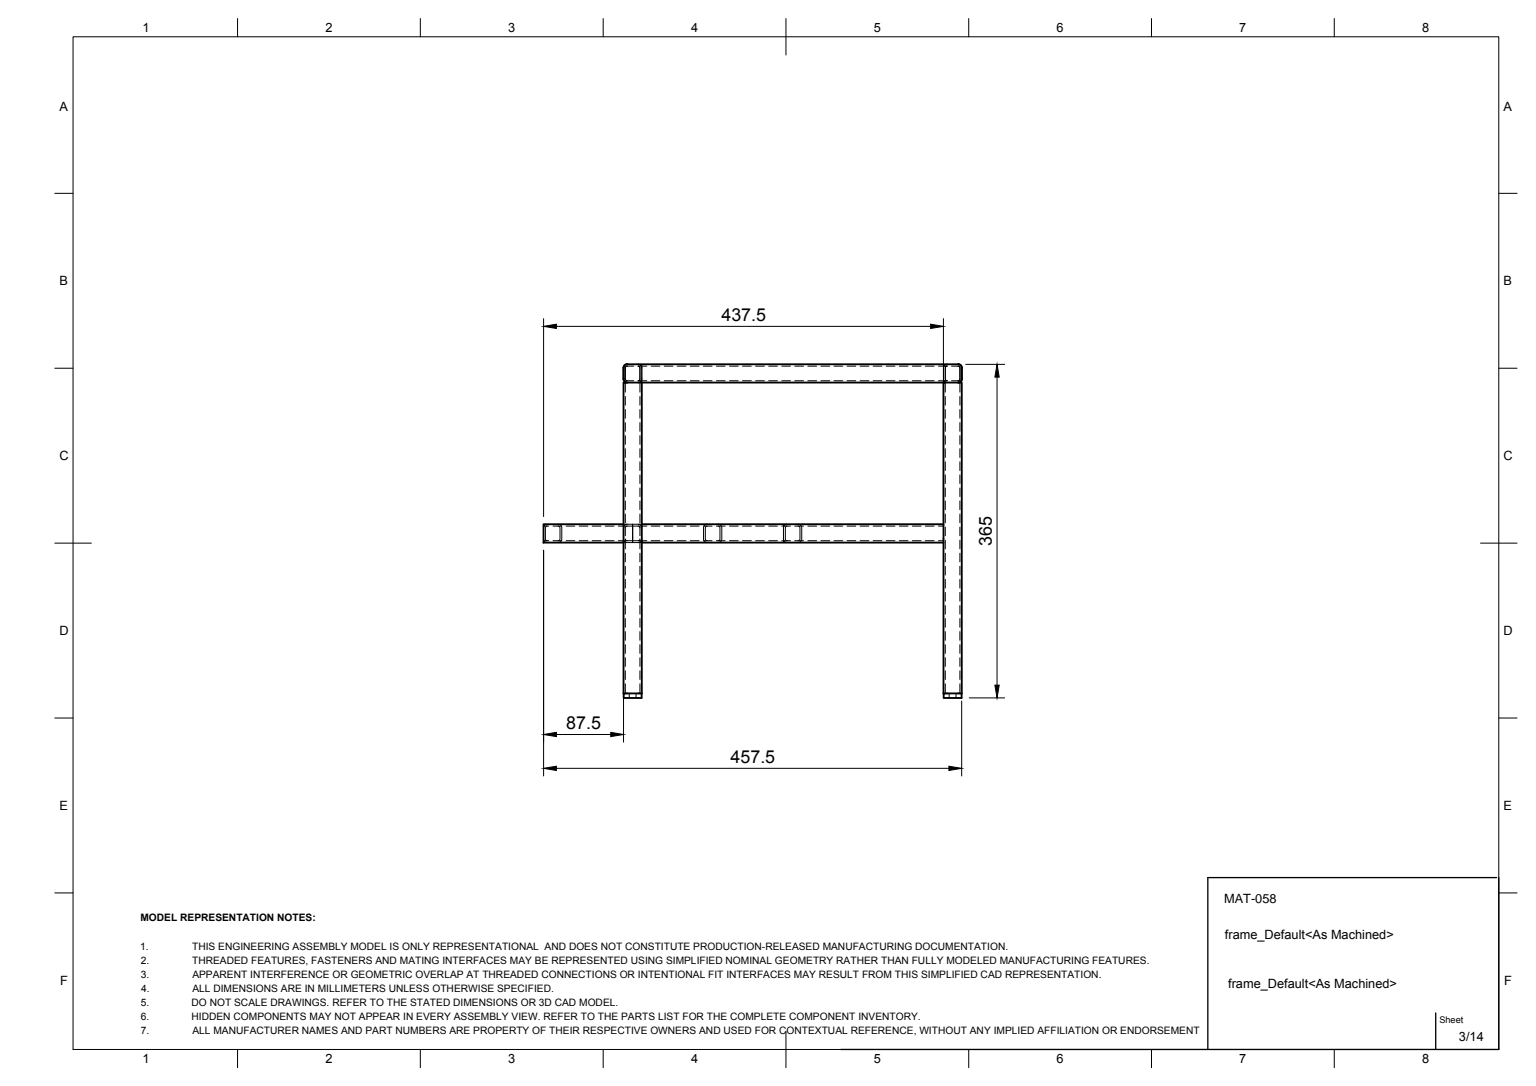
ISO-10303-21;
HEADER;
FILE_DESCRIPTION (('STEP AP214'),
    '1' );
FILE_NAME ('frame_Default<As Machined>.step',
    '2026-10-21T17:54:40',
    ( '' ),
    ( '' ),
    'SwSTEP 2.0',
    'SolidWorks 2026',
    '' );
FILE_SCHEMA (( 'AUTOMOTIVE_DESIGN' ));
ENDSEC;

DATA;
#2=CIRCLE ( 'NONE', #7396, 2.000000000000001776 ) ;
#8=CARTESIAN_POINT ( 'NONE',  ( 341.9999999999999432, -181.0000000000001421, -349.9999999999998863 ) ) ;
#10=ORIENTED_EDGE ( 'NONE', *, *, #50701, .F. ) ;
#13=EDGE_CURVE ( 'NONE', #17667, #14780, #49006, .T. ) ;
#24=AXIS2_PLACEMENT_3D ( 'NONE', #27397, #19697, #35376 ) ;
#26=AXIS2_PLACEMENT_3D ( 'NONE', #26313, #42956, #39141 ) ;
#27=VECTOR ( 'NONE', #2447, 1000.000000000000000 ) ;
#28=EDGE_LOOP ( 'NONE', ( #27721, #41383, #11208, #21958 ) ) ;
#31=ORIENTED_EDGE ( 'NONE', *, *, #39072, .F. ) ;
#35=CARTESIAN_POINT ( 'NONE',  ( 181.0000000000000284, -174.9999999999999716, -111.0000000000001563 ) ) ;
#40=VECTOR ( 'NONE', #48975, 1000.000000000000000 ) ;
#52=( LENGTH_UNIT ( ) NAMED_UNIT ( * ) SI_UNIT ( .MILLI., .METRE. ) );
#53=DIRECTION ( 'NONE',  ( -1.000000000000000000, -0.000000000000000000, -0.000000000000000000 ) ) ;
#55=VERTEX_POINT ( 'NONE', #2115 ) ;
#59=CARTESIAN_POINT ( 'NONE',  ( 164.9999999999999716, -174.9999999999999716, -340.0000000000001137 ) ) ;
#62=AXIS2_PLACEMENT_3D ( 'NONE', #28771, #36489, #21066 ) ;
#68=CARTESIAN_POINT ( 'NONE',  ( 183.0000000000000000, 175.0000000000000284, -356.0000000000001705 ) ) ;
#70=AXIS2_PLACEMENT_3D ( 'NONE', #6927, #30792, #6416 ) ;
#79=DIRECTION ( 'NONE',  ( 0.000000000000000000, -1.000000000000000000, -3.186989995019654210E-49 ) ) ;
#83=ORIENTED_EDGE ( 'NONE', *, *, #42278, .F. ) ;
#87=CARTESIAN_POINT ( 'NONE',  ( 355.9999999999999432, -181.0000000000001421, -349.9999999999999432 ) ) ;
#88=DIRECTION ( 'NONE',  ( 1.121065046350011585E-16, 0.7071067811865475727, 0.7071067811865474617 ) ) ;
#91=ORIENTED_EDGE ( 'NONE', *, *, #48428, .F. ) ;
#96=CIRCLE ( 'NONE', #3362, 4.000000000000003553 ) ;
#98=AXIS2_PLACEMENT_3D ( 'NONE', #41759, #33325, #22512 ) ;
#100=EDGE_LOOP ( 'NONE', ( #22322, #8541, #32792, #19627 ) ) ;
#101=ORIENTED_EDGE ( 'NONE', *, *, #35031, .T. ) ;
#103=FACE_OUTER_BOUND ( 'NONE', #47648, .T. ) ;
#105=ORIENTED_EDGE ( 'NONE', *, *, #23023, .F. ) ;
#111=DIRECTION ( 'NONE',  ( 0.000000000000000000, -2.265761274745217480E-16, 1.000000000000000000 ) ) ;
#114=CARTESIAN_POINT ( 'NONE',  ( 0.000000000000000000, 181.0000000000000284, -356.0000000000002274 ) ) ;
#116=PLANE ( 'NONE',  #46273 ) ;
#117=CARTESIAN_POINT ( 'NONE',  ( 357.1715728752538439, -167.0000000000001137, 342.0000000000000000 ) ) ;
#118=LINE ( 'NONE', #878, #10886 ) ;
#126=CARTESIAN_POINT ( 'NONE',  ( 168.9999999999999716, -272.4999999999999432, -359.9999999999999432 ) ) ;
#127=ORIENTED_EDGE ( 'NONE', *, *, #28456, .T. ) ;
#128=CARTESIAN_POINT ( 'NONE',  ( 355.9999999999999432, 174.9999999999996589, -356.0000000000003411 ) ) ;
#129=CIRCLE ( 'NONE', #5860, 4.000000000000003553 ) ;
#135=EDGE_CURVE ( 'NONE', #16306, #8464, #38459, .T. ) ;
#141=ORIENTED_EDGE ( 'NONE', *, *, #37641, .T. ) ;
#151=ORIENTED_EDGE ( 'NONE', *, *, #46263, .F. ) ;
#152=ORIENTED_EDGE ( 'NONE', *, *, #12710, .F. ) ;
#153=ORIENTED_EDGE ( 'NONE', *, *, #11070, .T. ) ;
#167=EDGE_CURVE ( 'NONE', #5103, #46968, #26727, .T. ) ;
#176=EDGE_CURVE ( 'NONE', #39875, #24207, #43623, .T. ) ;
#177=VECTOR ( 'NONE', #3121, 1000.000000000000000 ) ;
#181=CYLINDRICAL_SURFACE ( 'NONE', #33279, 4.000000000000003553 ) ;
#185=CARTESIAN_POINT ( 'NONE',  ( 359.9999999999999432, -165.0000000000001137, -106.0000000000001990 ) ) ;
#189=EDGE_CURVE ( 'NONE', #37243, #19301, #48193, .T. ) ;
#195=FACE_OUTER_BOUND ( 'NONE', #5721, .T. ) ;
#203=CARTESIAN_POINT ( 'NONE',  ( 349.9999999999999432, -168.9999999999999432, 339.9999999999997726 ) ) ;
#204=ORIENTED_EDGE ( 'NONE', *, *, #887, .F. ) ;
#208=ORIENTED_EDGE ( 'NONE', *, *, #13614, .F. ) ;
#210=CARTESIAN_POINT ( 'NONE',  ( 168.9999999999999716, 165.0000000000000000, -360.0000000000002274 ) ) ;
#211=DIRECTION ( 'NONE',  ( -1.000000000000000000, 0.000000000000000000, 1.860490536778032451E-50 ) ) ;
#212=ADVANCED_FACE ( 'NONE', ( #47688 ), #43368, .T. ) ;
#215=DIRECTION ( 'NONE',  ( 0.000000000000000000, 3.186989995019654210E-49, 1.000000000000000000 ) ) ;
#216=DIRECTION ( 'NONE',  ( 3.172065784643302499E-16, 1.000000000000000000, 0.000000000000000000 ) ) ;
#218=VERTEX_POINT ( 'NONE', #20031 ) ;
#220=CARTESIAN_POINT ( 'NONE',  ( 168.9999999999999716, 10.00000000000006395, 339.9999999999998295 ) ) ;
#223=EDGE_LOOP ( 'NONE', ( #625, #40155, #13058, #17108 ) ) ;
#236=DIRECTION ( 'NONE',  ( -0.000000000000000000, -1.000000000000000000, 2.537652627714643577E-15 ) ) ;
#250=AXIS2_PLACEMENT_3D ( 'NONE', #2774, #2274, #17912 ) ;
#254=DIRECTION ( 'NONE',  ( 0.000000000000000000, -1.000000000000000000, 0.000000000000000000 ) ) ;
#260=ORIENTED_EDGE ( 'NONE', *, *, #20042, .T. ) ;
#262=ORIENTED_EDGE ( 'NONE', *, *, #31509, .T. ) ;
#269=VERTEX_POINT ( 'NONE', #28497 ) ;
#274=ORIENTED_EDGE ( 'NONE', *, *, #2719, .F. ) ;
#276=CARTESIAN_POINT ( 'NONE',  ( 358.0000000000000000, -165.0000000000001137, -94.00000000000019895 ) ) ;
#278=DIRECTION ( 'NONE',  ( 0.000000000000000000, 5.664403186863042467E-17, 1.000000000000000000 ) ) ;
#280=DIRECTION ( 'NONE',  ( 3.172065784643304472E-16, 1.000000000000000000, -1.710569414459005214E-49 ) ) ;
#281=EDGE_CURVE ( 'NONE', #25566, #31089, #9489, .T. ) ;
#286=EDGE_LOOP ( 'NONE', ( #4759, #15600, #2107, #33444, #6619, #35466, #25872, #11433 ) ) ;
#291=CARTESIAN_POINT ( 'NONE',  ( 356.0000000000000000, -167.0000000000001137, -349.9999999999999432 ) ) ;
#292=FACE_OUTER_BOUND ( 'NONE', #17808, .T. ) ;
#296=EDGE_CURVE ( 'NONE', #47828, #22723, #5634, .T. ) ;
#301=DIRECTION ( 'NONE',  ( 0.000000000000000000, 0.000000000000000000, -1.000000000000000000 ) ) ;
#303=ORIENTED_EDGE ( 'NONE', *, *, #21142, .F. ) ;
#304=EDGE_CURVE ( 'NONE', #27971, #25755, #44964, .T. ) ;
#310=CIRCLE ( 'NONE', #31701, 4.000000000000003553 ) ;
#315=CARTESIAN_POINT ( 'NONE',  ( 339.9999999999998863, -183.3431457505075741, 358.3431457505074036 ) ) ;
#318=PLANE ( 'NONE',  #3677 ) ;
#324=CARTESIAN_POINT ( 'NONE',  ( 340.0000000000000000, 181.0000000000000568, 359.9999999999998295 ) ) ;
#328=CARTESIAN_POINT ( 'NONE',  ( 340.0000000000000568, 185.0000000000000284, 355.9999999999997726 ) ) ;
#330=ORIENTED_EDGE ( 'NONE', *, *, #46512, .T. ) ;
#333=CARTESIAN_POINT ( 'NONE',  ( 355.9999999999999432, 185.0000000000002274, -360.0000000000003411 ) ) ;
#336=LINE ( 'NONE', #31644, #47492 ) ;
#340=ORIENTED_EDGE ( 'NONE', *, *, #875, .T. ) ;
#345=DIRECTION ( 'NONE',  ( -1.000000000000000000, 0.000000000000000000, 0.000000000000000000 ) ) ;
#347=VECTOR ( 'NONE', #5302, 1000.000000000000000 ) ;
#351=AXIS2_PLACEMENT_3D ( 'NONE', #22254, #34073, #6858 ) ;
#353=DIRECTION ( 'NONE',  ( 0.000000000000000000, 0.000000000000000000, 1.000000000000000000 ) ) ;
#354=VECTOR ( 'NONE', #29219, 1000.000000000000000 ) ;
#355=DIRECTION ( 'NONE',  ( 3.172065745548403743E-16, 1.000000000000000000, 0.000000000000000000 ) ) ;
#359=EDGE_LOOP ( 'NONE', ( #2759, #29859, #45477, #2453, #26930, #35930, #303, #44900 ) ) ;
#363=ORIENTED_EDGE ( 'NONE', *, *, #44882, .T. ) ;
#370=CARTESIAN_POINT ( 'NONE',  ( 356.0000000000000000, 175.0000000000000284, -108.0000000000002132 ) ) ;
#372=CARTESIAN_POINT ( 'NONE',  ( 185.0000000000000000, -93.49999999999998579, -350.0000000000001705 ) ) ;
#373=LINE ( 'NONE', #27571, #20702 ) ;
#376=EDGE_CURVE ( 'NONE', #35109, #22226, #31907, .T. ) ;
#380=CARTESIAN_POINT ( 'NONE',  ( 0.000000000000000000, -165.1999999999999602, 340.1999999999997044 ) ) ;
#390=DIRECTION ( 'NONE',  ( 0.000000000000000000, -2.265761274745217480E-16, 1.000000000000000000 ) ) ;
#399=CARTESIAN_POINT ( 'NONE',  ( 343.9999999999999432, 174.9999999999996589, -360.0000000000003411 ) ) ;
#401=CYLINDRICAL_SURFACE ( 'NONE', #39045, 4.000000000000003553 ) ;
#402=DIRECTION ( 'NONE',  ( 1.000000000000000000, -4.105366553918459587E-48, -1.586032880504786307E-16 ) ) ;
#416=CARTESIAN_POINT ( 'NONE',  ( 344.0000000000000000, 165.0000000000000000, -90.00000000000018474 ) ) ;
#417=ORIENTED_EDGE ( 'NONE', *, *, #25940, .F. ) ;
#424=LINE ( 'NONE', #28123, #46558 ) ;
#427=EDGE_CURVE ( 'NONE', #32721, #15345, #25659, .T. ) ;
#428=PLANE ( 'NONE',  #26708 ) ;
#432=DIRECTION ( 'NONE',  ( -1.000000000000000000, 1.331116318405244905E-23, 4.755310728521421461E-16 ) ) ;
#433=ADVANCED_FACE ( 'NONE', ( #33614 ), #49204, .F. ) ;
#435=APPLICATION_CONTEXT ( 'automotive_design' ) ;
#439=DIRECTION ( 'NONE',  ( -1.586032892321652236E-16, -1.000000000000000000, -6.853681917100419162E-49 ) ) ;
#441=ORIENTED_EDGE ( 'NONE', *, *, #33733, .F. ) ;
#445=CIRCLE ( 'NONE', #40629, 2.000000000000001776 ) ;
#462=LINE ( 'NONE', #35873, #24910 ) ;
#471=ORIENTED_EDGE ( 'NONE', *, *, #17428, .F. ) ;
#473=CARTESIAN_POINT ( 'NONE',  ( 355.9999999999999432, -185.0000000000001421, 360.0000000000000000 ) ) ;
#474=ORIENTED_EDGE ( 'NONE', *, *, #34538, .F. ) ;
#476=ORIENTED_EDGE ( 'NONE', *, *, #29069, .T. ) ;
#479=AXIS2_PLACEMENT_3D ( 'NONE', #48205, #1053, #44377 ) ;
#481=ORIENTED_EDGE ( 'NONE', *, *, #5333, .T. ) ;
#489=EDGE_CURVE ( 'NONE', #13008, #49667, #30971, .T. ) ;
#492=DIRECTION ( 'NONE',  ( 1.000000000000000000, 0.000000000000000000, 0.000000000000000000 ) ) ;
#495=DIRECTION ( 'NONE',  ( 0.000000000000000000, 2.537652627714642000E-15, 1.000000000000000000 ) ) ;
#497=AXIS2_PLACEMENT_3D ( 'NONE', #34833, #26856, #31230 ) ;
#498=EDGE_CURVE ( 'NONE', #19922, #10844, #20629, .T. ) ;
#500=PLANE ( 'NONE',  #17515 ) ;
#501=CARTESIAN_POINT ( 'NONE',  ( 359.9999999999999432, -181.0000000000001137, -356.0000000000003411 ) ) ;
#504=CARTESIAN_POINT ( 'NONE',  ( 343.9999999999999432, 165.0000000000000000, -108.0000000000002132 ) ) ;
#505=ORIENTED_EDGE ( 'NONE', *, *, #34410, .F. ) ;
#513=LINE ( 'NONE', #24116, #49110 ) ;
#514=EDGE_CURVE ( 'NONE', #45973, #15209, #36212, .T. ) ;
#524=CIRCLE ( 'NONE', #29193, 2.000000000000001776 ) ;
#537=CARTESIAN_POINT ( 'NONE',  ( 168.9999999999999716, 10.00000000000006395, -350.0000000000001705 ) ) ;
#541=VERTEX_POINT ( 'NONE', #28876 ) ;
#545=DIRECTION ( 'NONE',  ( 0.000000000000000000, 0.000000000000000000, -1.000000000000000000 ) ) ;
#551=DIRECTION ( 'NONE',  ( 1.000000000000000000, -4.758098676964956461E-16, -8.975803739141899931E-48 ) ) ;
#557=CARTESIAN_POINT ( 'NONE',  ( 181.0000000000000000, -182.9999999999999716, -350.0000000000001705 ) ) ;
#558=PLANE ( 'NONE',  #37929 ) ;
#564=CARTESIAN_POINT ( 'NONE',  ( 339.9999999999999432, -168.9999999999999432, 343.9999999999998295 ) ) ;
#584=VECTOR ( 'NONE', #25385, 1000.000000000000000 ) ;
#586=VERTEX_POINT ( 'NONE', #1185 ) ;
#590=DIRECTION ( 'NONE',  ( 0.000000000000000000, 0.000000000000000000, -1.000000000000000000 ) ) ;
#605=FACE_OUTER_BOUND ( 'NONE', #3161, .T. ) ;
#606=DIRECTION ( 'NONE',  ( 3.172065745548403743E-16, 1.000000000000000000, 0.000000000000000000 ) ) ;
#607=ORIENTED_EDGE ( 'NONE', *, *, #46352, .F. ) ;
#618=ORIENTED_EDGE ( 'NONE', *, *, #16431, .T. ) ;
#619=CARTESIAN_POINT ( 'NONE',  ( 350.0000000000000000, -164.9999999999999432, -344.0000000000001705 ) ) ;
#621=DIRECTION ( 'NONE',  ( 0.000000000000000000, 0.000000000000000000, -1.000000000000000000 ) ) ;
#625=ORIENTED_EDGE ( 'NONE', *, *, #32485, .F. ) ;
#626=ORIENTED_EDGE ( 'NONE', *, *, #37900, .T. ) ;
#627=DIRECTION ( 'NONE',  ( -0.000000000000000000, 0.000000000000000000, 1.000000000000000000 ) ) ;
#631=DIRECTION ( 'NONE',  ( 0.000000000000000000, -1.000000000000000000, 5.664403186863042467E-17 ) ) ;
#637=DIRECTION ( 'NONE',  ( 0.000000000000000000, 2.537652627714642000E-15, 1.000000000000000000 ) ) ;
#640=ORIENTED_EDGE ( 'NONE', *, *, #27418, .F. ) ;
#644=ORIENTED_EDGE ( 'NONE', *, *, #10302, .T. ) ;
#647=DIRECTION ( 'NONE',  ( 1.000000000000000000, 0.000000000000000000, 0.000000000000000000 ) ) ;
#660=LINE ( 'NONE', #35837, #18061 ) ;
#664=ORIENTED_EDGE ( 'NONE', *, *, #22451, .F. ) ;
#665=ORIENTED_EDGE ( 'NONE', *, *, #13294, .F. ) ;
#673=EDGE_LOOP ( 'NONE', ( #3363, #25492, #26505, #29647 ) ) ;
#677=EDGE_CURVE ( 'NONE', #7451, #29467, #310, .T. ) ;
#695=EDGE_LOOP ( 'NONE', ( #33411, #25754, #20493, #618 ) ) ;
#697=DIRECTION ( 'NONE',  ( -1.000000000000000000, 0.000000000000000000, 0.000000000000000000 ) ) ;
#701=LINE ( 'NONE', #27656, #40511 ) ;
#710=ORIENTED_EDGE ( 'NONE', *, *, #4911, .F. ) ;
#711=AXIS2_PLACEMENT_3D ( 'NONE', #49529, #33197, #17779 ) ;
#716=ORIENTED_EDGE ( 'NONE', *, *, #36986, .T. ) ;
#722=CLOSED_SHELL ( 'NONE', ( #33273, #13699, #32863, #47477, #42616, #48990, #26917, #42906, #40350, #7482, #18343, #10767, #37802, #12006, #35923, #10315, #35706, #47951 ) ) ;
#723=EDGE_CURVE ( 'NONE', #541, #5037, #49825, .T. ) ;
#724=DIRECTION ( 'NONE',  ( 0.000000000000000000, 1.000000000000000000, 0.000000000000000000 ) ) ;
#727=DIRECTION ( 'NONE',  ( 0.000000000000000000, 0.000000000000000000, 1.000000000000000000 ) ) ;
#728=PLANE ( 'NONE',  #43991 ) ;
#737=EDGE_CURVE ( 'NONE', #25893, #7888, #18657, .T. ) ;
#742=DIRECTION ( 'NONE',  ( 1.000000000000000000, 0.000000000000000000, 0.000000000000000000 ) ) ;
#750=VERTEX_POINT ( 'NONE', #17821 ) ;
#753=VECTOR ( 'NONE', #3880, 1000.000000000000000 ) ;
#754=ORIENTED_EDGE ( 'NONE', *, *, #25734, .F. ) ;
#761=CARTESIAN_POINT ( 'NONE',  ( 344.0000000000000568, -165.0000000000001137, 340.0000000000000568 ) ) ;
#767=EDGE_CURVE ( 'NONE', #14253, #48821, #16231, .T. ) ;
#770=DIRECTION ( 'NONE',  ( 0.000000000000000000, 0.000000000000000000, -1.000000000000000000 ) ) ;
#771=ORIENTED_EDGE ( 'NONE', *, *, #33152, .T. ) ;
#773=CARTESIAN_POINT ( 'NONE',  ( 350.0000000000000000, -164.9999999999999432, 339.9999999999997726 ) ) ;
#775=CARTESIAN_POINT ( 'NONE',  ( 181.0000000000000000, -93.49999999999998579, -350.0000000000001705 ) ) ;
#779=PLANE ( 'NONE',  #43621 ) ;
#780=ORIENTED_EDGE ( 'NONE', *, *, #22663, .T. ) ;
#782=ORIENTED_EDGE ( 'NONE', *, *, #44110, .F. ) ;
#786=DIRECTION ( 'NONE',  ( 4.996003610813203446E-16, 1.000000000000000000, 0.000000000000000000 ) ) ;
#790=FACE_OUTER_BOUND ( 'NONE', #30397, .T. ) ;
#792=EDGE_LOOP ( 'NONE', ( #16265, #22967, #43892, #43654, #12939, #41162, #11499, #30707 ) ) ;
#795=DIRECTION ( 'NONE',  ( -1.586032892321652236E-16, -1.000000000000000000, -6.853681917100419162E-49 ) ) ;
#804=VECTOR ( 'NONE', #10594, 1000.000000000000000 ) ;
#805=FACE_OUTER_BOUND ( 'NONE', #27242, .T. ) ;
#808=EDGE_CURVE ( 'NONE', #7132, #20673, #30143, .T. ) ;
#812=ORIENTED_EDGE ( 'NONE', *, *, #6128, .T. ) ;
#813=EDGE_CURVE ( 'NONE', #46472, #47613, #15528, .T. ) ;
#816=CARTESIAN_POINT ( 'NONE',  ( 340.0000000000000000, 165.0000000000000000, -94.00000000000019895 ) ) ;
#825=DIRECTION ( 'NONE',  ( 0.000000000000000000, 3.186989995019654210E-49, 1.000000000000000000 ) ) ;
#827=DIRECTION ( 'NONE',  ( 1.000000000000000000, -4.996003610813203446E-16, 1.033975765691284410E-24 ) ) ;
#828=AXIS2_PLACEMENT_3D ( 'NONE', #16656, #16407, #1278 ) ;
#831=VECTOR ( 'NONE', #20626, 1000.000000000000000 ) ;
#843=ORIENTED_EDGE ( 'NONE', *, *, #48550, .T. ) ;
#846=ORIENTED_EDGE ( 'NONE', *, *, #17978, .T. ) ;
#847=DIRECTION ( 'NONE',  ( 0.000000000000000000, 0.000000000000000000, -1.000000000000000000 ) ) ;
#849=CARTESIAN_POINT ( 'NONE',  ( 181.0000000000000000, 165.0000000000000000, -356.0000000000001705 ) ) ;
#850=ORIENTED_EDGE ( 'NONE', *, *, #26302, .T. ) ;
#853=CARTESIAN_POINT ( 'NONE',  ( 341.9999999999999432, -174.9999999999999432, 343.9999999999998295 ) ) ;
#859=ORIENTED_EDGE ( 'NONE', *, *, #37775, .T. ) ;
#870=CARTESIAN_POINT ( 'NONE',  ( 360.0000000000000000, 169.0000000000000000, -344.0000000000001705 ) ) ;
#873=EDGE_CURVE ( 'NONE', #23733, #17617, #46498, .T. ) ;
#874=AXIS2_PLACEMENT_3D ( 'NONE', #50548, #11862, #46963 ) ;
#875=EDGE_CURVE ( 'NONE', #3991, #24185, #15745, .T. ) ;
#878=CARTESIAN_POINT ( 'NONE',  ( 350.0000000000001137, 165.0000000000000000, 339.9999999999997726 ) ) ;
#879=ORIENTED_EDGE ( 'NONE', *, *, #10874, .F. ) ;
#881=VECTOR ( 'NONE', #25390, 1000.000000000000000 ) ;
#887=EDGE_CURVE ( 'NONE', #25778, #16503, #8068, .T. ) ;
#888=ADVANCED_FACE ( 'NONE', ( #35027, #43446 ), #35271, .F. ) ;
#890=CARTESIAN_POINT ( 'NONE',  ( 356.0000000000000000, 175.0000000000000284, -106.0000000000001990 ) ) ;
#891=VERTEX_POINT ( 'NONE', #8318 ) ;
#899=DIRECTION ( 'NONE',  ( -1.000000000000000000, 0.000000000000000000, -2.958228394578794270E-31 ) ) ;
#901=EDGE_LOOP ( 'NONE', ( #812, #8607, #36597, #25658, #49808, #20531, #25126, #10877 ) ) ;
#905=AXIS2_PLACEMENT_3D ( 'NONE', #21960, #14251, #29911 ) ;
#912=CARTESIAN_POINT ( 'NONE',  ( 358.0000000000000000, 181.0000000000000284, -356.0000000000001705 ) ) ;
#913=VERTEX_POINT ( 'NONE', #3428 ) ;
#917=ADVANCED_FACE ( 'NONE', ( #47265 ), #4455, .F. ) ;
#921=VERTEX_POINT ( 'NONE', #15493 ) ;
#922=CARTESIAN_POINT ( 'NONE',  ( 166.9999999999999716, -81.49999999999997158, -350.0000000000001705 ) ) ;
#933=EDGE_CURVE ( 'NONE', #12765, #28712, #42680, .T. ) ;
#943=EDGE_CURVE ( 'NONE', #29362, #4473, #21108, .T. ) ;
#945=LINE ( 'NONE', #44015, #12242 ) ;
#946=VECTOR ( 'NONE', #12223, 1000.000000000000000 ) ;
#948=CIRCLE ( 'NONE', #42702, 4.000000000000003553 ) ;
#951=( LENGTH_UNIT ( ) NAMED_UNIT ( * ) SI_UNIT ( .MILLI., .METRE. ) );
#958=FACE_OUTER_BOUND ( 'NONE', #48495, .T. ) ;
#964=DIRECTION ( 'NONE',  ( -1.586032880504786307E-16, 1.654361225106055350E-24, -1.000000000000000000 ) ) ;
#974=ORIENTED_EDGE ( 'NONE', *, *, #47561, .T. ) ;
#976=VECTOR ( 'NONE', #24664, 1000.000000000000000 ) ;
#980=VERTEX_POINT ( 'NONE', #870 ) ;
#994=FACE_BOUND ( 'NONE', #1999, .T. ) ;
#996=UNCERTAINTY_MEASURE_WITH_UNIT (LENGTH_MEASURE( 1.000000000000000082E-05 ), #25917, 'distance_accuracy_value', 'NONE');
#1002=AXIS2_PLACEMENT_3D ( 'NONE', #43365, #551, #47189 ) ;
#1006=AXIS2_PLACEMENT_3D ( 'NONE', #10575, #7241, #26244 ) ;
#1007=ORIENTED_EDGE ( 'NONE', *, *, #6239, .F. ) ;
#1009=AXIS2_PLACEMENT_3D ( 'NONE', #24502, #44226, #9104 ) ;
#1011=ORIENTED_EDGE ( 'NONE', *, *, #33096, .F. ) ;
#1013=CARTESIAN_POINT ( 'NONE',  ( 169.0000000000000000, -174.9999999999999716, -111.0000000000001563 ) ) ;
#1018=ORIENTED_EDGE ( 'NONE', *, *, #28826, .T. ) ;
#1025=DIRECTION ( 'NONE',  ( 2.874857526315640942E-31, -1.000000000000000000, 2.537652627714643577E-15 ) ) ;
#1026=AXIS2_PLACEMENT_3D ( 'NONE', #8099, #23744, #11682 ) ;
#1033=VECTOR ( 'NONE', #47820, 1000.000000000000000 ) ;
#1042=LINE ( 'NONE', #5128, #26252 ) ;
#1043=DIRECTION ( 'NONE',  ( -1.000000000000000000, 1.331116318405244905E-23, 4.759647537211363479E-16 ) ) ;
#1044=AXIS2_PLACEMENT_3D ( 'NONE', #45099, #28976, #17429 ) ;
#1045=VERTEX_POINT ( 'NONE', #32667 ) ;
#1047=PLANE ( 'NONE',  #45564 ) ;
#1053=DIRECTION ( 'NONE',  ( 0.000000000000000000, -2.537652627714643577E-15, -1.000000000000000000 ) ) ;
#1056=CARTESIAN_POINT ( 'NONE',  ( 183.0000000000000000, -164.9999999999999432, -344.0000000000001137 ) ) ;
#1063=PLANE ( 'NONE',  #31580 ) ;
#1064=EDGE_CURVE ( 'NONE', #18038, #23733, #24471, .T. ) ;
#1065=CARTESIAN_POINT ( 'NONE',  ( 0.000000000000000000, -184.9999999999999716, -344.0000000000001705 ) ) ;
#1076=DIRECTION ( 'NONE',  ( -4.996003610813203446E-16, -1.000000000000000000, 0.000000000000000000 ) ) ;
#1079=DIRECTION ( 'NONE',  ( -1.000000000000000000, 0.000000000000000000, -2.958228394578794270E-31 ) ) ;
#1080=VECTOR ( 'NONE', #22199, 1000.000000000000000 ) ;
#1084=LINE ( 'NONE', #28024, #34432 ) ;
#1088=ORIENTED_EDGE ( 'NONE', *, *, #677, .F. ) ;
#1102=EDGE_CURVE ( 'NONE', #9708, #15072, #33683, .T. ) ;
#1107=VERTEX_POINT ( 'NONE', #14152 ) ;
#1109=CIRCLE ( 'NONE', #39605, 4.000000000000003553 ) ;
#1115=VERTEX_POINT ( 'NONE', #45936 ) ;
#1122=CARTESIAN_POINT ( 'NONE',  ( 350.0000000000000000, -166.9999999999999432, -356.0000000000002274 ) ) ;
#1123=DIRECTION ( 'NONE',  ( -1.000000000000000000, 0.000000000000000000, 1.860490536778032451E-50 ) ) ;
#1124=DIRECTION ( 'NONE',  ( -1.860490536778032451E-50, 0.000000000000000000, 1.000000000000000000 ) ) ;
#1127=AXIS2_PLACEMENT_3D ( 'NONE', #37314, #21123, #10080 ) ;
#1132=CARTESIAN_POINT ( 'NONE',  ( 183.0000000000000000, -5.999999999999950262, -350.0000000000001705 ) ) ;
#1136=VECTOR ( 'NONE', #49570, 1000.000000000000000 ) ;
#1138=EDGE_LOOP ( 'NONE', ( #3171, #13323, #12762, #33669 ) ) ;
#1140=ORIENTED_EDGE ( 'NONE', *, *, #36191, .F. ) ;
#1146=CARTESIAN_POINT ( 'NONE',  ( 344.0000000000000000, 165.0000000000000000, -340.0000000000001137 ) ) ;
#1151=ORIENTED_EDGE ( 'NONE', *, *, #23396, .F. ) ;
#1163=LINE ( 'NONE', #28851, #47055 ) ;
#1166=ORIENTED_EDGE ( 'NONE', *, *, #19540, .F. ) ;
#1171=EDGE_CURVE ( 'NONE', #24437, #48718, #17769, .T. ) ;
#1175=FACE_OUTER_BOUND ( 'NONE', #4354, .T. ) ;
#1177=VERTEX_POINT ( 'NONE', #50018 ) ;
#1185=CARTESIAN_POINT ( 'NONE',  ( 168.9999999999999716, 165.0000000000000000, -342.0000000000001137 ) ) ;
#1187=DIRECTION ( 'NONE',  ( 0.000000000000000000, -1.000000000000000000, 3.186989995019654210E-49 ) ) ;
#1190=DIRECTION ( 'NONE',  ( 0.000000000000000000, -1.000000000000000000, 2.537652627714643577E-15 ) ) ;
#1191=ORIENTED_EDGE ( 'NONE', *, *, #21634, .T. ) ;
#1194=DIRECTION ( 'NONE',  ( 0.000000000000000000, 0.000000000000000000, 1.000000000000000000 ) ) ;
#1196=AXIS2_PLACEMENT_3D ( 'NONE', #1796, #2048, #11002 ) ;
#1203=ORIENTED_EDGE ( 'NONE', *, *, #7025, .F. ) ;
#1206=AXIS2_PLACEMENT_3D ( 'NONE', #1940, #6300, #16138 ) ;
#1207=VERTEX_POINT ( 'NONE', #42867 ) ;
#1210=CARTESIAN_POINT ( 'NONE',  ( 343.9999999999999432, 183.0000000000002274, -358.0000000000003411 ) ) ;
#1218=EDGE_CURVE ( 'NONE', #14253, #1522, #27244, .T. ) ;
#1225=EDGE_CURVE ( 'NONE', #46658, #3850, #26979, .T. ) ;
#1242=CARTESIAN_POINT ( 'NONE',  ( 5.551115123125782702E-14, -168.9999999999999432, 355.9999999999997726 ) ) ;
#1254=DIRECTION ( 'NONE',  ( 1.586032880504786307E-16, -1.654361225106055350E-24, 1.000000000000000000 ) ) ;
#1255=DIRECTION ( 'NONE',  ( 0.000000000000000000, 0.000000000000000000, 1.000000000000000000 ) ) ;
#1256=AXIS2_PLACEMENT_3D ( 'NONE', #22784, #50179, #26889 ) ;
#1260=LINE ( 'NONE', #5343, #40134 ) ;
#1264=LINE ( 'NONE', #17150, #43490 ) ;
#1271=CARTESIAN_POINT ( 'NONE',  ( 181.0000000000000000, -95.49999999999998579, -340.0000000000001137 ) ) ;
#1273=LINE ( 'NONE', #24619, #10109 ) ;
#1278=DIRECTION ( 'NONE',  ( 0.000000000000000000, 0.000000000000000000, -1.000000000000000000 ) ) ;
#1281=CARTESIAN_POINT ( 'NONE',  ( 339.9999999999999432, -180.9999999999999432, 355.9999999999998295 ) ) ;
#1283=DIRECTION ( 'NONE',  ( -1.586032892321652482E-16, 0.000000000000000000, -1.000000000000000000 ) ) ;
#1290=CARTESIAN_POINT ( 'NONE',  ( 358.0000000000000568, -167.8284271247462982, -342.8284271247463835 ) ) ;
#1300=DIRECTION ( 'NONE',  ( -1.000000000000000000, 0.000000000000000000, 0.000000000000000000 ) ) ;
#1301=DIRECTION ( 'NONE',  ( 0.000000000000000000, 1.000000000000000000, 0.000000000000000000 ) ) ;
#1304=ORIENTED_EDGE ( 'NONE', *, *, #7631, .F. ) ;
#1309=ORIENTED_EDGE ( 'NONE', *, *, #16925, .F. ) ;
#1311=SHAPE_DEFINITION_REPRESENTATION ( #4067, #13952 ) ;
#1312=CARTESIAN_POINT ( 'NONE',  ( -5.000000000000000000, -165.1999999999999602, -340.2000000000001592 ) ) ;
#1315=CARTESIAN_POINT ( 'NONE',  ( 341.9999999999999432, -169.0000000000001705, 344.0000000000000568 ) ) ;
#1316=CIRCLE ( 'NONE', #14411, 2.000000000000001776 ) ;
#1317=DIRECTION ( 'NONE',  ( -1.000000000000000000, 4.996003610813203446E-16, 1.586032878436834529E-16 ) ) ;
#1318=ORIENTED_EDGE ( 'NONE', *, *, #3537, .T. ) ;
#1325=EDGE_CURVE ( 'NONE', #33108, #17487, #26735, .T. ) ;
#1332=LINE ( 'NONE', #2322, #36429 ) ;
#1338=CARTESIAN_POINT ( 'NONE',  ( 168.9999999999999716, -164.9999999999999432, -340.0000000000001705 ) ) ;
#1342=CARTESIAN_POINT ( 'NONE',  ( 168.9999999999999716, -168.9999999999999432, -340.0000000000001137 ) ) ;
#1345=DIRECTION ( 'NONE',  ( 0.000000000000000000, 0.000000000000000000, -1.000000000000000000 ) ) ;
#1351=AXIS2_PLACEMENT_3D ( 'NONE', #46682, #786, #27229 ) ;
#1358=DIRECTION ( 'NONE',  ( -1.000000000000000000, 0.000000000000000000, 0.000000000000000000 ) ) ;
#1361=ORIENTED_EDGE ( 'NONE', *, *, #3520, .F. ) ;
#1363=ORIENTED_EDGE ( 'NONE', *, *, #40965, .F. ) ;
#1368=CARTESIAN_POINT ( 'NONE',  ( 356.0000000000000000, 183.0000000000000284, -358.0000000000002842 ) ) ;
#1371=EDGE_CURVE ( 'NONE', #10844, #33292, #12098, .T. ) ;
#1378=DIRECTION ( 'NONE',  ( -1.612977847700450206E-50, 0.000000000000000000, -1.000000000000000000 ) ) ;
#1382=DIRECTION ( 'NONE',  ( -1.000000000000000000, 0.000000000000000000, -0.000000000000000000 ) ) ;
#1390=AXIS2_PLACEMENT_3D ( 'NONE', #45292, #10176, #42469 ) ;
#1391=ORIENTED_EDGE ( 'NONE', *, *, #49902, .T. ) ;
#1394=CARTESIAN_POINT ( 'NONE',  ( 356.0000000000000568, 185.0000000000001137, 359.9999999999998295 ) ) ;
#1397=LINE ( 'NONE', #5476, #31278 ) ;
#1398=VERTEX_POINT ( 'NONE', #44129 ) ;
#1406=ADVANCED_FACE ( 'NONE', ( #805 ), #5140, .T. ) ;
#1411=ORIENTED_EDGE ( 'NONE', *, *, #17073, .T. ) ;
#1412=ADVANCED_FACE ( 'NONE', ( #40805 ), #8763, .F. ) ;
#1414=LINE ( 'NONE', #32464, #28071 ) ;
#1426=VERTEX_POINT ( 'NONE', #1312 ) ;
#1428=CARTESIAN_POINT ( 'NONE',  ( 360.0000000000000000, 169.0000000000000000, -344.0000000000001705 ) ) ;
#1438=EDGE_CURVE ( 'NONE', #16652, #39156, #48204, .T. ) ;
#1442=CARTESIAN_POINT ( 'NONE',  ( 167.0000000000000000, 2.775557561562891351E-14, -111.0000000000001563 ) ) ;
#1447=ADVANCED_FACE ( 'NONE', ( #43629 ), #8507, .F. ) ;
#1449=LINE ( 'NONE', #40699, #40095 ) ;
#1450=DIRECTION ( 'NONE',  ( 0.000000000000000000, 2.969158215481698263E-48, -1.000000000000000000 ) ) ;
#1454=EDGE_CURVE ( 'NONE', #19947, #30540, #41558, .T. ) ;
#1469=ORIENTED_EDGE ( 'NONE', *, *, #25027, .T. ) ;
#1472=FACE_OUTER_BOUND ( 'NONE', #12433, .T. ) ;
#1484=ORIENTED_EDGE ( 'NONE', *, *, #39994, .T. ) ;
#1488=LINE ( 'NONE', #1981, #6990 ) ;
#1489=EDGE_LOOP ( 'NONE', ( #35101, #41501, #18818, #26566 ) ) ;
#1490=CARTESIAN_POINT ( 'NONE',  ( 181.0000000000000284, -174.9999999999999716, -95.00000000000014211 ) ) ;
#1493=DIRECTION ( 'NONE',  ( 0.000000000000000000, 0.7071067811865475727, 0.7071067811865474617 ) ) ;
#1508=DIRECTION ( 'NONE',  ( 0.000000000000000000, -1.000000000000000000, 0.000000000000000000 ) ) ;
#1511=ADVANCED_FACE ( 'NONE', ( #37485 ), #21549, .F. ) ;
#1515=VERTEX_POINT ( 'NONE', #49713 ) ;
#1516=CARTESIAN_POINT ( 'NONE',  ( 340.0000000000000000, 2.999999999999780176, -172.0000000000003126 ) ) ;
#1518=LINE ( 'NONE', #31819, #42378 ) ;
#1522=VERTEX_POINT ( 'NONE', #29757 ) ;
#1531=LINE ( 'NONE', #48673, #24115 ) ;
#1534=CLOSED_SHELL ( 'NONE', ( #35763, #10524, #38050, #13677, #45020, #8977, #29636, #25368 ) ) ;
#1540=ORIENTED_EDGE ( 'NONE', *, *, #24099, .F. ) ;
#1544=CARTESIAN_POINT ( 'NONE',  ( 168.9999999999999716, -77.49999999999997158, -350.0000000000001705 ) ) ;
#1552=CARTESIAN_POINT ( 'NONE',  ( 185.0000000000000568, 175.0000000000000284, 343.9999999999998863 ) ) ;
#1554=LINE ( 'NONE', #40548, #3495 ) ;
#1557=VECTOR ( 'NONE', #22431, 1000.000000000000000 ) ;
#1563=CARTESIAN_POINT ( 'NONE',  ( 166.9999999999999716, -81.49999999999988631, -115.0000000000001563 ) ) ;
#1569=VECTOR ( 'NONE', #37477, 1000.000000000000000 ) ;
#1575=CARTESIAN_POINT ( 'NONE',  ( 0.000000000000000000, 184.8000000000000114, -340.2000000000001592 ) ) ;
#1583=ORIENTED_EDGE ( 'NONE', *, *, #30240, .F. ) ;
#1589=CARTESIAN_POINT ( 'NONE',  ( -5.000000000000000000, 175.0000000000000284, -350.0000000000002274 ) ) ;
#1600=DIRECTION ( 'NONE',  ( 0.000000000000000000, 0.000000000000000000, -1.000000000000000000 ) ) ;
#1604=DIRECTION ( 'NONE',  ( 0.000000000000000000, 0.000000000000000000, 1.000000000000000000 ) ) ;
#1606=CARTESIAN_POINT ( 'NONE',  ( 168.9999999999999716, -256.4999999999999432, -349.9999999999999432 ) ) ;
#1609=CARTESIAN_POINT ( 'NONE',  ( 183.0000000000000284, 2.775557561562891351E-14, -111.0000000000001563 ) ) ;
#1612=ORIENTED_EDGE ( 'NONE', *, *, #40096, .F. ) ;
#1615=CYLINDRICAL_SURFACE ( 'NONE', #5829, 4.000000000000003553 ) ;
#1622=ORIENTED_EDGE ( 'NONE', *, *, #18111, .T. ) ;
#1640=ADVANCED_FACE ( 'NONE', ( #18697 ), #19729, .F. ) ;
#1643=DIRECTION ( 'NONE',  ( -1.000000000000000000, 0.000000000000000000, 0.000000000000000000 ) ) ;
#1644=CARTESIAN_POINT ( 'NONE',  ( 181.0000000000000284, -9.999999999999953815, -97.00000000000014211 ) ) ;
#1645=ORIENTED_EDGE ( 'NONE', *, *, #40228, .T. ) ;
#1647=DIRECTION ( 'NONE',  ( -0.000000000000000000, -0.000000000000000000, 1.000000000000000000 ) ) ;
#1655=ORIENTED_EDGE ( 'NONE', *, *, #46232, .F. ) ;
#1659=DIRECTION ( 'NONE',  ( 0.000000000000000000, 2.537652627714642000E-15, 1.000000000000000000 ) ) ;
#1668=CARTESIAN_POINT ( 'NONE',  ( 169.0000000000000000, -174.9999999999999716, -115.0000000000001563 ) ) ;
#1680=CARTESIAN_POINT ( 'NONE',  ( 185.0000000000000000, -93.49999999999997158, -115.0000000000001563 ) ) ;
#1685=ORIENTED_EDGE ( 'NONE', *, *, #39068, .F. ) ;
#1688=CARTESIAN_POINT ( 'NONE',  ( 341.9999999999999432, -169.0000000000001137, -344.0000000000002842 ) ) ;
#1690=EDGE_CURVE ( 'NONE', #32484, #24437, #16703, .T. ) ;
#1692=LINE ( 'NONE', #37373, #33868 ) ;
#1698=AXIS2_PLACEMENT_3D ( 'NONE', #6620, #22275, #38696 ) ;
#1702=CIRCLE ( 'NONE', #49186, 2.000000000000001776 ) ;
#1722=FACE_OUTER_BOUND ( 'NONE', #20432, .T. ) ;
#1724=ADVANCED_FACE ( 'NONE', ( #23579 ), #22557, .T. ) ;
#1731=ORIENTED_EDGE ( 'NONE', *, *, #10149, .F. ) ;
#1733=EDGE_CURVE ( 'NONE', #27742, #2419, #8705, .T. ) ;
#1740=PLANE ( 'NONE',  #4006 ) ;
#1742=LINE ( 'NONE', #9179, #8730 ) ;
#1749=EDGE_CURVE ( 'NONE', #8266, #33773, #42921, .T. ) ;
#1753=LINE ( 'NONE', #10453, #28621 ) ;
#1757=CARTESIAN_POINT ( 'NONE',  ( 168.9999999999999716, -5.999999999999950262, 339.9999999999998295 ) ) ;
#1758=ORIENTED_EDGE ( 'NONE', *, *, #29451, .T. ) ;
#1760=DIRECTION ( 'NONE',  ( 0.000000000000000000, -1.000000000000000000, 0.000000000000000000 ) ) ;
#1766=AXIS2_PLACEMENT_3D ( 'NONE', #6164, #29765, #40809 ) ;
#1771=DIRECTION ( 'NONE',  ( 0.000000000000000000, 1.000000000000000000, 0.000000000000000000 ) ) ;
#1779=DIRECTION ( 'NONE',  ( -0.000000000000000000, -1.000000000000000000, -0.000000000000000000 ) ) ;
#1781=DIRECTION ( 'NONE',  ( 1.000000000000000000, 0.000000000000000000, 0.000000000000000000 ) ) ;
#1782=ORIENTED_EDGE ( 'NONE', *, *, #10448, .T. ) ;
#1789=ORIENTED_EDGE ( 'NONE', *, *, #37137, .F. ) ;
#1791=DIRECTION ( 'NONE',  ( 0.000000000000000000, 1.000000000000000000, 3.186989995019654210E-49 ) ) ;
#1795=ADVANCED_FACE ( 'NONE', ( #994, #12278 ), #500, .F. ) ;
#1796=CARTESIAN_POINT ( 'NONE',  ( 168.9999999999999716, -180.9999999999999716, -340.0000000000001137 ) ) ;
#1799=DIRECTION ( 'NONE',  ( 4.759647537211363479E-16, -5.772796816983493182E-42, 1.000000000000000000 ) ) ;
#1800=ORIENTED_EDGE ( 'NONE', *, *, #24123, .F. ) ;
#1808=ORIENTED_EDGE ( 'NONE', *, *, #7338, .T. ) ;
#1809=PRODUCT_CONTEXT ( 'NONE', #435, 'mechanical' ) ;
#1811=CARTESIAN_POINT ( 'NONE',  ( 350.0000000000000000, -180.9999999999999716, -342.0000000000001705 ) ) ;
#1831=EDGE_CURVE ( 'NONE', #2097, #37129, #16137, .T. ) ;
#1832=DIRECTION ( 'NONE',  ( 0.000000000000000000, 0.000000000000000000, -1.000000000000000000 ) ) ;
#1833=ORIENTED_EDGE ( 'NONE', *, *, #29322, .T. ) ;
#1841=ORIENTED_EDGE ( 'NONE', *, *, #15312, .T. ) ;
#1847=AXIS2_PLACEMENT_3D ( 'NONE', #32204, #47802, #21146 ) ;
#1855=DIRECTION ( 'NONE',  ( 0.000000000000000000, 0.000000000000000000, -1.000000000000000000 ) ) ;
#1858=DIRECTION ( 'NONE',  ( 0.000000000000000000, 0.000000000000000000, -1.000000000000000000 ) ) ;
#1861=VERTEX_POINT ( 'NONE', #10199 ) ;
#1879=DIRECTION ( 'NONE',  ( 3.172065745548403743E-16, 1.000000000000000000, 0.000000000000000000 ) ) ;
#1885=CIRCLE ( 'NONE', #37936, 4.000000000000003553 ) ;
#1887=ORIENTED_EDGE ( 'NONE', *, *, #32928, .T. ) ;
#1903=DIRECTION ( 'NONE',  ( -1.654361225106055350E-24, -1.654361225106055350E-24, 1.000000000000000000 ) ) ;
#1905=ORIENTED_EDGE ( 'NONE', *, *, #23688, .T. ) ;
#1906=DIRECTION ( 'NONE',  ( 0.000000000000000000, 2.537652627714642000E-15, 1.000000000000000000 ) ) ;
#1907=CARTESIAN_POINT ( 'NONE',  ( 181.0000000000000000, 165.0000000000000000, -342.0000000000001137 ) ) ;
#1908=DIRECTION ( 'NONE',  ( -1.000000000000000000, 0.000000000000000000, 1.860490536778032451E-50 ) ) ;
#1917=CARTESIAN_POINT ( 'NONE',  ( 358.0000000000001137, 181.0000000000000284, 355.9999999999998295 ) ) ;
#1918=DIRECTION ( 'NONE',  ( 5.473822126268816076E-48, -1.000000000000000000, -1.654361225106055350E-24 ) ) ;
#1922=EDGE_CURVE ( 'NONE', #43357, #31210, #34071, .T. ) ;
#1925=ORIENTED_EDGE ( 'NONE', *, *, #50399, .T. ) ;
#1930=CARTESIAN_POINT ( 'NONE',  ( 164.9999999999999716, -174.9999999999999716, -344.0000000000001137 ) ) ;
#1933=CARTESIAN_POINT ( 'NONE',  ( 169.0000000000000284, 165.0000000000000000, 355.9999999999998863 ) ) ;
#1937=DIRECTION ( 'NONE',  ( 0.000000000000000000, 0.000000000000000000, -1.000000000000000000 ) ) ;
#1938=DIRECTION ( 'NONE',  ( -0.000000000000000000, -1.000000000000000000, -0.000000000000000000 ) ) ;
#1939=CARTESIAN_POINT ( 'NONE',  ( 169.0000000000000284, -164.9999999999999432, 357.9999999999998863 ) ) ;
#1940=CARTESIAN_POINT ( 'NONE',  ( 164.9999999999999716, -81.49999999999997158, -350.0000000000001705 ) ) ;
#1942=CYLINDRICAL_SURFACE ( 'NONE', #24536, 2.000000000000001776 ) ;
#1944=CARTESIAN_POINT ( 'NONE',  ( 181.0000000000000000, -81.49999999999997158, -340.0000000000001137 ) ) ;
#1960=CYLINDRICAL_SURFACE ( 'NONE', #905, 4.000000000000003553 ) ;
#1961=AXIS2_PLACEMENT_3D ( 'NONE', #37355, #34239, #45491 ) ;
#1965=ORIENTED_EDGE ( 'NONE', *, *, #42761, .F. ) ;
#1969=DIRECTION ( 'NONE',  ( -1.000000000000000000, 4.996003610813203446E-16, -1.033975765691284226E-24 ) ) ;
#1975=VERTEX_POINT ( 'NONE', #13532 ) ;
#1978=DIRECTION ( 'NONE',  ( 1.000000000000000000, 0.000000000000000000, 0.000000000000000000 ) ) ;
#1981=CARTESIAN_POINT ( 'NONE',  ( 169.0000000000000000, -174.9999999999999716, -97.00000000000014211 ) ) ;
#1982=ORIENTED_EDGE ( 'NONE', *, *, #10169, .F. ) ;
#1987=CARTESIAN_POINT ( 'NONE',  ( 0.000000000000000000, -175.0000000000000284, 350.0000000000002274 ) ) ;
#1988=CARTESIAN_POINT ( 'NONE',  ( 169.0000000000000000, -174.9999999999999716, -95.00000000000014211 ) ) ;
#1998=DIRECTION ( 'NONE',  ( 1.000000000000000000, 0.000000000000000000, 0.000000000000000000 ) ) ;
#1999=EDGE_LOOP ( 'NONE', ( #37853, #12484 ) ) ;
#2010=VECTOR ( 'NONE', #2165, 1000.000000000000000 ) ;
#2018=EDGE_CURVE ( 'NONE', #19301, #5374, #45810, .T. ) ;
#2027=DIRECTION ( 'NONE',  ( -3.364279341222521245E-16, -0.7071067811865474617, 0.7071067811865476838 ) ) ;
#2032=LINE ( 'NONE', #36962, #2633 ) ;
#2033=VECTOR ( 'NONE', #32426, 1000.000000000000000 ) ;
#2035=VERTEX_POINT ( 'NONE', #4525 ) ;
#2038=CARTESIAN_POINT ( 'NONE',  ( 344.0000000000000000, 165.0000000000000000, -340.0000000000001137 ) ) ;
#2040=AXIS2_PLACEMENT_3D ( 'NONE', #24732, #40384, #5220 ) ;
#2045=LINE ( 'NONE', #47938, #29961 ) ;
#2048=DIRECTION ( 'NONE',  ( 0.000000000000000000, -2.537652627714643577E-15, -1.000000000000000000 ) ) ;
#2051=EDGE_LOOP ( 'NONE', ( #4881, #9393, #45610, #17203, #16422, #32497, #38156, #30559 ) ) ;
#2058=ADVANCED_FACE ( 'NONE', ( #39693 ), #31486, .F. ) ;
#2059=VERTEX_POINT ( 'NONE', #47332 ) ;
#2079=ORIENTED_EDGE ( 'NONE', *, *, #4226, .T. ) ;
#2080=EDGE_CURVE ( 'NONE', #26957, #35927, #31747, .T. ) ;
#2081=DIRECTION ( 'NONE',  ( 0.000000000000000000, -1.000000000000000000, -0.000000000000000000 ) ) ;
#2084=AXIS2_PLACEMENT_3D ( 'NONE', #35793, #19594, #621 ) ;
#2092=AXIS2_PLACEMENT_3D ( 'NONE', #39484, #32035, #23299 ) ;
#2097=VERTEX_POINT ( 'NONE', #4278 ) ;
#2099=VECTOR ( 'NONE', #44927, 1000.000000000000000 ) ;
#2103=CARTESIAN_POINT ( 'NONE',  ( 168.9999999999999716, -93.49999999999997158, -115.0000000000001563 ) ) ;
#2106=CARTESIAN_POINT ( 'NONE',  ( 344.0000000000000568, 165.0000000000000000, 339.9999999999998295 ) ) ;
#2107=ORIENTED_EDGE ( 'NONE', *, *, #15288, .T. ) ;
#2115=CARTESIAN_POINT ( 'NONE',  ( 168.9999999999999716, -184.9999999999999716, -360.0000000000002274 ) ) ;
#2122=ORIENTED_EDGE ( 'NONE', *, *, #44011, .T. ) ;
#2125=( GEOMETRIC_REPRESENTATION_CONTEXT ( 3 ) GLOBAL_UNCERTAINTY_ASSIGNED_CONTEXT ( ( #15805 ) ) GLOBAL_UNIT_ASSIGNED_CONTEXT ( ( #47360, #50706, #15603 ) ) REPRESENTATION_CONTEXT ( 'NONE', 'WORKASPACE' ) );
#2132=CARTESIAN_POINT ( 'NONE',  ( 356.0000000000000000, 183.0000000000000284, -358.0000000000002842 ) ) ;
#2134=DIRECTION ( 'NONE',  ( 1.000000000000000000, 0.000000000000000000, -0.000000000000000000 ) ) ;
#2145=ADVANCED_FACE ( 'NONE', ( #38849 ), #14973, .T. ) ;
#2147=EDGE_CURVE ( 'NONE', #4051, #45035, #26522, .T. ) ;
#2149=AXIS2_PLACEMENT_3D ( 'NONE', #39779, #12555, #7716 ) ;
#2154=LINE ( 'NONE', #26261, #29470 ) ;
#2161=VECTOR ( 'NONE', #28800, 1000.000000000000000 ) ;
#2163=EDGE_LOOP ( 'NONE', ( #44906, #42703, #11861, #33184 ) ) ;
#2165=DIRECTION ( 'NONE',  ( 0.000000000000000000, -2.265761274745217480E-16, 1.000000000000000000 ) ) ;
#2167=CARTESIAN_POINT ( 'NONE',  ( 339.9999999999999432, 169.0000000000000000, -360.0000000000002274 ) ) ;
#2168=VECTOR ( 'NONE', #40547, 1000.000000000000000 ) ;
#2175=ORIENTED_EDGE ( 'NONE', *, *, #25307, .F. ) ;
#2176=LINE ( 'NONE', #11381, #9477 ) ;
#2187=CYLINDRICAL_SURFACE ( 'NONE', #42517, 4.000000000000003553 ) ;
#2188=CARTESIAN_POINT ( 'NONE',  ( 168.9999999999999716, -184.9999999999999716, -342.0000000000001137 ) ) ;
#2190=ORIENTED_EDGE ( 'NONE', *, *, #135, .T. ) ;
#2194=FACE_OUTER_BOUND ( 'NONE', #13713, .T. ) ;
#2196=DIRECTION ( 'NONE',  ( 0.000000000000000000, -1.000000000000000000, -3.186989995019654210E-49 ) ) ;
#2198=CYLINDRICAL_SURFACE ( 'NONE', #5680, 2.000000000000001776 ) ;
#2199=CARTESIAN_POINT ( 'NONE',  ( 344.0000000000000000, 185.0000000000000284, -360.0000000000002274 ) ) ;
#2202=VECTOR ( 'NONE', #33848, 1000.000000000000000 ) ;
#2204=EDGE_LOOP ( 'NONE', ( #30820, #13242, #49742, #5430 ) ) ;
#2208=EDGE_CURVE ( 'NONE', #44283, #11192, #19323, .T. ) ;
#2214=CARTESIAN_POINT ( 'NONE',  ( 185.0000000000000000, -81.49999999999997158, -340.0000000000001137 ) ) ;
#2219=ORIENTED_EDGE ( 'NONE', *, *, #45089, .F. ) ;
#2221=ORIENTED_EDGE ( 'NONE', *, *, #5750, .F. ) ;
#2224=LINE ( 'NONE', #40973, #47164 ) ;
#2226=LINE ( 'NONE', #6578, #11231 ) ;
#2227=DIRECTION ( 'NONE',  ( 1.000000000000000000, -4.758098676964956461E-16, -8.975803739141899931E-48 ) ) ;
#2228=VERTEX_POINT ( 'NONE', #15237 ) ;
#2231=CARTESIAN_POINT ( 'NONE',  ( 341.9999999999999432, 169.0000000000000568, -344.0000000000002842 ) ) ;
#2239=CARTESIAN_POINT ( 'NONE',  ( 168.9999999999999716, -9.999999999999953815, -340.0000000000001137 ) ) ;
#2241=DIRECTION ( 'NONE',  ( 0.000000000000000000, 5.664403186863042467E-17, 1.000000000000000000 ) ) ;
#2245=CARTESIAN_POINT ( 'NONE',  ( -5.000000000000000000, 165.2000000000000171, -359.8000000000002387 ) ) ;
#2251=DIRECTION ( 'NONE',  ( 0.000000000000000000, 4.687818848539279227E-49, -1.000000000000000000 ) ) ;
#2252=CARTESIAN_POINT ( 'NONE',  ( 358.0000000000000568, 3.000000000000086153, 177.9999999999998295 ) ) ;
#2270=EDGE_CURVE ( 'NONE', #43944, #27545, #39351, .T. ) ;
#2272=DIRECTION ( 'NONE',  ( -7.793956916774524585E-48, 0.000000000000000000, -1.000000000000000000 ) ) ;
#2274=DIRECTION ( 'NONE',  ( 0.000000000000000000, -1.000000000000000000, -3.186989995019654210E-49 ) ) ;
#2279=AXIS2_PLACEMENT_3D ( 'NONE', #44315, #4588, #1254 ) ;
#2281=FACE_BOUND ( 'NONE', #45381, .T. ) ;
#2286=CARTESIAN_POINT ( 'NONE',  ( 168.9999999999999716, -256.5000000000000000, -114.9999999999999574 ) ) ;
#2298=DIRECTION ( 'NONE',  ( -1.000000000000000000, 4.758098676964957447E-16, 1.586032892321651989E-16 ) ) ;
#2301=CARTESIAN_POINT ( 'NONE',  ( 350.0000000000001137, 169.0000000000000000, 339.9999999999997726 ) ) ;
#2306=CARTESIAN_POINT ( 'NONE',  ( 350.0000000000000000, 165.0000000000000000, -356.0000000000002274 ) ) ;
#2308=CARTESIAN_POINT ( 'NONE',  ( 168.9999999999999716, -272.4999999999999432, -343.9999999999999432 ) ) ;
#2313=EDGE_CURVE ( 'NONE', #26016, #29839, #45378, .T. ) ;
#2322=CARTESIAN_POINT ( 'NONE',  ( -5.000000000000000000, 184.8000000000000114, 340.1999999999997044 ) ) ;
#2328=ORIENTED_EDGE ( 'NONE', *, *, #11109, .F. ) ;
#2339=DIRECTION ( 'NONE',  ( -7.793956916774524585E-48, 0.000000000000000000, -1.000000000000000000 ) ) ;
#2341=ORIENTED_EDGE ( 'NONE', *, *, #41912, .F. ) ;
#2342=CARTESIAN_POINT ( 'NONE',  ( 168.9999999999999716, -95.49999999999998579, -350.0000000000001705 ) ) ;
#2344=PLANE ( 'NONE',  #23482 ) ;
#2347=CARTESIAN_POINT ( 'NONE',  ( 168.9999999999999716, -174.9999999999999716, -344.0000000000001137 ) ) ;
#2355=AXIS2_PLACEMENT_3D ( 'NONE', #30400, #50607, #11660 ) ;
#2360=PLANE ( 'NONE',  #30682 ) ;
#2361=EDGE_CURVE ( 'NONE', #14253, #47520, #3083, .T. ) ;
#2363=CLOSED_SHELL ( 'NONE', ( #3342, #14419, #2748, #34512, #34172, #9170, #15477, #49367, #30911, #4283, #29578, #33056, #33074, #22732, #2145, #35939, #19462, #13002 ) ) ;
#2365=CARTESIAN_POINT ( 'NONE',  ( 185.0000000000000000, -272.5000000000000000, -98.99999999999874944 ) ) ;
#2368=CARTESIAN_POINT ( 'NONE',  ( 344.0000000000000000, 175.0000000000000284, -90.00000000000018474 ) ) ;
#2369=DIRECTION ( 'NONE',  ( -2.220446049250312588E-16, -0.7071067811865475727, -0.7071067811865474617 ) ) ;
#2371=DIRECTION ( 'NONE',  ( 0.000000000000000000, 1.000000000000000000, 0.000000000000000000 ) ) ;
#2372=DIRECTION ( 'NONE',  ( -4.755310728521421461E-16, 0.000000000000000000, -1.000000000000000000 ) ) ;
#2378=DIRECTION ( 'NONE',  ( 1.000000000000000000, 0.000000000000000000, -1.132880637372608740E-16 ) ) ;
#2379=ORIENTED_EDGE ( 'NONE', *, *, #11745, .T. ) ;
#2381=CARTESIAN_POINT ( 'NONE',  ( 168.9999999999999716, 175.0000000000000284, -344.0000000000001137 ) ) ;
#2384=LINE ( 'NONE', #29339, #15161 ) ;
#2386=EDGE_LOOP ( 'NONE', ( #42573, #21078, #47318, #22481 ) ) ;
#2387=CIRCLE ( 'NONE', #17935, 4.000000000000003553 ) ;
#2388=AXIS2_PLACEMENT_3D ( 'NONE', #2308, #25931, #45386 ) ;
#2392=DIRECTION ( 'NONE',  ( 0.000000000000000000, -3.186989995019654210E-49, -1.000000000000000000 ) ) ;
#2393=VECTOR ( 'NONE', #7981, 1000.000000000000000 ) ;
#2396=AXIS2_PLACEMENT_3D ( 'NONE', #6923, #46891, #27436 ) ;
#2401=EDGE_LOOP ( 'NONE', ( #45203, #22728, #47305, #23767 ) ) ;
#2408=LINE ( 'NONE', #34746, #30082 ) ;
#2411=PLANE ( 'NONE',  #25717 ) ;
#2419=VERTEX_POINT ( 'NONE', #38768 ) ;
#2420=LINE ( 'NONE', #18066, #10038 ) ;
#2424=EDGE_CURVE ( 'NONE', #26016, #15667, #10789, .T. ) ;
#2438=AXIS2_PLACEMENT_3D ( 'NONE', #35705, #23368, #545 ) ;
#2447=DIRECTION ( 'NONE',  ( -1.000000000000000000, 0.000000000000000000, 0.000000000000000000 ) ) ;
#2449=VERTEX_POINT ( 'NONE', #46150 ) ;
#2453=ORIENTED_EDGE ( 'NONE', *, *, #25212, .F. ) ;
#2457=EDGE_CURVE ( 'NONE', #48255, #46544, #10294, .T. ) ;
#2460=ORIENTED_EDGE ( 'NONE', *, *, #35958, .T. ) ;
#2467=STYLED_ITEM('',(#50747),#5021);
#2468=DIRECTION ( 'NONE',  ( -1.000000000000000000, -0.000000000000000000, -0.000000000000000000 ) ) ;
#2469=PLANE ( 'NONE',  #47155 ) ;
#2470=DIRECTION ( 'NONE',  ( -1.000000000000000000, 0.000000000000000000, 0.000000000000000000 ) ) ;
#2477=CARTESIAN_POINT ( 'NONE',  ( -5.000000000000000000, 184.8000000000000114, -340.2000000000001592 ) ) ;
#2488=CARTESIAN_POINT ( 'NONE',  ( 344.0000000000000000, -166.9999999999999716, 341.9999999999998295 ) ) ;
#2491=( NAMED_UNIT ( * ) PLANE_ANGLE_UNIT ( ) SI_UNIT ( $, .RADIAN. ) );
#2492=EDGE_CURVE ( 'NONE', #30746, #40029, #27211, .T. ) ;
#2493=CARTESIAN_POINT ( 'NONE',  ( 339.9999999999999432, -169.0000000000001137, -349.9999999999998863 ) ) ;
#2496=CIRCLE ( 'NONE', #16462, 2.000000000000001776 ) ;
#2498=VECTOR ( 'NONE', #50224, 1000.000000000000000 ) ;
#2501=VECTOR ( 'NONE', #18867, 1000.000000000000000 ) ;
#2502=CARTESIAN_POINT ( 'NONE',  ( 168.9999999999999716, -184.9999999999999716, -344.0000000000001137 ) ) ;
#2512=PLANE ( 'NONE',  #24670 ) ;
#2515=ORIENTED_EDGE ( 'NONE', *, *, #16148, .F. ) ;
#2522=DIRECTION ( 'NONE',  ( 0.000000000000000000, 0.000000000000000000, -1.000000000000000000 ) ) ;
#2524=CARTESIAN_POINT ( 'NONE',  ( -5.000000000000000000, 0.000000000000000000, 0.000000000000000000 ) ) ;
#2529=CIRCLE ( 'NONE', #36175, 4.000000000000003553 ) ;
#2541=VERTEX_POINT ( 'NONE', #42839 ) ;
#2545=CYLINDRICAL_SURFACE ( 'NONE', #3046, 3.749999999999975575 ) ;
#2546=ORIENTED_EDGE ( 'NONE', *, *, #32505, .T. ) ;
#2548=ADVANCED_FACE ( 'NONE', ( #4623 ), #20009, .T. ) ;
#2551=VERTEX_POINT ( 'NONE', #20268 ) ;
#2553=LINE ( 'NONE', #37983, #38904 ) ;
#2557=CARTESIAN_POINT ( 'NONE',  ( 168.9999999999999716, -164.9999999999999432, -342.0000000000001137 ) ) ;
#2560=CARTESIAN_POINT ( 'NONE',  ( 183.0000000000000000, -268.4999999999999432, -349.9999999999999432 ) ) ;
#2574=LINE ( 'NONE', #10289, #3246 ) ;
#2577=LINE ( 'NONE', #18223, #6215 ) ;
#2584=CARTESIAN_POINT ( 'NONE',  ( 0.000000000000000000, 169.0000000000000000, -340.0000000000001705 ) ) ;
#2588=LINE ( 'NONE', #49506, #26736 ) ;
#2590=CYLINDRICAL_SURFACE ( 'NONE', #2970, 4.000000000000003553 ) ;
#2596=ORIENTED_EDGE ( 'NONE', *, *, #44123, .T. ) ;
#2600=CARTESIAN_POINT ( 'NONE',  ( 183.0000000000000284, -174.9999999999999716, -111.0000000000001563 ) ) ;
#2604=ORIENTED_EDGE ( 'NONE', *, *, #16925, .T. ) ;
#2610=DIRECTION ( 'NONE',  ( -1.586032892321651989E-16, 8.666415220619855873E-32, -1.000000000000000000 ) ) ;
#2615=CARTESIAN_POINT ( 'NONE',  ( -5.000000000000000000, 175.0000000000000284, 350.0000000000002274 ) ) ;
#2616=DIRECTION ( 'NONE',  ( 0.000000000000000000, -1.000000000000000000, -3.186989995019654210E-49 ) ) ;
#2619=ORIENTED_EDGE ( 'NONE', *, *, #19864, .F. ) ;
#2621=ORIENTED_EDGE ( 'NONE', *, *, #16201, .F. ) ;
#2624=CIRCLE ( 'NONE', #18996, 3.749999999999975575 ) ;
#2629=VERTEX_POINT ( 'NONE', #3853 ) ;
#2633=VECTOR ( 'NONE', #24633, 1000.000000000000000 ) ;
#2637=CARTESIAN_POINT ( 'NONE',  ( 350.0000000000001137, 181.0000000000000284, 359.9999999999997726 ) ) ;
#2638=EDGE_CURVE ( 'NONE', #11949, #7818, #19759, .T. ) ;
#2648=CARTESIAN_POINT ( 'NONE',  ( 185.0000000000000000, -256.4999999999999432, -349.9999999999999432 ) ) ;
#2650=FACE_BOUND ( 'NONE', #33391, .T. ) ;
#2651=ORIENTED_EDGE ( 'NONE', *, *, #19532, .T. ) ;
#2655=EDGE_CURVE ( 'NONE', #15017, #11842, #1531, .T. ) ;
#2664=VECTOR ( 'NONE', #47949, 1000.000000000000000 ) ;
#2674=DIRECTION ( 'NONE',  ( 1.000000000000000000, 0.000000000000000000, 1.612977847700450206E-50 ) ) ;
#2680=DIRECTION ( 'NONE',  ( 0.000000000000000000, 1.000000000000000000, 6.123233995736766036E-17 ) ) ;
#2683=DIRECTION ( 'NONE',  ( 1.000000000000000000, 0.000000000000000000, -4.758098676964956461E-16 ) ) ;
#2685=ADVANCED_FACE ( 'NONE', ( #17173 ), #48921, .T. ) ;
#2690=CARTESIAN_POINT ( 'NONE',  ( 166.9999999999999716, -93.49999999999998579, -350.0000000000001705 ) ) ;
#2693=EDGE_CURVE ( 'NONE', #25153, #19185, #16663, .T. ) ;
#2696=CARTESIAN_POINT ( 'NONE',  ( 341.9999999999999432, -169.0000000000001137, -344.0000000000002842 ) ) ;
#2703=AXIS2_PLACEMENT_3D ( 'NONE', #27519, #26312, #46017 ) ;
#2705=CARTESIAN_POINT ( 'NONE',  ( 181.0000000000000000, -164.9999999999999432, 355.9999999999998863 ) ) ;
#2706=ADVANCED_FACE ( 'NONE', ( #28726 ), #44099, .F. ) ;
#2714=DIRECTION ( 'NONE',  ( 0.000000000000000000, 0.000000000000000000, 1.000000000000000000 ) ) ;
#2717=ORIENTED_EDGE ( 'NONE', *, *, #18899, .T. ) ;
#2719=EDGE_CURVE ( 'NONE', #22911, #25388, #32841, .T. ) ;
#2720=LINE ( 'NONE', #33034, #22236 ) ;
#2721=CARTESIAN_POINT ( 'NONE',  ( 0.000000000000000000, -164.9999999999999432, -356.0000000000002274 ) ) ;
#2723=( BOUNDED_CURVE ( )  B_SPLINE_CURVE ( 3, ( #20348, #32663, #48259, #24213 ),
 .UNSPECIFIED., .F., .F. ) 
 B_SPLINE_CURVE_WITH_KNOTS ( ( 4, 4 ),
 ( 4.712388980384682569, 6.283185307179586232 ),
 .UNSPECIFIED. ) 
 CURVE ( )  GEOMETRIC_REPRESENTATION_ITEM ( )  RATIONAL_B_SPLINE_CURVE ( ( 1.000000000000000000, 0.8047378541243632721, 0.8047378541243632721, 1.000000000000000000 ) ) 
 REPRESENTATION_ITEM ( '' )  );
#2728=ORIENTED_EDGE ( 'NONE', *, *, #167, .F. ) ;
#2731=DIRECTION ( 'NONE',  ( -1.000000000000000000, -0.000000000000000000, -0.000000000000000000 ) ) ;
#2733=AXIS2_PLACEMENT_3D ( 'NONE', #43344, #47167, #770 ) ;
#2746=DIRECTION ( 'NONE',  ( -1.586032892321652236E-16, -1.000000000000000000, -6.853681917100419162E-49 ) ) ;
#2748=ADVANCED_FACE ( 'NONE', ( #37209 ), #24628, .T. ) ;
#2749=ADVANCED_FACE ( 'NONE', ( #33846 ), #42028, .T. ) ;
#2750=CARTESIAN_POINT ( 'NONE',  ( 181.0000000000000000, -252.5000000000000000, -114.9999999999999716 ) ) ;
#2755=CARTESIAN_POINT ( 'NONE',  ( 0.000000000000000000, -165.1999999999999602, -359.8000000000002387 ) ) ;
#2759=ORIENTED_EDGE ( 'NONE', *, *, #28887, .F. ) ;
#2763=ADVANCED_FACE ( 'NONE', ( #14066 ), #30231, .T. ) ;
#2764=ORIENTED_EDGE ( 'NONE', *, *, #43668, .T. ) ;
#2765=FACE_OUTER_BOUND ( 'NONE', #28, .T. ) ;
#2766=VECTOR ( 'NONE', #1025, 1000.000000000000000 ) ;
#2772=DIRECTION ( 'NONE',  ( 0.000000000000000000, -2.969158215481698263E-48, 1.000000000000000000 ) ) ;
#2774=CARTESIAN_POINT ( 'NONE',  ( 181.0000000000000000, -164.9999999999999432, -356.0000000000001705 ) ) ;
#2779=ORIENTED_EDGE ( 'NONE', *, *, #37076, .T. ) ;
#2780=CARTESIAN_POINT ( 'NONE',  ( 340.0000000000000568, 169.0000000000000000, 357.9999999999997726 ) ) ;
#2787=DIRECTION ( 'NONE',  ( -1.000000000000000000, 0.000000000000000000, 1.586032892321651989E-16 ) ) ;
#2793=LINE ( 'NONE', #15874, #12076 ) ;
#2799=DIRECTION ( 'NONE',  ( -1.000000000000000000, 5.326388832052271710E-25, -1.587271980518778491E-16 ) ) ;
#2800=DIRECTION ( 'NONE',  ( 1.000000000000000000, 0.000000000000000000, 0.000000000000000000 ) ) ;
#2814=ORIENTED_EDGE ( 'NONE', *, *, #43072, .F. ) ;
#2818=DIRECTION ( 'NONE',  ( -0.000000000000000000, -0.000000000000000000, 1.000000000000000000 ) ) ;
#2819=ORIENTED_EDGE ( 'NONE', *, *, #38022, .T. ) ;
#2834=CIRCLE ( 'NONE', #13502, 4.000000000000003553 ) ;
#2836=EDGE_LOOP ( 'NONE', ( #15416, #20351, #9369, #19438 ) ) ;
#2845=VERTEX_POINT ( 'NONE', #29728 ) ;
#2847=LINE ( 'NONE', #46690, #18224 ) ;
#2864=VERTEX_POINT ( 'NONE', #22021 ) ;
#2873=ORIENTED_EDGE ( 'NONE', *, *, #943, .F. ) ;
#2876=CARTESIAN_POINT ( 'NONE',  ( 344.0000000000000000, 165.0000000000000000, -106.0000000000001990 ) ) ;
#2881=LINE ( 'NONE', #50053, #43153 ) ;
#2882=DIRECTION ( 'NONE',  ( 0.000000000000000000, 0.000000000000000000, -1.000000000000000000 ) ) ;
#2889=EDGE_LOOP ( 'NONE', ( #8359, #12907, #27713, #1484 ) ) ;
#2895=CARTESIAN_POINT ( 'NONE',  ( 350.0000000000000000, 167.0000000000000000, -356.0000000000002274 ) ) ;
#2897=DIRECTION ( 'NONE',  ( -9.711650524620651178E-33, 1.223873602809432483E-48, -1.000000000000000000 ) ) ;
#2898=VECTOR ( 'NONE', #22285, 1000.000000000000000 ) ;
#2903=CARTESIAN_POINT ( 'NONE',  ( 344.0000000000000000, -167.0000000000001137, 342.0000000000000000 ) ) ;
#2910=VECTOR ( 'NONE', #15592, 1000.000000000000000 ) ;
#2911=DIRECTION ( 'NONE',  ( -1.000000000000000000, 0.000000000000000000, 0.000000000000000000 ) ) ;
#2913=ORIENTED_EDGE ( 'NONE', *, *, #26154, .T. ) ;
#2926=DIRECTION ( 'NONE',  ( -1.000000000000000000, 0.000000000000000000, 0.000000000000000000 ) ) ;
#2928=CIRCLE ( 'NONE', #2149, 4.000000000000003553 ) ;
#2938=VECTOR ( 'NONE', #50385, 1000.000000000000000 ) ;
#2942=STYLED_ITEM('',(#50747),#21395);
#2945=CARTESIAN_POINT ( 'NONE',  ( 0.000000000000000000, -184.7999999999999545, 359.7999999999997840 ) ) ;
#2946=EDGE_CURVE ( 'NONE', #891, #3572, #16803, .T. ) ;
#2948=VERTEX_POINT ( 'NONE', #28353 ) ;
#2953=VERTEX_POINT ( 'NONE', #912 ) ;
#2960=CARTESIAN_POINT ( 'NONE',  ( 344.0000000000000000, -167.0000000000001137, -349.9999999999998863 ) ) ;
#2969=EDGE_CURVE ( 'NONE', #10537, #47246, #45013, .T. ) ;
#2970=AXIS2_PLACEMENT_3D ( 'NONE', #7481, #38785, #33917 ) ;
#2979=VECTOR ( 'NONE', #15930, 1000.000000000000000 ) ;
#2981=DIRECTION ( 'NONE',  ( 0.000000000000000000, 1.000000000000000000, 0.000000000000000000 ) ) ;
#2984=MECHANICAL_DESIGN_GEOMETRIC_PRESENTATION_REPRESENTATION('',(#20173),#3804);
#2987=CARTESIAN_POINT ( 'NONE',  ( 339.9999999999999432, 181.0000000000000284, -344.0000000000001705 ) ) ;
#2988=EDGE_CURVE ( 'NONE', #8719, #14950, #29690, .T. ) ;
#2990=ADVANCED_FACE ( 'NONE', ( #8356 ), #5248, .F. ) ;
#2994=ADVANCED_FACE ( 'NONE', ( #16299 ), #31960, .T. ) ;
#2996=DIRECTION ( 'NONE',  ( -1.000000000000000000, -0.000000000000000000, -0.000000000000000000 ) ) ;
#2999=DIRECTION ( 'NONE',  ( 0.000000000000000000, 0.000000000000000000, 1.000000000000000000 ) ) ;
#3003=AXIS2_PLACEMENT_3D ( 'NONE', #28425, #36657, #24825 ) ;
#3019=CARTESIAN_POINT ( 'NONE',  ( 339.9999999999998863, -168.9999999999999432, 359.9999999999998295 ) ) ;
#3026=LINE ( 'NONE', #46094, #25786 ) ;
#3030=CARTESIAN_POINT ( 'NONE',  ( 356.0000000000000000, -167.0000000000001137, -342.0000000000003411 ) ) ;
#3031=CARTESIAN_POINT ( 'NONE',  ( 350.0000000000000000, -184.9999999999999716, -360.0000000000002274 ) ) ;
#3042=ADVANCED_FACE ( 'NONE', ( #2650, #14191 ), #29862, .T. ) ;
#3046=AXIS2_PLACEMENT_3D ( 'NONE', #25399, #10254, #18187 ) ;
#3051=VERTEX_POINT ( 'NONE', #2167 ) ;
#3053=EDGE_CURVE ( 'NONE', #40413, #29620, #38717, .T. ) ;
#3063=PLANE ( 'NONE',  #26611 ) ;
#3067=CARTESIAN_POINT ( 'NONE',  ( 169.0000000000000000, -184.9999999999999716, -115.0000000000001137 ) ) ;
#3068=ORIENTED_EDGE ( 'NONE', *, *, #48539, .F. ) ;
#3076=AXIS2_PLACEMENT_3D ( 'NONE', #25784, #41431, #22936 ) ;
#3083=LINE ( 'NONE', #23094, #39682 ) ;
#3090=ORIENTED_EDGE ( 'NONE', *, *, #5480, .T. ) ;
#3092=PLANE ( 'NONE',  #35201 ) ;
#3103=ADVANCED_FACE ( 'NONE', ( #10104 ), #40907, .F. ) ;
#3109=EDGE_LOOP ( 'NONE', ( #26223, #41186, #50645, #15630 ) ) ;
#3117=CARTESIAN_POINT ( 'NONE',  ( 339.9999999999999432, 181.0000000000000284, -356.0000000000002274 ) ) ;
#3119=ORIENTED_EDGE ( 'NONE', *, *, #9665, .F. ) ;
#3121=DIRECTION ( 'NONE',  ( 0.000000000000000000, -2.265761274745217480E-16, 1.000000000000000000 ) ) ;
#3122=CARTESIAN_POINT ( 'NONE',  ( 0.000000000000000000, 181.0000000000000284, -358.0000000000002274 ) ) ;
#3125=ORIENTED_EDGE ( 'NONE', *, *, #489, .F. ) ;
#3127=EDGE_LOOP ( 'NONE', ( #32010, #30119, #20434, #19432, #32405, #5133, #24170, #17306 ) ) ;
#3128=DIRECTION ( 'NONE',  ( 0.000000000000000000, 0.000000000000000000, -1.000000000000000000 ) ) ;
#3145=ORIENTED_EDGE ( 'NONE', *, *, #1325, .F. ) ;
#3146=DIRECTION ( 'NONE',  ( -1.000000000000000000, 0.000000000000000000, -1.612977847700450206E-50 ) ) ;
#3148=DIRECTION ( 'NONE',  ( 0.000000000000000000, 1.000000000000000000, 3.186989995019654210E-49 ) ) ;
#3150=PLANE ( 'NONE',  #12025 ) ;
#3158=ORIENTED_EDGE ( 'NONE', *, *, #41068, .F. ) ;
#3161=EDGE_LOOP ( 'NONE', ( #20847, #24621, #34113, #33708 ) ) ;
#3162=PLANE ( 'NONE',  #17396 ) ;
#3165=CARTESIAN_POINT ( 'NONE',  ( 356.0000000000000000, -165.0000000000001137, 339.9999999999999432 ) ) ;
#3168=DIRECTION ( 'NONE',  ( -1.612977847700450206E-50, 0.000000000000000000, -1.000000000000000000 ) ) ;
#3171=ORIENTED_EDGE ( 'NONE', *, *, #26645, .F. ) ;
#3172=EDGE_CURVE ( 'NONE', #43697, #47413, #15239, .T. ) ;
#3174=LINE ( 'NONE', #49089, #37999 ) ;
#3179=VECTOR ( 'NONE', #31098, 1000.000000000000000 ) ;
#3184=AXIS2_PLACEMENT_3D ( 'NONE', #45627, #5893, #29753 ) ;
#3186=EDGE_CURVE ( 'NONE', #10986, #4748, #46729, .T. ) ;
#3187=EDGE_LOOP ( 'NONE', ( #16068, #45085, #15128, #42404 ) ) ;
#3192=ORIENTED_EDGE ( 'NONE', *, *, #28018, .F. ) ;
#3204=ORIENTED_EDGE ( 'NONE', *, *, #45592, .F. ) ;
#3206=CYLINDRICAL_SURFACE ( 'NONE', #16813, 3.749999999999975575 ) ;
#3219=VECTOR ( 'NONE', #30789, 1000.000000000000000 ) ;
#3227=AXIS2_PLACEMENT_3D ( 'NONE', #2876, #41648, #21639 ) ;
#3232=ORIENTED_EDGE ( 'NONE', *, *, #33834, .F. ) ;
#3234=ADVANCED_FACE ( 'NONE', ( #15229 ), #22406, .F. ) ;
#3235=CARTESIAN_POINT ( 'NONE',  ( 181.0000000000000000, -270.5000000000000000, -114.9999999999999147 ) ) ;
#3239=EDGE_CURVE ( 'NONE', #16830, #586, #41153, .T. ) ;
#3243=ORIENTED_EDGE ( 'NONE', *, *, #1225, .F. ) ;
#3246=VECTOR ( 'NONE', #45655, 1000.000000000000000 ) ;
#3248=VERTEX_POINT ( 'NONE', #35005 ) ;
#3251=CYLINDRICAL_SURFACE ( 'NONE', #40962, 2.000000000000001776 ) ;
#3252=ORIENTED_EDGE ( 'NONE', *, *, #4842, .T. ) ;
#3253=DIRECTION ( 'NONE',  ( -1.000000000000000000, 0.000000000000000000, -0.000000000000000000 ) ) ;
#3257=LINE ( 'NONE', #46079, #10237 ) ;
#3262=EDGE_LOOP ( 'NONE', ( #6568, #13904, #48658, #8787, #15034, #39005, #20964, #2515 ) ) ;
#3265=AXIS2_PLACEMENT_3D ( 'NONE', #29791, #37017, #18483 ) ;
#3268=ORIENTED_EDGE ( 'NONE', *, *, #20803, .F. ) ;
#3269=CARTESIAN_POINT ( 'NONE',  ( 0.000000000000000000, -168.9999999999999432, -360.0000000000002274 ) ) ;
#3272=EDGE_CURVE ( 'NONE', #23694, #14722, #50314, .T. ) ;
#3282=ORIENTED_EDGE ( 'NONE', *, *, #15272, .F. ) ;
#3283=VERTEX_POINT ( 'NONE', #19316 ) ;
#3290=AXIS2_PLACEMENT_3D ( 'NONE', #42388, #7253, #38578 ) ;
#3292=CARTESIAN_POINT ( 'NONE',  ( 168.9999999999999716, 165.0000000000000000, -356.0000000000001705 ) ) ;
#3298=CARTESIAN_POINT ( 'NONE',  ( 181.0000000000000000, -174.9999999999999716, -344.0000000000001137 ) ) ;
#3308=DIRECTION ( 'NONE',  ( -2.958228394578793832E-31, 0.000000000000000000, -1.000000000000000000 ) ) ;
#3312=EDGE_CURVE ( 'NONE', #2953, #46163, #28291, .T. ) ;
#3318=VERTEX_POINT ( 'NONE', #16239 ) ;
#3319=DIRECTION ( 'NONE',  ( 0.000000000000000000, -1.000000000000000000, 0.000000000000000000 ) ) ;
#3320=EDGE_CURVE ( 'NONE', #16572, #26176, #25634, .T. ) ;
#3322=CARTESIAN_POINT ( 'NONE',  ( 343.9999999999999432, -185.0000000000001421, -360.0000000000003411 ) ) ;
#3330=CARTESIAN_POINT ( 'NONE',  ( 356.0000000000001137, 185.0000000000000284, 349.9999999999998295 ) ) ;
#3334=CARTESIAN_POINT ( 'NONE',  ( 356.0000000000000000, -174.9999999999999432, 339.9999999999998295 ) ) ;
#3337=EDGE_CURVE ( 'NONE', #31887, #46968, #35500, .T. ) ;
#3342=ADVANCED_FACE ( 'NONE', ( #8800 ), #24451, .T. ) ;
#3343=LINE ( 'NONE', #25251, #28878 ) ;
#3358=CARTESIAN_POINT ( 'NONE',  ( 344.0000000000000568, 165.0000000000000000, 339.9999999999998295 ) ) ;
#3362=AXIS2_PLACEMENT_3D ( 'NONE', #10601, #19310, #2882 ) ;
#3363=ORIENTED_EDGE ( 'NONE', *, *, #4350, .T. ) ;
#3366=CARTESIAN_POINT ( 'NONE',  ( 168.9999999999999716, -174.9999999999999716, -340.0000000000001137 ) ) ;
#3368=DIRECTION ( 'NONE',  ( 0.000000000000000000, 0.000000000000000000, -1.000000000000000000 ) ) ;
#3372=AXIS2_PLACEMENT_3D ( 'NONE', #30630, #11891, #353 ) ;
#3376=PLANE ( 'NONE',  #1006 ) ;
#3392=LINE ( 'NONE', #30879, #29506 ) ;
#3394=VECTOR ( 'NONE', #6579, 1000.000000000000000 ) ;
#3399=DIRECTION ( 'NONE',  ( 0.000000000000000000, 0.000000000000000000, -1.000000000000000000 ) ) ;
#3408=ORIENTED_EDGE ( 'NONE', *, *, #14245, .F. ) ;
#3420=DIRECTION ( 'NONE',  ( -1.000000000000000000, 0.000000000000000000, -4.758098658057970186E-16 ) ) ;
#3422=ORIENTED_EDGE ( 'NONE', *, *, #38744, .F. ) ;
#3428=CARTESIAN_POINT ( 'NONE',  ( 181.0000000000003411, 165.0000000000000000, 341.9999999999998863 ) ) ;
#3431=CARTESIAN_POINT ( 'NONE',  ( 350.0000000000001137, 185.0000000000000284, 343.9999999999997726 ) ) ;
#3435=CIRCLE ( 'NONE', #32132, 2.000000000000001776 ) ;
#3439=EDGE_CURVE ( 'NONE', #34800, #16909, #48597, .T. ) ;
#3440=LINE ( 'NONE', #23202, #28871 ) ;
#3441=VECTOR ( 'NONE', #27335, 1000.000000000000000 ) ;
#3445=CARTESIAN_POINT ( 'NONE',  ( 356.0000000000000000, 175.0000000000000284, -110.0000000000002132 ) ) ;
#3449=CARTESIAN_POINT ( 'NONE',  ( 359.9999999999999432, -165.0000000000001137, -106.0000000000001990 ) ) ;
#3451=EDGE_LOOP ( 'NONE', ( #36840, #5856, #20569, #18117, #14582, #42576, #19182, #46370 ) ) ;
#3454=DIRECTION ( 'NONE',  ( 1.000000000000000000, 0.000000000000000000, 1.612977847700450206E-50 ) ) ;
#3462=ORIENTED_EDGE ( 'NONE', *, *, #24269, .F. ) ;
#3467=DIRECTION ( 'NONE',  ( 0.000000000000000000, 0.000000000000000000, -1.000000000000000000 ) ) ;
#3479=CARTESIAN_POINT ( 'NONE',  ( 168.9999999999999716, -184.9999999999999716, -342.0000000000001137 ) ) ;
#3482=CARTESIAN_POINT ( 'NONE',  ( 356.0000000000001137, 185.0000000000000284, 359.9999999999998295 ) ) ;
#3490=EDGE_CURVE ( 'NONE', #11094, #28407, #10304, .T. ) ;
#3495=VECTOR ( 'NONE', #2298, 1000.000000000000000 ) ;
#3496=CARTESIAN_POINT ( 'NONE',  ( 0.000000000000000000, 169.0000000000000000, 343.9999999999997726 ) ) ;
#3511=ORIENTED_EDGE ( 'NONE', *, *, #33199, .T. ) ;
#3516=ORIENTED_EDGE ( 'NONE', *, *, #41546, .T. ) ;
#3519=DIRECTION ( 'NONE',  ( -1.586032892321652236E-16, -1.000000000000000000, -6.853681917100419162E-49 ) ) ;
#3520=EDGE_CURVE ( 'NONE', #19871, #11669, #41598, .T. ) ;
#3525=DIRECTION ( 'NONE',  ( -1.000000000000000000, 0.000000000000000000, -2.958228394578794270E-31 ) ) ;
#3526=EDGE_CURVE ( 'NONE', #33292, #50656, #50146, .T. ) ;
#3527=DIRECTION ( 'NONE',  ( 0.000000000000000000, 0.000000000000000000, 1.000000000000000000 ) ) ;
#3537=EDGE_CURVE ( 'NONE', #25776, #3827, #22096, .T. ) ;
#3542=( LENGTH_UNIT ( ) NAMED_UNIT ( * ) SI_UNIT ( .MILLI., .METRE. ) );
#3544=LINE ( 'NONE', #34121, #37892 ) ;
#3547=CIRCLE ( 'NONE', #37977, 4.000000000000003553 ) ;
#3551=CARTESIAN_POINT ( 'NONE',  ( 0.000000000000000000, 184.8000000000000114, 359.7999999999997840 ) ) ;
#3554=EDGE_CURVE ( 'NONE', #48314, #3283, #8429, .T. ) ;
#3568=CARTESIAN_POINT ( 'NONE',  ( 168.9999999999999716, -166.9999999999999432, -350.0000000000001705 ) ) ;
#3572=VERTEX_POINT ( 'NONE', #34941 ) ;
#3578=FACE_OUTER_BOUND ( 'NONE', #13186, .T. ) ;
#3582=ORIENTED_EDGE ( 'NONE', *, *, #24464, .F. ) ;
#3585=EDGE_CURVE ( 'NONE', #47178, #12755, #26452, .T. ) ;
#3587=VERTEX_POINT ( 'NONE', #6955 ) ;
#3595=ORIENTED_EDGE ( 'NONE', *, *, #9327, .F. ) ;
#3598=EDGE_CURVE ( 'NONE', #8209, #33697, #26206, .T. ) ;
#3603=CARTESIAN_POINT ( 'NONE',  ( 181.0000000000000000, 175.0000000000000284, -344.0000000000001137 ) ) ;
#3609=CARTESIAN_POINT ( 'NONE',  ( 339.9999999999999432, 169.0000000000000000, -342.0000000000001705 ) ) ;
#3612=CARTESIAN_POINT ( 'NONE',  ( 0.000000000000000000, -175.0000000000000284, -350.0000000000002274 ) ) ;
#3615=VECTOR ( 'NONE', #15292, 1000.000000000000000 ) ;
#3621=EDGE_LOOP ( 'NONE', ( #43249, #780, #29487, #20056 ) ) ;
#3622=AXIS2_PLACEMENT_3D ( 'NONE', #24895, #36459, #1300 ) ;
#3626=CARTESIAN_POINT ( 'NONE',  ( 5.551115123125782702E-14, -168.9999999999999432, 339.9999999999997726 ) ) ;
#3627=ADVANCED_FACE ( 'NONE', ( #34421 ), #3092, .F. ) ;
#3628=EDGE_CURVE ( 'NONE', #35494, #45431, #34342, .T. ) ;
#3640=ADVANCED_FACE ( 'NONE', ( #14399 ), #34678, .F. ) ;
#3645=DIRECTION ( 'NONE',  ( 0.000000000000000000, 2.537652627714642000E-15, 1.000000000000000000 ) ) ;
#3646=ORIENTED_EDGE ( 'NONE', *, *, #43668, .F. ) ;
#3648=DIRECTION ( 'NONE',  ( 1.860490536778032451E-50, 0.000000000000000000, -1.000000000000000000 ) ) ;
#3653=DIRECTION ( 'NONE',  ( -1.000000000000000000, 0.000000000000000000, 0.000000000000000000 ) ) ;
#3655=CARTESIAN_POINT ( 'NONE',  ( 343.9999999999998863, -165.0000000000001137, -110.0000000000002132 ) ) ;
#3658=VERTEX_POINT ( 'NONE', #49502 ) ;
#3660=CARTESIAN_POINT ( 'NONE',  ( 5.551115123125782702E-14, -168.9999999999999432, 339.9999999999997726 ) ) ;
#3664=ORIENTED_EDGE ( 'NONE', *, *, #13355, .T. ) ;
#3668=LINE ( 'NONE', #31659, #25168 ) ;
#3677=AXIS2_PLACEMENT_3D ( 'NONE', #31623, #43385, #23902 ) ;
#3681=LINE ( 'NONE', #23699, #15884 ) ;
#3684=ORIENTED_EDGE ( 'NONE', *, *, #43166, .T. ) ;
#3687=CARTESIAN_POINT ( 'NONE',  ( 350.0000000000000000, 181.0000000000000284, -342.0000000000001705 ) ) ;
#3688=DIRECTION ( 'NONE',  ( -1.000000000000000000, 0.000000000000000000, 1.586032892321651989E-16 ) ) ;
#3692=EDGE_CURVE ( 'NONE', #22226, #28031, #43117, .T. ) ;
#3694=CARTESIAN_POINT ( 'NONE',  ( 4.999999999999999112, -175.0000000000000284, 346.2500000000002274 ) ) ;
#3702=CARTESIAN_POINT ( 'NONE',  ( 183.0000000000000000, -272.4999999999999432, -356.0000000000001705 ) ) ;
#3707=CARTESIAN_POINT ( 'NONE',  ( 350.0000000000001137, 169.0000000000000000, 355.9999999999997726 ) ) ;
#3708=ORIENTED_EDGE ( 'NONE', *, *, #5550, .T. ) ;
#3716=LINE ( 'NONE', #43470, #31128 ) ;
#3717=DIRECTION ( 'NONE',  ( 0.000000000000000000, 2.537652627714642000E-15, 1.000000000000000000 ) ) ;
#3721=CARTESIAN_POINT ( 'NONE',  ( 181.0000000000000000, 8.000000000000062172, -340.0000000000001137 ) ) ;
#3723=AXIS2_PLACEMENT_3D ( 'NONE', #10567, #45186, #2371 ) ;
#3729=VECTOR ( 'NONE', #42933, 1000.000000000000000 ) ;
#3734=CIRCLE ( 'NONE', #38991, 3.749999999999975575 ) ;
#3738=ORIENTED_EDGE ( 'NONE', *, *, #16114, .T. ) ;
#3741=DIRECTION ( 'NONE',  ( 7.793956916774525800E-48, 0.000000000000000000, 1.000000000000000000 ) ) ;
#3743=ORIENTED_EDGE ( 'NONE', *, *, #48497, .F. ) ;
#3751=ORIENTED_EDGE ( 'NONE', *, *, #9821, .F. ) ;
#3757=AXIS2_PLACEMENT_3D ( 'NONE', #37588, #17056, #33476 ) ;
#3761=VECTOR ( 'NONE', #19467, 1000.000000000000000 ) ;
#3763=EDGE_CURVE ( 'NONE', #17953, #42814, #31332, .T. ) ;
#3767=MECHANICAL_DESIGN_GEOMETRIC_PRESENTATION_REPRESENTATION('',(#48780),#46328);
#3773=CIRCLE ( 'NONE', #43113, 4.000000000000003553 ) ;
#3774=EDGE_LOOP ( 'NONE', ( #34613, #34237, #18842, #18030 ) ) ;
#3776=DIRECTION ( 'NONE',  ( 0.000000000000000000, -0.000000000000000000, 1.000000000000000000 ) ) ;
#3790=PLANE ( 'NONE',  #24 ) ;
#3792=AXIS2_PLACEMENT_3D ( 'NONE', #8237, #35194, #35952 ) ;
#3795=EDGE_CURVE ( 'NONE', #25569, #6330, #43356, .T. ) ;
#3802=LINE ( 'NONE', #8424, #49042 ) ;
#3804=( GEOMETRIC_REPRESENTATION_CONTEXT ( 3 ) GLOBAL_UNCERTAINTY_ASSIGNED_CONTEXT ( ( #44071 ) ) GLOBAL_UNIT_ASSIGNED_CONTEXT ( ( #19723, #46878, #43572 ) ) REPRESENTATION_CONTEXT ( 'NONE', 'WORKASPACE' ) );
#3808=DIRECTION ( 'NONE',  ( 1.000000000000000000, 0.000000000000000000, 2.958228394578794270E-31 ) ) ;
#3809=VERTEX_POINT ( 'NONE', #4124 ) ;
#3816=FACE_OUTER_BOUND ( 'NONE', #13441, .T. ) ;
#3821=ORIENTED_EDGE ( 'NONE', *, *, #16569, .F. ) ;
#3823=LINE ( 'NONE', #38492, #3761 ) ;
#3827=VERTEX_POINT ( 'NONE', #8230 ) ;
#3829=CARTESIAN_POINT ( 'NONE',  ( 0.000000000000000000, -180.9999999999999716, -340.0000000000001705 ) ) ;
#3835=CARTESIAN_POINT ( 'NONE',  ( 343.9999999999999432, -165.0000000000001137, -106.0000000000001990 ) ) ;
#3837=DIRECTION ( 'NONE',  ( -4.758098676964956461E-16, 0.000000000000000000, -1.000000000000000000 ) ) ;
#3850=VERTEX_POINT ( 'NONE', #32595 ) ;
#3853=CARTESIAN_POINT ( 'NONE',  ( 356.0000000000006253, 167.0000000000000000, 341.9999999999998863 ) ) ;
#3854=VERTEX_POINT ( 'NONE', #5373 ) ;
#3856=CARTESIAN_POINT ( 'NONE',  ( 344.0000000000000568, 181.0000000000000284, 349.9999999999998295 ) ) ;
#3857=EDGE_CURVE ( 'NONE', #21703, #29662, #29319, .T. ) ;
#3859=ADVANCED_FACE ( 'NONE', ( #36967 ), #37464, .F. ) ;
#3865=FACE_OUTER_BOUND ( 'NONE', #49674, .T. ) ;
#3873=ORIENTED_EDGE ( 'NONE', *, *, #9412, .T. ) ;
#3874=FACE_OUTER_BOUND ( 'NONE', #19231, .T. ) ;
#3875=DIRECTION ( 'NONE',  ( 1.000000000000000000, 0.000000000000000000, -1.586032892321651989E-16 ) ) ;
#3877=EDGE_CURVE ( 'NONE', #8815, #47173, #13814, .T. ) ;
#3880=DIRECTION ( 'NONE',  ( -1.586032892321652236E-16, -1.000000000000000000, -2.288264760618012091E-48 ) ) ;
#3883=EDGE_CURVE ( 'NONE', #34447, #17617, #20770, .T. ) ;
#3886=VERTEX_POINT ( 'NONE', #48930 ) ;
#3892=CARTESIAN_POINT ( 'NONE',  ( 344.0000000000000000, 174.9999999999996589, -344.0000000000002842 ) ) ;
#3894=DIRECTION ( 'NONE',  ( 3.172065745548403743E-16, 1.000000000000000000, 0.000000000000000000 ) ) ;
#3895=AXIS2_PLACEMENT_3D ( 'NONE', #12157, #20101, #1378 ) ;
#3902=CARTESIAN_POINT ( 'NONE',  ( 181.0000000000000000, -184.9999999999999716, -342.0000000000001137 ) ) ;
#3903=ORIENTED_EDGE ( 'NONE', *, *, #13705, .F. ) ;
#3904=CARTESIAN_POINT ( 'NONE',  ( 5.551115123125782702E-14, -168.9999999999999432, 359.9999999999997726 ) ) ;
#3905=DIRECTION ( 'NONE',  ( 0.000000000000000000, 0.000000000000000000, -1.000000000000000000 ) ) ;
#3913=ADVANCED_FACE ( 'NONE', ( #2281, #21788 ), #44851, .F. ) ;
#3918=EDGE_CURVE ( 'NONE', #34995, #13154, #32326, .T. ) ;
#3931=CARTESIAN_POINT ( 'NONE',  ( 185.0000000000000284, -180.9999999999993747, -115.0000000000001279 ) ) ;
#3939=CARTESIAN_POINT ( 'NONE',  ( 344.0000000000000000, 175.0000000000000284, -94.00000000000019895 ) ) ;
#3942=DIRECTION ( 'NONE',  ( -1.368455531567204171E-48, 1.000000000000000000, 2.265761274745217480E-16 ) ) ;
#3944=( NAMED_UNIT ( * ) PLANE_ANGLE_UNIT ( ) SI_UNIT ( $, .RADIAN. ) );
#3946=LINE ( 'NONE', #19079, #14545 ) ;
#3959=ORIENTED_EDGE ( 'NONE', *, *, #50304, .T. ) ;
#3962=DIRECTION ( 'NONE',  ( 0.000000000000000000, -2.265761274745217480E-16, 1.000000000000000000 ) ) ;
#3963=ORIENTED_EDGE ( 'NONE', *, *, #13651, .T. ) ;
#3967=CARTESIAN_POINT ( 'NONE',  ( 183.0000000000000568, 175.0000000000000284, 355.9999999999998863 ) ) ;
#3970=CLOSED_SHELL ( 'NONE', ( #5604, #21662, #14912, #36988, #40306, #22135, #14564, #29609, #3913, #4055, #40441, #39067, #37568, #15185, #49985, #11877, #2685, #16782 ) ) ;
#3979=FACE_OUTER_BOUND ( 'NONE', #5848, .T. ) ;
#3987=EDGE_CURVE ( 'NONE', #20660, #10986, #48211, .T. ) ;
#3991=VERTEX_POINT ( 'NONE', #33855 ) ;
#3994=DIRECTION ( 'NONE',  ( -1.000000000000000000, -0.000000000000000000, -0.000000000000000000 ) ) ;
#3995=ORIENTED_EDGE ( 'NONE', *, *, #23764, .T. ) ;
#3996=EDGE_LOOP ( 'NONE', ( #13400, #28611, #38508, #24216 ) ) ;
#4002=UNCERTAINTY_MEASURE_WITH_UNIT (LENGTH_MEASURE( 1.000000000000000082E-05 ), #34161, 'distance_accuracy_value', 'NONE');
#4003=VERTEX_POINT ( 'NONE', #50453 ) ;
#4006=AXIS2_PLACEMENT_3D ( 'NONE', #17381, #17135, #21731 ) ;
#4007=EDGE_LOOP ( 'NONE', ( #3068, #30208, #39787, #782 ) ) ;
#4010=CARTESIAN_POINT ( 'NONE',  ( 181.0000000000000000, -164.9999999999999432, -350.0000000000001705 ) ) ;
#4013=VECTOR ( 'NONE', #39558, 1000.000000000000000 ) ;
#4014=VERTEX_POINT ( 'NONE', #2780 ) ;
#4026=CARTESIAN_POINT ( 'NONE',  ( 183.0000000000000568, 175.0000000000000284, 343.9999999999998863 ) ) ;
#4028=VERTEX_POINT ( 'NONE', #18428 ) ;
#4029=DIRECTION ( 'NONE',  ( -1.000000000000000000, 0.000000000000000000, -7.793956916774525800E-48 ) ) ;
#4030=CARTESIAN_POINT ( 'NONE',  ( 181.0000000000000284, -174.9999999999999716, -113.0000000000001563 ) ) ;
#4032=DIRECTION ( 'NONE',  ( -1.000000000000000000, 0.000000000000000000, 0.000000000000000000 ) ) ;
#4035=ORIENTED_EDGE ( 'NONE', *, *, #24733, .F. ) ;
#4042=EDGE_CURVE ( 'NONE', #18475, #55, #46609, .T. ) ;
#4043=AXIS2_PLACEMENT_3D ( 'NONE', #40755, #1508, #13033 ) ;
#4046=FACE_OUTER_BOUND ( 'NONE', #4196, .T. ) ;
#4048=( GEOMETRIC_REPRESENTATION_CONTEXT ( 3 ) GLOBAL_UNCERTAINTY_ASSIGNED_CONTEXT ( ( #38700 ) ) GLOBAL_UNIT_ASSIGNED_CONTEXT ( ( #20976, #36658, #48372 ) ) REPRESENTATION_CONTEXT ( 'NONE', 'WORKASPACE' ) );
#4051=VERTEX_POINT ( 'NONE', #15361 ) ;
#4054=DIRECTION ( 'NONE',  ( 1.000000000000000000, -3.172065784643302499E-16, -1.942330104924128867E-32 ) ) ;
#4055=ADVANCED_FACE ( 'NONE', ( #14842 ), #30494, .F. ) ;
#4057=AXIS2_PLACEMENT_3D ( 'NONE', #24752, #36814, #43720 ) ;
#4065=EDGE_CURVE ( 'NONE', #24372, #6656, #22031, .T. ) ;
#4067=PRODUCT_DEFINITION_SHAPE ( 'NONE', 'NONE',  #6792 ) ;
#4081=DIRECTION ( 'NONE',  ( 0.000000000000000000, 1.000000000000000000, 7.004339610132985974E-48 ) ) ;
#4089=LINE ( 'NONE', #19471, #3219 ) ;
#4090=EDGE_CURVE ( 'NONE', #11678, #7132, #7150, .T. ) ;
#4094=EDGE_CURVE ( 'NONE', #14213, #34995, #39982, .T. ) ;
#4103=ORIENTED_EDGE ( 'NONE', *, *, #35044, .F. ) ;
#4106=EDGE_LOOP ( 'NONE', ( #5600, #5557, #11696, #10221 ) ) ;
#4109=ORIENTED_EDGE ( 'NONE', *, *, #35919, .F. ) ;
#4113=VERTEX_POINT ( 'NONE', #43803 ) ;
#4115=AXIS2_PLACEMENT_3D ( 'NONE', #4245, #30424, #43231 ) ;
#4124=CARTESIAN_POINT ( 'NONE',  ( 168.9999999999999716, -164.9999999999999432, 339.9999999999997726 ) ) ;
#4128=AXIS2_PLACEMENT_3D ( 'NONE', #35136, #26655, #23821 ) ;
#4147=CYLINDRICAL_SURFACE ( 'NONE', #7760, 2.000000000000001776 ) ;
#4154=DIRECTION ( 'NONE',  ( 1.333906992743555050E-23, -1.000000000000000000, 0.000000000000000000 ) ) ;
#4163=LINE ( 'NONE', #39836, #23280 ) ;
#4170=CARTESIAN_POINT ( 'NONE',  ( 359.9999999999999432, 181.0000000000002274, -356.0000000000003411 ) ) ;
#4172=LINE ( 'NONE', #19302, #49987 ) ;
#4179=EDGE_CURVE ( 'NONE', #48410, #42209, #3802, .T. ) ;
#4182=DIRECTION ( 'NONE',  ( 0.000000000000000000, 2.969158215481698263E-48, -1.000000000000000000 ) ) ;
#4184=EDGE_LOOP ( 'NONE', ( #47272, #39256, #17712, #24398 ) ) ;
#4186=EDGE_CURVE ( 'NONE', #6015, #18793, #33541, .T. ) ;
#4196=EDGE_LOOP ( 'NONE', ( #24393, #2122, #39598, #1151 ) ) ;
#4201=EDGE_CURVE ( 'NONE', #20632, #2059, #39478, .T. ) ;
#4209=( NAMED_UNIT ( * ) SI_UNIT ( $, .STERADIAN. ) SOLID_ANGLE_UNIT ( ) );
#4226=EDGE_CURVE ( 'NONE', #11669, #31642, #27373, .T. ) ;
#4227=ORIENTED_EDGE ( 'NONE', *, *, #1690, .T. ) ;
#4232=ORIENTED_EDGE ( 'NONE', *, *, #23170, .F. ) ;
#4233=DIRECTION ( 'NONE',  ( 1.586032892321652236E-16, 1.000000000000000000, 2.288264760618012091E-48 ) ) ;
#4236=ORIENTED_EDGE ( 'NONE', *, *, #28320, .F. ) ;
#4239=EDGE_CURVE ( 'NONE', #5007, #44276, #10595, .T. ) ;
#4242=ORIENTED_EDGE ( 'NONE', *, *, #17612, .F. ) ;
#4243=EDGE_CURVE ( 'NONE', #15209, #25755, #24335, .T. ) ;
#4245=CARTESIAN_POINT ( 'NONE',  ( 350.0000000000000000, 169.0000000000000000, -340.0000000000001705 ) ) ;
#4268=CARTESIAN_POINT ( 'NONE',  ( 181.0000000000000000, -270.4999999999999432, -339.9999999999998863 ) ) ;
#4277=CARTESIAN_POINT ( 'NONE',  ( 360.0000000000000568, 175.0000000000000284, -94.00000000000019895 ) ) ;
#4278=CARTESIAN_POINT ( 'NONE',  ( 341.9999999999999432, 181.0000000000001705, -356.0000000000003411 ) ) ;
#4281=MANIFOLD_SOLID_BREP ( 'Cut-Extrude1[2]', #49809 ) ;
#4283=ADVANCED_FACE ( 'NONE', ( #13255 ), #28920, .F. ) ;
#4312=FACE_OUTER_BOUND ( 'NONE', #10861, .T. ) ;
#4313=CARTESIAN_POINT ( 'NONE',  ( 185.0000000000000000, -256.4999999999999432, -339.9999999999999432 ) ) ;
#4319=ORIENTED_EDGE ( 'NONE', *, *, #5775, .F. ) ;
#4320=ORIENTED_EDGE ( 'NONE', *, *, #23459, .T. ) ;
#4323=DIRECTION ( 'NONE',  ( 2.874857526315639190E-31, -1.000000000000000000, 2.537652627714642000E-15 ) ) ;
#4328=DIRECTION ( 'NONE',  ( 0.000000000000000000, -1.000000000000000000, 0.000000000000000000 ) ) ;
#4336=DIRECTION ( 'NONE',  ( -1.586032880504786307E-16, 1.654361225106055350E-24, -1.000000000000000000 ) ) ;
#4344=EDGE_LOOP ( 'NONE', ( #19608, #49372, #18854, #12937, #4227, #10937, #4320, #34801 ) ) ;
#4346=EDGE_CURVE ( 'NONE', #23180, #25776, #50129, .T. ) ;
#4350=EDGE_CURVE ( 'NONE', #24372, #46042, #30176, .T. ) ;
#4354=EDGE_LOOP ( 'NONE', ( #8608, #27915, #8498, #19628 ) ) ;
#4357=CARTESIAN_POINT ( 'NONE',  ( 181.0000000000000000, -272.5000000000000000, -110.9999999999999005 ) ) ;
#4364=ORIENTED_EDGE ( 'NONE', *, *, #12501, .T. ) ;
#4373=ORIENTED_EDGE ( 'NONE', *, *, #17362, .F. ) ;
#4380=ORIENTED_EDGE ( 'NONE', *, *, #427, .T. ) ;
#4385=CARTESIAN_POINT ( 'NONE',  ( 350.0000000000000000, 169.0000000000000000, -344.0000000000001705 ) ) ;
#4397=CIRCLE ( 'NONE', #28174, 2.000000000000001776 ) ;
#4404=( GEOMETRIC_REPRESENTATION_CONTEXT ( 3 ) GLOBAL_UNCERTAINTY_ASSIGNED_CONTEXT ( ( #35331 ) ) GLOBAL_UNIT_ASSIGNED_CONTEXT ( ( #46966, #14238, #23660 ) ) REPRESENTATION_CONTEXT ( 'NONE', 'WORKASPACE' ) );
#4417=ORIENTED_EDGE ( 'NONE', *, *, #3337, .T. ) ;
#4418=VECTOR ( 'NONE', #39610, 1000.000000000000000 ) ;
#4422=CARTESIAN_POINT ( 'NONE',  ( 343.9999999999993747, -183.0000000000000000, 357.9999999999998295 ) ) ;
#4425=CYLINDRICAL_SURFACE ( 'NONE', #17665, 2.000000000000001776 ) ;
#4433=DIRECTION ( 'NONE',  ( 1.612977847700450206E-50, 0.000000000000000000, -1.000000000000000000 ) ) ;
#4435=DIRECTION ( 'NONE',  ( -1.586032892321652236E-16, -1.000000000000000000, -2.288264760618012091E-48 ) ) ;
#4436=CIRCLE ( 'NONE', #38068, 2.000000000000001776 ) ;
#4438=( GEOMETRIC_REPRESENTATION_CONTEXT ( 3 ) GLOBAL_UNCERTAINTY_ASSIGNED_CONTEXT ( ( #23426 ) ) GLOBAL_UNIT_ASSIGNED_CONTEXT ( ( #10973, #50166, #38953 ) ) REPRESENTATION_CONTEXT ( 'NONE', 'WORKASPACE' ) );
#4442=CARTESIAN_POINT ( 'NONE',  ( 185.0000000000000000, -180.9999999999999716, -350.0000000000001705 ) ) ;
#4444=VERTEX_POINT ( 'NONE', #2721 ) ;
#4445=MANIFOLD_SOLID_BREP ( 'Square tube 20 X 20 X 2(1)[10]', #47371 ) ;
#4448=CARTESIAN_POINT ( 'NONE',  ( 339.9999999999998863, -181.0000000000001990, -356.0000000000003411 ) ) ;
#4450=FACE_OUTER_BOUND ( 'NONE', #35951, .T. ) ;
#4455=PLANE ( 'NONE',  #8129 ) ;
#4457=CARTESIAN_POINT ( 'NONE',  ( 350.0000000000000000, 165.0000000000000000, -340.0000000000001705 ) ) ;
#4469=EDGE_CURVE ( 'NONE', #14362, #45172, #37649, .T. ) ;
#4473=VERTEX_POINT ( 'NONE', #10428 ) ;
#4475=LINE ( 'NONE', #42450, #21265 ) ;
#4477=EDGE_CURVE ( 'NONE', #4444, #24185, #33794, .T. ) ;
#4479=ORIENTED_EDGE ( 'NONE', *, *, #24296, .T. ) ;
#4481=CARTESIAN_POINT ( 'NONE',  ( 169.0000000000000000, 2.775557561562891351E-14, -97.00000000000014211 ) ) ;
#4488=CARTESIAN_POINT ( 'NONE',  ( 169.0000000000000284, 175.0000000000000284, 357.9999999999998863 ) ) ;
#4489=CARTESIAN_POINT ( 'NONE',  ( 165.0000000000000284, 175.0000000000000284, 339.9999999999998863 ) ) ;
#4491=CARTESIAN_POINT ( 'NONE',  ( 339.9999999999999432, 174.9999999999996589, -344.0000000000002842 ) ) ;
#4508=( NAMED_UNIT ( * ) PLANE_ANGLE_UNIT ( ) SI_UNIT ( $, .RADIAN. ) );
#4514=LINE ( 'NONE', #20402, #1033 ) ;
#4515=ORIENTED_EDGE ( 'NONE', *, *, #45651, .F. ) ;
#4525=CARTESIAN_POINT ( 'NONE',  ( 356.0000000000000000, 167.0000000000001990, -342.0000000000002842 ) ) ;
#4528=EDGE_CURVE ( 'NONE', #25778, #15830, #47310, .T. ) ;
#4530=DIRECTION ( 'NONE',  ( -1.000000000000000000, 0.000000000000000000, -7.793956916774525800E-48 ) ) ;
#4532=DIRECTION ( 'NONE',  ( -0.000000000000000000, 1.544785076050074834E-48, 1.000000000000000000 ) ) ;
#4534=EDGE_CURVE ( 'NONE', #40413, #41767, #47563, .T. ) ;
#4556=ADVANCED_FACE ( 'NONE', ( #31459 ), #24270, .T. ) ;
#4561=ADVANCED_FACE ( 'NONE', ( #1175 ), #28601, .T. ) ;
#4565=DIRECTION ( 'NONE',  ( 0.000000000000000000, -1.000000000000000000, -3.186989995019654210E-49 ) ) ;
#4573=CIRCLE ( 'NONE', #479, 2.000000000000001776 ) ;
#4577=LINE ( 'NONE', #20224, #22970 ) ;
#4583=VECTOR ( 'NONE', #38297, 1000.000000000000000 ) ;
#4588=DIRECTION ( 'NONE',  ( -1.000000000000000000, 4.105366553918459587E-48, 1.586032880504786307E-16 ) ) ;
#4596=EDGE_LOOP ( 'NONE', ( #30129, #44161, #27134, #24118 ) ) ;
#4608=ORIENTED_EDGE ( 'NONE', *, *, #3877, .F. ) ;
#4610=DIRECTION ( 'NONE',  ( 1.000000000000000000, 0.000000000000000000, 1.612977847700450206E-50 ) ) ;
#4614=ORIENTED_EDGE ( 'NONE', *, *, #23802, .F. ) ;
#4619=EDGE_CURVE ( 'NONE', #35739, #48420, #23779, .T. ) ;
#4621=DIRECTION ( 'NONE',  ( -4.996003610813203446E-16, -1.000000000000000000, 0.000000000000000000 ) ) ;
#4622=FACE_OUTER_BOUND ( 'NONE', #43088, .T. ) ;
#4623=FACE_OUTER_BOUND ( 'NONE', #36457, .T. ) ;
#4624=CARTESIAN_POINT ( 'NONE',  ( 168.9999999999999147, -272.5000000000000000, -96.99999999999988631 ) ) ;
#4633=ORIENTED_EDGE ( 'NONE', *, *, #7158, .T. ) ;
#4636=CARTESIAN_POINT ( 'NONE',  ( 344.0000000000000568, 165.0000000000000000, 339.9999999999998295 ) ) ;
#4641=CARTESIAN_POINT ( 'NONE',  ( 169.0000000000000000, 2.775557561562891351E-14, -115.0000000000001563 ) ) ;
#4642=EDGE_CURVE ( 'NONE', #13147, #6226, #49255, .T. ) ;
#4651=ORIENTED_EDGE ( 'NONE', *, *, #28220, .F. ) ;
#4654=CARTESIAN_POINT ( 'NONE',  ( 181.0000000000000000, -93.49999999999998579, -350.0000000000001705 ) ) ;
#4655=DIRECTION ( 'NONE',  ( -0.000000000000000000, -1.000000000000000000, -0.000000000000000000 ) ) ;
#4663=DIRECTION ( 'NONE',  ( 0.000000000000000000, 0.000000000000000000, -1.000000000000000000 ) ) ;
#4667=EDGE_LOOP ( 'NONE', ( #3743, #25148, #44337, #20755 ) ) ;
#4673=DIRECTION ( 'NONE',  ( 0.000000000000000000, -1.000000000000000000, 0.000000000000000000 ) ) ;
#4674=EDGE_LOOP ( 'NONE', ( #39071, #15651, #40427, #12695 ) ) ;
#4675=EDGE_CURVE ( 'NONE', #30474, #19896, #34182, .T. ) ;
#4679=ORIENTED_EDGE ( 'NONE', *, *, #44953, .F. ) ;
#4686=DIRECTION ( 'NONE',  ( 0.000000000000000000, 1.000000000000000000, -7.004339610132985974E-48 ) ) ;
#4695=CARTESIAN_POINT ( 'NONE',  ( 166.9999999999999716, -180.9999999999999716, -340.0000000000001137 ) ) ;
#4697=ADVANCED_FACE ( 'NONE', ( #6705 ), #30572, .F. ) ;
#4703=DIRECTION ( 'NONE',  ( -1.586032880504786307E-16, 1.654361225106055350E-24, -1.000000000000000000 ) ) ;
#4709=VERTEX_POINT ( 'NONE', #50009 ) ;
#4719=CARTESIAN_POINT ( 'NONE',  ( 341.9999999999999432, 169.0000000000001990, -344.0000000000002842 ) ) ;
#4721=EDGE_LOOP ( 'NONE', ( #30390, #101, #27010, #3516 ) ) ;
#4724=DIRECTION ( 'NONE',  ( 0.000000000000000000, 0.000000000000000000, 1.000000000000000000 ) ) ;
#4732=DIRECTION ( 'NONE',  ( 0.000000000000000000, 0.000000000000000000, -1.000000000000000000 ) ) ;
#4733=LINE ( 'NONE', #20375, #38965 ) ;
#4740=ORIENTED_EDGE ( 'NONE', *, *, #15770, .F. ) ;
#4741=VERTEX_POINT ( 'NONE', #18502 ) ;
#4746=ORIENTED_EDGE ( 'NONE', *, *, #46903, .T. ) ;
#4748=VERTEX_POINT ( 'NONE', #42359 ) ;
#4759=ORIENTED_EDGE ( 'NONE', *, *, #41700, .T. ) ;
#4765=DIRECTION ( 'NONE',  ( -1.000000000000000000, 0.000000000000000000, 0.000000000000000000 ) ) ;
#4772=DIRECTION ( 'NONE',  ( -0.000000000000000000, 1.000000000000000000, 0.000000000000000000 ) ) ;
#4774=CARTESIAN_POINT ( 'NONE',  ( 343.9999999999993747, -183.0000000000000000, 357.9999999999998295 ) ) ;
#4782=DIRECTION ( 'NONE',  ( -3.172065784643302499E-16, -1.000000000000000000, 2.537652627714642000E-15 ) ) ;
#4787=ORIENTED_EDGE ( 'NONE', *, *, #20326, .F. ) ;
#4789=CARTESIAN_POINT ( 'NONE',  ( 0.000000000000000000, -165.1999999999999602, 359.7999999999997840 ) ) ;
#4801=ORIENTED_EDGE ( 'NONE', *, *, #37775, .F. ) ;
#4808=EDGE_CURVE ( 'NONE', #11842, #39424, #45925, .T. ) ;
#4810=DIRECTION ( 'NONE',  ( 0.000000000000000000, 1.000000000000000000, 0.000000000000000000 ) ) ;
#4816=LINE ( 'NONE', #48135, #43873 ) ;
#4824=DIRECTION ( 'NONE',  ( 0.000000000000000000, -1.000000000000000000, -0.000000000000000000 ) ) ;
#4826=EDGE_CURVE ( 'NONE', #13377, #46801, #19773, .T. ) ;
#4829=EDGE_CURVE ( 'NONE', #25755, #24963, #8991, .T. ) ;
#4830=EDGE_LOOP ( 'NONE', ( #10, #3738, #28768, #18671 ) ) ;
#4831=LINE ( 'NONE', #47394, #28905 ) ;
#4833=VECTOR ( 'NONE', #35972, 1000.000000000000000 ) ;
#4841=CYLINDRICAL_SURFACE ( 'NONE', #35859, 2.000000000000001776 ) ;
#4842=EDGE_CURVE ( 'NONE', #25256, #46047, #1042, .T. ) ;
#4844=CARTESIAN_POINT ( 'NONE',  ( 165.0000000000000000, -174.9999999999999716, -115.0000000000001563 ) ) ;
#4848=ORIENTED_EDGE ( 'NONE', *, *, #17713, .F. ) ;
#4849=DIRECTION ( 'NONE',  ( 1.000000000000000000, 0.000000000000000000, 0.000000000000000000 ) ) ;
#4850=CARTESIAN_POINT ( 'NONE',  ( 181.0000000000000000, -256.5000000000000000, -114.9999999999999574 ) ) ;
#4860=ORIENTED_EDGE ( 'NONE', *, *, #44400, .T. ) ;
#4865=DIRECTION ( 'NONE',  ( 1.000000000000000000, 0.000000000000000000, 0.000000000000000000 ) ) ;
#4880=DIRECTION ( 'NONE',  ( -1.000000000000000000, 0.000000000000000000, 0.000000000000000000 ) ) ;
#4881=ORIENTED_EDGE ( 'NONE', *, *, #49715, .T. ) ;
#4884=VECTOR ( 'NONE', #27836, 1000.000000000000000 ) ;
#4885=CARTESIAN_POINT ( 'NONE',  ( 360.0000000000000000, 165.0000000000000000, -106.0000000000001990 ) ) ;
#4886=CARTESIAN_POINT ( 'NONE',  ( 168.9999999999999147, -182.9999999999999716, -340.0000000000001137 ) ) ;
#4891=CARTESIAN_POINT ( 'NONE',  ( 183.0000000000000000, 6.000000000000060396, -340.0000000000001137 ) ) ;
#4901=ORIENTED_EDGE ( 'NONE', *, *, #35450, .F. ) ;
#4906=CARTESIAN_POINT ( 'NONE',  ( 344.0000000000000000, -165.0000000000001137, -349.9999999999999432 ) ) ;
#4907=CIRCLE ( 'NONE', #10656, 4.000000000000003553 ) ;
#4910=CIRCLE ( 'NONE', #30304, 4.000000000000003553 ) ;
#4911=EDGE_CURVE ( 'NONE', #46936, #20632, #30350, .T. ) ;
#4919=VECTOR ( 'NONE', #33797, 1000.000000000000000 ) ;
#4922=ORIENTED_EDGE ( 'NONE', *, *, #5195, .T. ) ;
#4926=ORIENTED_EDGE ( 'NONE', *, *, #7368, .F. ) ;
#4932=DIRECTION ( 'NONE',  ( 0.000000000000000000, 0.000000000000000000, 1.000000000000000000 ) ) ;
#4935=DIRECTION ( 'NONE',  ( 0.000000000000000000, 0.000000000000000000, 1.000000000000000000 ) ) ;
#4947=CIRCLE ( 'NONE', #3290, 2.000000000000001776 ) ;
#4950=DIRECTION ( 'NONE',  ( 1.000000000000000000, -1.586032997072805650E-16, -4.759647537211363479E-16 ) ) ;
#4954=CARTESIAN_POINT ( 'NONE',  ( 356.0000000000001137, 185.0000000000000284, 359.9999999999998295 ) ) ;
#4957=EDGE_LOOP ( 'NONE', ( #34276, #33944, #15179, #17325 ) ) ;
#4960=AXIS2_PLACEMENT_3D ( 'NONE', #922, #47566, #16308 ) ;
#4961=AXIS2_PLACEMENT_3D ( 'NONE', #35075, #19126, #50644 ) ;
#4963=AXIS2_PLACEMENT_3D ( 'NONE', #10016, #44629, #36745 ) ;
#4968=ORIENTED_EDGE ( 'NONE', *, *, #16129, .T. ) ;
#4971=LINE ( 'NONE', #1394, #33610 ) ;
#4973=LINE ( 'NONE', #5229, #45981 ) ;
#4979=EDGE_CURVE ( 'NONE', #42541, #19163, #14084, .T. ) ;
#4983=ORIENTED_EDGE ( 'NONE', *, *, #31542, .F. ) ;
#4984=FACE_BOUND ( 'NONE', #6640, .T. ) ;
#5002=EDGE_LOOP ( 'NONE', ( #34463, #19470, #9346, #1309 ) ) ;
#5007=VERTEX_POINT ( 'NONE', #33865 ) ;
#5010=DIRECTION ( 'NONE',  ( 0.000000000000000000, 0.000000000000000000, -1.000000000000000000 ) ) ;
#5013=FACE_OUTER_BOUND ( 'NONE', #34492, .T. ) ;
#5014=PLANE ( 'NONE',  #47391 ) ;
#5021=MANIFOLD_SOLID_BREP ( 'Square tube 20 X 20 X 2(1)[17]', #722 ) ;
#5029=VERTEX_POINT ( 'NONE', #26145 ) ;
#5032=DIRECTION ( 'NONE',  ( 3.172065745548403743E-16, 1.000000000000000000, 0.000000000000000000 ) ) ;
#5036=CARTESIAN_POINT ( 'NONE',  ( 181.0000000000000284, -174.9999999999999716, -99.00000000000014211 ) ) ;
#5037=VERTEX_POINT ( 'NONE', #14853 ) ;
#5038=ORIENTED_EDGE ( 'NONE', *, *, #6128, .F. ) ;
#5051=FACE_OUTER_BOUND ( 'NONE', #31565, .T. ) ;
#5059=DIRECTION ( 'NONE',  ( -3.172065784643302499E-16, -1.000000000000000000, 2.537652627714642000E-15 ) ) ;
#5060=CARTESIAN_POINT ( 'NONE',  ( 0.000000000000000000, -184.7999999999999545, 340.1999999999997044 ) ) ;
#5062=EDGE_CURVE ( 'NONE', #24255, #26993, #38722, .T. ) ;
#5064=DIRECTION ( 'NONE',  ( 0.000000000000000000, 0.000000000000000000, -1.000000000000000000 ) ) ;
#5083=ORIENTED_EDGE ( 'NONE', *, *, #42429, .T. ) ;
#5084=CARTESIAN_POINT ( 'NONE',  ( 181.0000000000000284, -182.9999999999999716, -340.0000000000001137 ) ) ;
#5090=DIRECTION ( 'NONE',  ( 1.000000000000000000, 0.000000000000000000, 0.000000000000000000 ) ) ;
#5095=ORIENTED_EDGE ( 'NONE', *, *, #12796, .T. ) ;
#5098=EDGE_CURVE ( 'NONE', #35933, #22449, #36081, .T. ) ;
#5099=EDGE_LOOP ( 'NONE', ( #8851, #44841, #22069, #50245 ) ) ;
#5102=MANIFOLD_SOLID_BREP ( 'Square tube 20 X 20 X 2(1)[4]', #21186 ) ;
#5103=VERTEX_POINT ( 'NONE', #30256 ) ;
#5107=DIRECTION ( 'NONE',  ( -0.000000000000000000, 1.000000000000000000, 0.000000000000000000 ) ) ;
#5108=AXIS2_PLACEMENT_3D ( 'NONE', #18291, #13940, #14460 ) ;
#5111=ORIENTED_EDGE ( 'NONE', *, *, #11475, .T. ) ;
#5116=CARTESIAN_POINT ( 'NONE',  ( 339.9999999999999432, -171.9999999999998863, 346.9999999999998295 ) ) ;
#5120=CARTESIAN_POINT ( 'NONE',  ( -5.000000000000000000, 184.8000000000000114, 340.1999999999997044 ) ) ;
#5122=DIRECTION ( 'NONE',  ( -1.612977847700450206E-50, 0.000000000000000000, -1.000000000000000000 ) ) ;
#5123=EDGE_CURVE ( 'NONE', #36547, #14416, #47531, .T. ) ;
#5128=CARTESIAN_POINT ( 'NONE',  ( 183.0000000000000000, -164.9999999999999432, -356.0000000000001705 ) ) ;
#5133=ORIENTED_EDGE ( 'NONE', *, *, #3795, .F. ) ;
#5136=EDGE_CURVE ( 'NONE', #46920, #25256, #4577, .T. ) ;
#5137=LINE ( 'NONE', #12841, #2664 ) ;
#5140=PLANE ( 'NONE',  #42523 ) ;
#5141=CARTESIAN_POINT ( 'NONE',  ( 181.0000000000000284, 2.775557561562891351E-14, -113.0000000000001563 ) ) ;
#5144=ORIENTED_EDGE ( 'NONE', *, *, #8038, .T. ) ;
#5148=LINE ( 'NONE', #36744, #14333 ) ;
#5150=CARTESIAN_POINT ( 'NONE',  ( -5.000000000000000000, 165.2000000000000171, 359.7999999999997840 ) ) ;
#5151=EDGE_LOOP ( 'NONE', ( #47247, #28527, #3595, #14498 ) ) ;
#5153=ORIENTED_EDGE ( 'NONE', *, *, #19035, .T. ) ;
#5154=ADVANCED_FACE ( 'NONE', ( #40231 ), #27671, .F. ) ;
#5155=PLANE ( 'NONE',  #28610 ) ;
#5170=CARTESIAN_POINT ( 'NONE',  ( 339.9999999999998863, -168.9999999999999432, 339.9999999999997726 ) ) ;
#5175=ORIENTED_EDGE ( 'NONE', *, *, #31986, .F. ) ;
#5179=( BOUNDED_CURVE ( )  B_SPLINE_CURVE ( 3, ( #25306, #21444, #40462, #48859 ),
 .UNSPECIFIED., .F., .F. ) 
 B_SPLINE_CURVE_WITH_KNOTS ( ( 4, 4 ),
 ( 1.570796326794896780, 3.141592653589793116 ),
 .UNSPECIFIED. ) 
 CURVE ( )  GEOMETRIC_REPRESENTATION_ITEM ( )  RATIONAL_B_SPLINE_CURVE ( ( 1.000000000000000000, 0.8047378541243650485, 0.8047378541243650485, 1.000000000000000000 ) ) 
 REPRESENTATION_ITEM ( '' )  );
#5182=DIRECTION ( 'NONE',  ( 6.203854594147707562E-25, -2.067951531382569187E-25, 1.000000000000000000 ) ) ;
#5184=EDGE_CURVE ( 'NONE', #38709, #9291, #35281, .T. ) ;
#5185=ORIENTED_EDGE ( 'NONE', *, *, #3628, .F. ) ;
#5188=CARTESIAN_POINT ( 'NONE',  ( 342.0000000000000000, 165.0000000000000000, -106.0000000000001990 ) ) ;
#5195=EDGE_CURVE ( 'NONE', #31812, #8645, #12515, .T. ) ;
#5202=CARTESIAN_POINT ( 'NONE',  ( 181.0000000000000000, -174.9999999999999716, -360.0000000000001705 ) ) ;
#5211=CARTESIAN_POINT ( 'NONE',  ( 355.9999999999998863, -185.0000000000002558, -360.0000000000003411 ) ) ;
#5220=DIRECTION ( 'NONE',  ( 0.000000000000000000, 0.000000000000000000, 1.000000000000000000 ) ) ;
#5221=VECTOR ( 'NONE', #20152, 1000.000000000000000 ) ;
#5222=CARTESIAN_POINT ( 'NONE',  ( 181.0000000000000000, -184.9999999999999716, -340.0000000000001137 ) ) ;
#5225=CARTESIAN_POINT ( 'NONE',  ( 181.0000000000000000, -184.9999999999999716, -356.0000000000001705 ) ) ;
#5229=CARTESIAN_POINT ( 'NONE',  ( 181.0000000000000000, -166.9999999999999432, -350.0000000000001705 ) ) ;
#5232=CARTESIAN_POINT ( 'NONE',  ( 181.0000000000000000, -256.5000000000000000, -114.9999999999999574 ) ) ;
#5235=DIRECTION ( 'NONE',  ( 1.586032892321651989E-16, -8.666415220619855873E-32, 1.000000000000000000 ) ) ;
#5242=AXIS2_PLACEMENT_3D ( 'NONE', #4654, #5900, #14605 ) ;
#5245=DIRECTION ( 'NONE',  ( -1.860490536778032451E-50, 0.000000000000000000, 1.000000000000000000 ) ) ;
#5246=CYLINDRICAL_SURFACE ( 'NONE', #21674, 2.000000000000001776 ) ;
#5248=PLANE ( 'NONE',  #28891 ) ;
#5250=ORIENTED_EDGE ( 'NONE', *, *, #17713, .T. ) ;
#5251=ORIENTED_EDGE ( 'NONE', *, *, #37371, .T. ) ;
#5252=LINE ( 'NONE', #27857, #43890 ) ;
#5275=AXIS2_PLACEMENT_3D ( 'NONE', #33892, #22578, #42072 ) ;
#5281=AXIS2_PLACEMENT_3D ( 'NONE', #42718, #26838, #38911 ) ;
#5282=DIRECTION ( 'NONE',  ( 6.203854594147707562E-25, -2.067951531382569187E-25, 1.000000000000000000 ) ) ;
#5292=CARTESIAN_POINT ( 'NONE',  ( 181.0000000000000568, 175.0000000000000284, 339.9999999999998863 ) ) ;
#5293=CARTESIAN_POINT ( 'NONE',  ( 342.8284271247460993, 183.0000000000002558, -358.0000000000002842 ) ) ;
#5300=ORIENTED_EDGE ( 'NONE', *, *, #42207, .T. ) ;
#5302=DIRECTION ( 'NONE',  ( 1.000000000000000000, 0.000000000000000000, 0.000000000000000000 ) ) ;
#5304=VERTEX_POINT ( 'NONE', #21474 ) ;
#5305=ORIENTED_EDGE ( 'NONE', *, *, #14245, .T. ) ;
#5324=CARTESIAN_POINT ( 'NONE',  ( 360.0000000000001137, -172.0000000000000000, -3.000000000000058620 ) ) ;
#5326=DIRECTION ( 'NONE',  ( -3.172065745548403743E-16, -1.000000000000000000, 0.000000000000000000 ) ) ;
#5327=AXIS2_PLACEMENT_3D ( 'NONE', #3117, #7235, #50532 ) ;
#5333=EDGE_CURVE ( 'NONE', #47613, #980, #40488, .T. ) ;
#5337=DIRECTION ( 'NONE',  ( 9.711650524620651178E-33, -1.223873602809432483E-48, 1.000000000000000000 ) ) ;
#5340=ORIENTED_EDGE ( 'NONE', *, *, #28158, .F. ) ;
#5343=CARTESIAN_POINT ( 'NONE',  ( 181.0000000000000284, -174.9999999999999716, -115.0000000000001563 ) ) ;
#5348=EDGE_LOOP ( 'NONE', ( #11752, #34730, #47560, #9812 ) ) ;
#5350=EDGE_LOOP ( 'NONE', ( #17797, #28284, #30245, #12155 ) ) ;
#5352=CARTESIAN_POINT ( 'NONE',  ( 181.0000000000000000, -182.9999999999999716, -350.0000000000001705 ) ) ;
#5363=DIRECTION ( 'NONE',  ( -5.551115123125782086E-17, -0.7071067811865475727, -0.7071067811865474617 ) ) ;
#5373=CARTESIAN_POINT ( 'NONE',  ( 356.0000000000001137, 165.0000000000000000, -108.0000000000002132 ) ) ;
#5374=VERTEX_POINT ( 'NONE', #46313 ) ;
#5375=VECTOR ( 'NONE', #24342, 1000.000000000000000 ) ;
#5376=EDGE_LOOP ( 'NONE', ( #3204, #47357, #7903, #27457 ) ) ;
#5385=ORIENTED_EDGE ( 'NONE', *, *, #20891, .F. ) ;
#5391=ORIENTED_EDGE ( 'NONE', *, *, #27997, .F. ) ;
#5398=CARTESIAN_POINT ( 'NONE',  ( 342.0000000000000000, 182.1715728752538439, 357.1715728752535597 ) ) ;
#5413=ADVANCED_FACE ( 'NONE', ( #30185 ), #41992, .F. ) ;
#5416=VECTOR ( 'NONE', #26952, 1000.000000000000000 ) ;
#5417=EDGE_CURVE ( 'NONE', #40834, #34025, #18627, .T. ) ;
#5419=VERTEX_POINT ( 'NONE', #3479 ) ;
#5428=DIRECTION ( 'NONE',  ( 0.000000000000000000, 7.004339610132985974E-48, 1.000000000000000000 ) ) ;
#5430=ORIENTED_EDGE ( 'NONE', *, *, #35263, .T. ) ;
#5436=CARTESIAN_POINT ( 'NONE',  ( -5.000000000000000000, 0.000000000000000000, 0.000000000000000000 ) ) ;
#5444=ORIENTED_EDGE ( 'NONE', *, *, #37795, .F. ) ;
#5454=EDGE_CURVE ( 'NONE', #14517, #7888, #6588, .T. ) ;
#5457=ORIENTED_EDGE ( 'NONE', *, *, #30071, .F. ) ;
#5460=LINE ( 'NONE', #9807, #33466 ) ;
#5465=VERTEX_POINT ( 'NONE', #46050 ) ;
#5476=CARTESIAN_POINT ( 'NONE',  ( 341.9999999999999432, -174.9999999999999432, 355.9999999999998295 ) ) ;
#5480=EDGE_CURVE ( 'NONE', #28586, #19058, #43753, .T. ) ;
#5489=ORIENTED_EDGE ( 'NONE', *, *, #50415, .T. ) ;
#5490=ORIENTED_EDGE ( 'NONE', *, *, #45364, .T. ) ;
#5501=ORIENTED_EDGE ( 'NONE', *, *, #36731, .F. ) ;
#5508=VECTOR ( 'NONE', #28679, 1000.000000000000000 ) ;
#5509=EDGE_CURVE ( 'NONE', #34922, #35337, #4514, .T. ) ;
#5512=CARTESIAN_POINT ( 'NONE',  ( 356.0000000000000000, 165.0000000000000000, -340.0000000000001137 ) ) ;
#5515=EDGE_LOOP ( 'NONE', ( #33670, #14415, #34675, #18540 ) ) ;
#5520=DIRECTION ( 'NONE',  ( 0.000000000000000000, 1.000000000000000000, 6.123233995736766036E-17 ) ) ;
#5534=DIRECTION ( 'NONE',  ( 3.172065745548403743E-16, 1.000000000000000000, 0.000000000000000000 ) ) ;
#5550=EDGE_CURVE ( 'NONE', #29259, #20258, #29373, .T. ) ;
#5557=ORIENTED_EDGE ( 'NONE', *, *, #34410, .T. ) ;
#5564=CARTESIAN_POINT ( 'NONE',  ( 185.0000000000000284, -174.9999999999999716, -99.00000000000014211 ) ) ;
#5576=VECTOR ( 'NONE', #2369, 1000.000000000000000 ) ;
#5584=DIRECTION ( 'NONE',  ( 1.000000000000000000, 0.000000000000000000, 0.000000000000000000 ) ) ;
#5586=FACE_OUTER_BOUND ( 'NONE', #11858, .T. ) ;
#5599=EDGE_CURVE ( 'NONE', #31636, #25458, #33247, .T. ) ;
#5600=ORIENTED_EDGE ( 'NONE', *, *, #7631, .T. ) ;
#5604=ADVANCED_FACE ( 'NONE', ( #44989 ), #49076, .T. ) ;
#5610=MANIFOLD_SOLID_BREP ( 'Cut-Extrude1[4]', #1534 ) ;
#5611=ORIENTED_EDGE ( 'NONE', *, *, #25632, .F. ) ;
#5612=DIRECTION ( 'NONE',  ( -1.000000000000000000, 0.000000000000000000, 0.000000000000000000 ) ) ;
#5613=DIRECTION ( 'NONE',  ( 0.000000000000000000, -2.265761274745217480E-16, 1.000000000000000000 ) ) ;
#5619=FACE_OUTER_BOUND ( 'NONE', #10615, .T. ) ;
#5623=EDGE_LOOP ( 'NONE', ( #19375, #43841, #13617, #30615 ) ) ;
#5634=LINE ( 'NONE', #45369, #34347 ) ;
#5640=EDGE_CURVE ( 'NONE', #49297, #5007, #37852, .T. ) ;
#5648=CARTESIAN_POINT ( 'NONE',  ( 342.0000000000000568, 181.0000000000000568, 355.9999999999998295 ) ) ;
#5659=ORIENTED_EDGE ( 'NONE', *, *, #5854, .T. ) ;
#5674=DIRECTION ( 'NONE',  ( 7.793956916774525800E-48, 0.000000000000000000, 1.000000000000000000 ) ) ;
#5679=LINE ( 'NONE', #6690, #27598 ) ;
#5680=AXIS2_PLACEMENT_3D ( 'NONE', #28889, #44507, #42883 ) ;
#5687=AXIS2_PLACEMENT_3D ( 'NONE', #12505, #39729, #32029 ) ;
#5693=CARTESIAN_POINT ( 'NONE',  ( 0.000000000000000000, -180.9999999999999716, -344.0000000000001705 ) ) ;
#5702=DIRECTION ( 'NONE',  ( 4.996003610813203446E-16, 1.000000000000000000, 0.000000000000000000 ) ) ;
#5707=CARTESIAN_POINT ( 'NONE',  ( -5.000000000000000000, 184.8000000000000114, 359.7999999999997840 ) ) ;
#5709=CARTESIAN_POINT ( 'NONE',  ( 168.9999999999999716, -180.9999999999999716, -340.0000000000001137 ) ) ;
#5713=ORIENTED_EDGE ( 'NONE', *, *, #47402, .T. ) ;
#5716=DIRECTION ( 'NONE',  ( 0.000000000000000000, 0.000000000000000000, -1.000000000000000000 ) ) ;
#5719=CIRCLE ( 'NONE', #34418, 2.000000000000001776 ) ;
#5720=CARTESIAN_POINT ( 'NONE',  ( 350.0000000000000000, -174.9999999999999716, -350.0000000000002274 ) ) ;
#5721=EDGE_LOOP ( 'NONE', ( #18465, #39616, #33856, #13679 ) ) ;
#5723=DIRECTION ( 'NONE',  ( 0.000000000000000000, 0.000000000000000000, -1.000000000000000000 ) ) ;
#5729=VERTEX_POINT ( 'NONE', #3165 ) ;
#5740=PLANE ( 'NONE',  #25497 ) ;
#5741=ADVANCED_FACE ( 'NONE', ( #47211 ), #8014, .F. ) ;
#5747=VERTEX_POINT ( 'NONE', #1065 ) ;
#5750=EDGE_CURVE ( 'NONE', #37243, #46256, #23903, .T. ) ;
#5752=PLANE ( 'NONE',  #39008 ) ;
#5754=EDGE_CURVE ( 'NONE', #19349, #21703, #39825, .T. ) ;
#5755=CARTESIAN_POINT ( 'NONE',  ( 4.999999999999999112, -175.0000000000000284, 350.0000000000002274 ) ) ;
#5759=AXIS2_PLACEMENT_3D ( 'NONE', #46305, #19648, #27351 ) ;
#5773=DIRECTION ( 'NONE',  ( 0.000000000000000000, -1.000000000000000000, 0.000000000000000000 ) ) ;
#5775=EDGE_CURVE ( 'NONE', #24618, #32124, #12595, .T. ) ;
#5776=LINE ( 'NONE', #37106, #36448 ) ;
#5781=DIRECTION ( 'NONE',  ( 0.000000000000000000, 1.000000000000000000, 0.000000000000000000 ) ) ;
#5793=VECTOR ( 'NONE', #49364, 1000.000000000000000 ) ;
#5796=EDGE_CURVE ( 'NONE', #39156, #5803, #31203, .T. ) ;
#5801=CARTESIAN_POINT ( 'NONE',  ( 344.0000000000000000, 183.0000000000000284, 357.9999999999998863 ) ) ;
#5803=VERTEX_POINT ( 'NONE', #41319 ) ;
#5806=DIRECTION ( 'NONE',  ( 0.000000000000000000, -2.265761274745217480E-16, 1.000000000000000000 ) ) ;
#5813=ORIENTED_EDGE ( 'NONE', *, *, #3987, .T. ) ;
#5816=LINE ( 'NONE', #37147, #10321 ) ;
#5829=AXIS2_PLACEMENT_3D ( 'NONE', #17507, #36020, #17258 ) ;
#5830=DIRECTION ( 'NONE',  ( 0.000000000000000000, 1.000000000000000000, 0.000000000000000000 ) ) ;
#5839=VECTOR ( 'NONE', #49149, 1000.000000000000000 ) ;
#5841=ADVANCED_FACE ( 'NONE', ( #17463 ), #29266, .T. ) ;
#5845=EDGE_CURVE ( 'NONE', #21498, #50507, #9077, .T. ) ;
#5847=LINE ( 'NONE', #21488, #42915 ) ;
#5848=EDGE_LOOP ( 'NONE', ( #16107, #30418, #1318, #15537 ) ) ;
#5854=EDGE_CURVE ( 'NONE', #46920, #12938, #27938, .T. ) ;
#5856=ORIENTED_EDGE ( 'NONE', *, *, #49764, .T. ) ;
#5860=AXIS2_PLACEMENT_3D ( 'NONE', #33793, #2227, #37648 ) ;
#5865=FACE_OUTER_BOUND ( 'NONE', #49027, .T. ) ;
#5870=CARTESIAN_POINT ( 'NONE',  ( 357.9999999999999432, -178.0000000000000000, 352.9999999999998295 ) ) ;
#5871=DIRECTION ( 'NONE',  ( -2.220446049250312588E-16, -0.7071067811865475727, 0.7071067811865474617 ) ) ;
#5874=CARTESIAN_POINT ( 'NONE',  ( 339.9999999999999432, 167.0000000000000000, -344.0000000000001705 ) ) ;
#5889=EDGE_CURVE ( 'NONE', #37542, #31812, #21309, .T. ) ;
#5893=DIRECTION ( 'NONE',  ( 1.000000000000000000, 0.000000000000000000, 2.958228394578794270E-31 ) ) ;
#5899=EDGE_CURVE ( 'NONE', #43723, #48553, #7445, .T. ) ;
#5900=DIRECTION ( 'NONE',  ( 0.000000000000000000, 5.664403186863042467E-17, 1.000000000000000000 ) ) ;
#5905=DIRECTION ( 'NONE',  ( 1.000000000000000000, 0.000000000000000000, 0.000000000000000000 ) ) ;
#5907=DIRECTION ( 'NONE',  ( -1.000000000000000000, 0.000000000000000000, 1.860490536778032451E-50 ) ) ;
#5912=ORIENTED_EDGE ( 'NONE', *, *, #26645, .T. ) ;
#5916=CARTESIAN_POINT ( 'NONE',  ( 360.0000000000002274, 166.6568542494923406, 341.6568542494921417 ) ) ;
#5917=AXIS2_PLACEMENT_3D ( 'NONE', #32974, #48558, #29109 ) ;
#5921=EDGE_LOOP ( 'NONE', ( #46869, #44703, #35440, #46941 ) ) ;
#5924=VECTOR ( 'NONE', #38415, 1000.000000000000000 ) ;
#5935=CIRCLE ( 'NONE', #1009, 2.000000000000001776 ) ;
#5937=DIRECTION ( 'NONE',  ( 0.000000000000000000, -2.969158215481698263E-48, 1.000000000000000000 ) ) ;
#5948=ORIENTED_EDGE ( 'NONE', *, *, #6745, .T. ) ;
#5949=ORIENTED_EDGE ( 'NONE', *, *, #2208, .F. ) ;
#5954=DIRECTION ( 'NONE',  ( 0.000000000000000000, 0.000000000000000000, 1.000000000000000000 ) ) ;
#5965=PLANE ( 'NONE',  #33978 ) ;
#5966=VECTOR ( 'NONE', #15694, 1000.000000000000000 ) ;
#5968=ORIENTED_EDGE ( 'NONE', *, *, #49942, .F. ) ;
#5972=CARTESIAN_POINT ( 'NONE',  ( 168.9999999999999716, 6.000000000000060396, -340.0000000000001137 ) ) ;
#5975=AXIS2_PLACEMENT_3D ( 'NONE', #19675, #31494, #50674 ) ;
#5980=EDGE_LOOP ( 'NONE', ( #45782, #15733, #28671, #12013 ) ) ;
#5981=DIRECTION ( 'NONE',  ( -1.000000000000000000, 0.000000000000000000, -7.793956916774525800E-48 ) ) ;
#5982=CARTESIAN_POINT ( 'NONE',  ( 360.0000000000001137, 181.0000000000000284, 349.9999999999998295 ) ) ;
#5988=CARTESIAN_POINT ( 'NONE',  ( 357.9999999999999432, -165.0000000000001137, -106.0000000000001990 ) ) ;
#5990=EDGE_LOOP ( 'NONE', ( #39418, #17995, #11209, #40774 ) ) ;
#6002=ORIENTED_EDGE ( 'NONE', *, *, #22415, .T. ) ;
#6003=VECTOR ( 'NONE', #31881, 1000.000000000000000 ) ;
#6005=CARTESIAN_POINT ( 'NONE',  ( 350.0000000000000000, -175.0000000000000000, 349.9999999999998295 ) ) ;
#6006=AXIS2_PLACEMENT_3D ( 'NONE', #6408, #26919, #22309 ) ;
#6015=VERTEX_POINT ( 'NONE', #22823 ) ;
#6019=DIRECTION ( 'NONE',  ( 0.000000000000000000, -3.186989995019654210E-49, -1.000000000000000000 ) ) ;
#6020=VECTOR ( 'NONE', #23765, 1000.000000000000000 ) ;
#6024=EDGE_CURVE ( 'NONE', #43206, #27540, #39416, .T. ) ;
#6028=CARTESIAN_POINT ( 'NONE',  ( 183.0000000000000000, -93.49999999999998579, -350.0000000000001705 ) ) ;
#6029=DIRECTION ( 'NONE',  ( -2.958228394578793832E-31, 0.000000000000000000, -1.000000000000000000 ) ) ;
#6032=DIRECTION ( 'NONE',  ( -1.000000000000000000, 0.000000000000000000, 0.000000000000000000 ) ) ;
#6038=AXIS2_PLACEMENT_3D ( 'NONE', #17098, #36370, #21699 ) ;
#6049=CYLINDRICAL_SURFACE ( 'NONE', #46991, 2.000000000000001776 ) ;
#6051=EDGE_CURVE ( 'NONE', #42585, #27971, #31045, .T. ) ;
#6055=LINE ( 'NONE', #21702, #5793 ) ;
#6056=UNCERTAINTY_MEASURE_WITH_UNIT (LENGTH_MEASURE( 1.000000000000000082E-05 ), #3542, 'distance_accuracy_value', 'NONE');
#6058=EDGE_CURVE ( 'NONE', #4113, #26133, #12537, .T. ) ;
#6065=CARTESIAN_POINT ( 'NONE',  ( 169.0000000000000000, -174.9999999999999716, -111.0000000000001563 ) ) ;
#6069=DIRECTION ( 'NONE',  ( -1.586032892321652236E-16, -1.000000000000000000, -2.288264760618012091E-48 ) ) ;
#6070=DIRECTION ( 'NONE',  ( 0.000000000000000000, 1.000000000000000000, 0.000000000000000000 ) ) ;
#6073=CARTESIAN_POINT ( 'NONE',  ( 168.9999999999999716, -174.9999999999999716, -344.0000000000001137 ) ) ;
#6077=ORIENTED_EDGE ( 'NONE', *, *, #10976, .T. ) ;
#6088=DIRECTION ( 'NONE',  ( -0.000000000000000000, -1.000000000000000000, -0.000000000000000000 ) ) ;
#6092=LINE ( 'NONE', #28447, #34667 ) ;
#6100=CARTESIAN_POINT ( 'NONE',  ( 181.0000000000003411, 165.0000000000000000, 359.9999999999997726 ) ) ;
#6101=DIRECTION ( 'NONE',  ( 1.000000000000000000, 0.000000000000000000, 0.000000000000000000 ) ) ;
#6102=ORIENTED_EDGE ( 'NONE', *, *, #5184, .T. ) ;
#6113=CARTESIAN_POINT ( 'NONE',  ( 168.9999999999999716, -272.5000000000000000, -114.9999999999999147 ) ) ;
#6116=ORIENTED_EDGE ( 'NONE', *, *, #4179, .F. ) ;
#6118=CARTESIAN_POINT ( 'NONE',  ( 356.0000000000001137, 165.0000000000000000, 339.9999999999998295 ) ) ;
#6120=EDGE_CURVE ( 'NONE', #32197, #20771, #1264, .T. ) ;
#6124=ORIENTED_EDGE ( 'NONE', *, *, #44962, .F. ) ;
#6128=EDGE_CURVE ( 'NONE', #33080, #35109, #33318, .T. ) ;
#6135=ORIENTED_EDGE ( 'NONE', *, *, #19751, .F. ) ;
#6138=ORIENTED_EDGE ( 'NONE', *, *, #15141, .F. ) ;
#6140=EDGE_LOOP ( 'NONE', ( #49167, #19830, #37309, #22354 ) ) ;
#6153=LINE ( 'NONE', #13336, #13616 ) ;
#6156=AXIS2_PLACEMENT_3D ( 'NONE', #20350, #36536, #24721 ) ;
#6160=CARTESIAN_POINT ( 'NONE',  ( 356.0000000000001137, 185.0000000000000284, 349.9999999999998295 ) ) ;
#6162=DIRECTION ( 'NONE',  ( -0.000000000000000000, -1.000000000000000000, -0.000000000000000000 ) ) ;
#6164=CARTESIAN_POINT ( 'NONE',  ( 168.9999999999999716, -256.4999999999999432, -339.9999999999998863 ) ) ;
#6169=DIRECTION ( 'NONE',  ( 0.000000000000000000, 1.000000000000000000, 7.004339610132985974E-48 ) ) ;
#6171=AXIS2_PLACEMENT_3D ( 'NONE', #43471, #16791, #47542 ) ;
#6176=VECTOR ( 'NONE', #12500, 1000.000000000000000 ) ;
#6190=AXIS2_PLACEMENT_3D ( 'NONE', #1242, #16884, #48377 ) ;
#6191=DIRECTION ( 'NONE',  ( -1.586032892321652236E-16, -1.000000000000000000, -6.853681917100419162E-49 ) ) ;
#6197=ORIENTED_EDGE ( 'NONE', *, *, #16528, .F. ) ;
#6199=VECTOR ( 'NONE', #33678, 1000.000000000000000 ) ;
#6205=ORIENTED_EDGE ( 'NONE', *, *, #7305, .T. ) ;
#6207=EDGE_CURVE ( 'NONE', #8852, #13504, #37183, .T. ) ;
#6215=VECTOR ( 'NONE', #33902, 1000.000000000000000 ) ;
#6225=LINE ( 'NONE', #9311, #42226 ) ;
#6226=VERTEX_POINT ( 'NONE', #36939 ) ;
#6238=CARTESIAN_POINT ( 'NONE',  ( 168.9999999999999716, 165.0000000000000000, 339.9999999999997726 ) ) ;
#6239=EDGE_CURVE ( 'NONE', #47737, #21998, #46713, .T. ) ;
#6244=PLANE ( 'NONE',  #7341 ) ;
#6248=DIRECTION ( 'NONE',  ( -3.172065784643302499E-16, -1.000000000000000000, 2.537652627714642000E-15 ) ) ;
#6250=AXIS2_PLACEMENT_3D ( 'NONE', #50502, #27210, #16411 ) ;
#6265=EDGE_CURVE ( 'NONE', #18739, #15426, #6354, .T. ) ;
#6269=ORIENTED_EDGE ( 'NONE', *, *, #42816, .F. ) ;
#6270=CYLINDRICAL_SURFACE ( 'NONE', #31514, 2.000000000000001776 ) ;
#6273=STYLED_ITEM('',(#50747),#21989);
#6281=ORIENTED_EDGE ( 'NONE', *, *, #167, .T. ) ;
#6283=LINE ( 'NONE', #17566, #20203 ) ;
#6290=VERTEX_POINT ( 'NONE', #33820 ) ;
#6291=PLANE ( 'NONE',  #43059 ) ;
#6294=DIRECTION ( 'NONE',  ( 0.000000000000000000, 0.000000000000000000, -1.000000000000000000 ) ) ;
#6300=DIRECTION ( 'NONE',  ( 1.000000000000000000, 0.000000000000000000, 0.000000000000000000 ) ) ;
#6302=ADVANCED_FACE ( 'NONE', ( #49412 ), #37674, .F. ) ;
#6305=LINE ( 'NONE', #21945, #23718 ) ;
#6313=CARTESIAN_POINT ( 'NONE',  ( 344.0000000000000000, -167.0000000000000853, -342.0000000000002842 ) ) ;
#6318=FACE_OUTER_BOUND ( 'NONE', #7397, .T. ) ;
#6327=CARTESIAN_POINT ( 'NONE',  ( 4.999999999999999112, -175.0000000000000284, -350.0000000000002274 ) ) ;
#6330=VERTEX_POINT ( 'NONE', #49900 ) ;
#6334=ORIENTED_EDGE ( 'NONE', *, *, #4346, .F. ) ;
#6335=LINE ( 'NONE', #29936, #13914 ) ;
#6339=LINE ( 'NONE', #26084, #13505 ) ;
#6346=CARTESIAN_POINT ( 'NONE',  ( 181.0000000000000000, -77.49999999999997158, -340.0000000000001137 ) ) ;
#6353=CARTESIAN_POINT ( 'NONE',  ( 350.0000000000001137, 185.0000000000000284, 355.9999999999997726 ) ) ;
#6354=LINE ( 'NONE', #14038, #49156 ) ;
#6356=DIRECTION ( 'NONE',  ( -1.121065046350011585E-16, -0.7071067811865475727, -0.7071067811865474617 ) ) ;
#6357=ORIENTED_EDGE ( 'NONE', *, *, #47916, .T. ) ;
#6359=FACE_BOUND ( 'NONE', #46768, .T. ) ;
#6360=DIRECTION ( 'NONE',  ( 1.000000000000000000, 0.000000000000000000, 0.000000000000000000 ) ) ;
#6371=FACE_BOUND ( 'NONE', #19739, .T. ) ;
#6377=CARTESIAN_POINT ( 'NONE',  ( 181.0000000000000000, 165.0000000000000000, -344.0000000000001137 ) ) ;
#6378=CARTESIAN_POINT ( 'NONE',  ( 183.0000000000000000, -272.4999999999999432, -343.9999999999994316 ) ) ;
#6379=EDGE_CURVE ( 'NONE', #29467, #16943, #26099, .T. ) ;
#6383=AXIS2_PLACEMENT_3D ( 'NONE', #3366, #33932, #42368 ) ;
#6384=DIRECTION ( 'NONE',  ( -1.000000000000000000, 0.000000000000000000, 0.000000000000000000 ) ) ;
#6385=DIRECTION ( 'NONE',  ( -1.000000000000000000, 0.000000000000000000, 0.000000000000000000 ) ) ;
#6386=ORIENTED_EDGE ( 'NONE', *, *, #27321, .F. ) ;
#6405=ADVANCED_FACE ( 'NONE', ( #45815, #10703 ), #14297, .F. ) ;
#6407=DIRECTION ( 'NONE',  ( 1.000000000000000000, 0.000000000000000000, 0.000000000000000000 ) ) ;
#6408=CARTESIAN_POINT ( 'NONE',  ( 349.9999999999999432, -168.9999999999999432, 343.9999999999997726 ) ) ;
#6416=DIRECTION ( 'NONE',  ( 0.000000000000000000, 0.000000000000000000, -1.000000000000000000 ) ) ;
#6425=CARTESIAN_POINT ( 'NONE',  ( 0.000000000000000000, 165.0000000000000000, 343.9999999999997726 ) ) ;
#6433=DIRECTION ( 'NONE',  ( -1.586032892321652236E-16, -1.000000000000000000, -6.853681917100419162E-49 ) ) ;
#6436=DIRECTION ( 'NONE',  ( -1.000000000000000000, 0.000000000000000000, -1.612977847700450206E-50 ) ) ;
#6444=CARTESIAN_POINT ( 'NONE',  ( 358.0000000000000568, 165.0000000000000000, -94.00000000000019895 ) ) ;
#6447=ORIENTED_EDGE ( 'NONE', *, *, #36855, .T. ) ;
#6449=CIRCLE ( 'NONE', #23674, 2.000000000000001776 ) ;
#6452=CARTESIAN_POINT ( 'NONE',  ( 339.9999999999998863, -169.0000000000001137, -349.9999999999998863 ) ) ;
#6457=DIRECTION ( 'NONE',  ( -7.793956916774525800E-48, 0.000000000000000000, 1.000000000000000000 ) ) ;
#6458=CLOSED_SHELL ( 'NONE', ( #38372, #1640, #27091, #34780, #41572, #37608, #26824, #41481, #37992, #39997, #2994, #13611, #15526, #36867, #39329, #19306, #24177, #43835 ) ) ;
#6460=LINE ( 'NONE', #29064, #29924 ) ;
#6464=LINE ( 'NONE', #41621, #5576 ) ;
#6467=EDGE_CURVE ( 'NONE', #34142, #43723, #35605, .T. ) ;
#6469=LINE ( 'NONE', #22125, #18389 ) ;
#6482=DIRECTION ( 'NONE',  ( -0.000000000000000000, -1.000000000000000000, -0.000000000000000000 ) ) ;
#6488=AXIS2_PLACEMENT_3D ( 'NONE', #44453, #631, #32680 ) ;
#6491=ORIENTED_EDGE ( 'NONE', *, *, #6700, .T. ) ;
#6493=DIRECTION ( 'NONE',  ( 1.000000000000000000, 0.000000000000000000, 0.000000000000000000 ) ) ;
#6499=LINE ( 'NONE', #22157, #23032 ) ;
#6502=ORIENTED_EDGE ( 'NONE', *, *, #21794, .T. ) ;
#6508=VERTEX_POINT ( 'NONE', #27380 ) ;
#6514=EDGE_LOOP ( 'NONE', ( #6875, #26279, #37179, #8431 ) ) ;
#6521=LINE ( 'NONE', #25779, #30742 ) ;
#6522=( LENGTH_UNIT ( ) NAMED_UNIT ( * ) SI_UNIT ( .MILLI., .METRE. ) );
#6532=PLANE ( 'NONE',  #9395 ) ;
#6535=CIRCLE ( 'NONE', #8198, 4.000000000000003553 ) ;
#6544=LINE ( 'NONE', #41440, #1080 ) ;
#6545=LINE ( 'NONE', #45758, #28590 ) ;
#6550=DIRECTION ( 'NONE',  ( 0.000000000000000000, 1.000000000000000000, 6.123233995736766036E-17 ) ) ;
#6558=ORIENTED_EDGE ( 'NONE', *, *, #20803, .T. ) ;
#6563=AXIS2_PLACEMENT_3D ( 'NONE', #30667, #27319, #36045 ) ;
#6567=EDGE_LOOP ( 'NONE', ( #3903, #8809, #39078, #40618 ) ) ;
#6568=ORIENTED_EDGE ( 'NONE', *, *, #48132, .F. ) ;
#6578=CARTESIAN_POINT ( 'NONE',  ( 168.9999999999999716, 165.0000000000000000, -342.0000000000001137 ) ) ;
#6579=DIRECTION ( 'NONE',  ( -1.942330104924128867E-32, 0.000000000000000000, -1.000000000000000000 ) ) ;
#6582=EDGE_LOOP ( 'NONE', ( #11865, #7339, #43736, #19141, #27309, #25903, #22286, #4232 ) ) ;
#6588=LINE ( 'NONE', #30448, #5924 ) ;
#6590=CARTESIAN_POINT ( 'NONE',  ( 358.3431457505077447, 185.0000000000000284, 359.9999999999998863 ) ) ;
#6592=EDGE_LOOP ( 'NONE', ( #6077, #260, #40368, #26391, #36192, #19814, #23537, #23326 ) ) ;
#6595=LINE ( 'NONE', #34564, #14160 ) ;
#6601=ORIENTED_EDGE ( 'NONE', *, *, #26431, .T. ) ;
#6619=ORIENTED_EDGE ( 'NONE', *, *, #40725, .T. ) ;
#6620=CARTESIAN_POINT ( 'NONE',  ( 350.0000000000000000, 169.0000000000000000, -356.0000000000002274 ) ) ;
#6621=EDGE_LOOP ( 'NONE', ( #40075, #27301, #48862, #10561 ) ) ;
#6633=CARTESIAN_POINT ( 'NONE',  ( 166.9999999999999716, -164.9999999999999432, 343.9999999999998863 ) ) ;
#6638=ORIENTED_EDGE ( 'NONE', *, *, #9099, .F. ) ;
#6640=EDGE_LOOP ( 'NONE', ( #42790, #15204, #31412, #26288, #39097, #23130, #39834, #22033 ) ) ;
#6644=AXIS2_PLACEMENT_3D ( 'NONE', #46015, #6550, #17841 ) ;
#6653=LINE ( 'NONE', #6160, #15236 ) ;
#6656=VERTEX_POINT ( 'NONE', #4774 ) ;
#6657=LINE ( 'NONE', #46123, #33752 ) ;
#6663=VECTOR ( 'NONE', #40743, 1000.000000000000000 ) ;
#6666=ORIENTED_EDGE ( 'NONE', *, *, #9875, .F. ) ;
#6679=FACE_OUTER_BOUND ( 'NONE', #45452, .T. ) ;
#6682=CARTESIAN_POINT ( 'NONE',  ( 181.0000000000000284, -174.9999999999999716, -113.0000000000001563 ) ) ;
#6687=ORIENTED_EDGE ( 'NONE', *, *, #23028, .F. ) ;
#6690=CARTESIAN_POINT ( 'NONE',  ( 183.0000000000000000, -5.999999999999950262, 339.9999999999998295 ) ) ;
#6700=EDGE_CURVE ( 'NONE', #13420, #17053, #10899, .T. ) ;
#6705=FACE_OUTER_BOUND ( 'NONE', #42021, .T. ) ;
#6707=CIRCLE ( 'NONE', #31311, 4.000000000000003553 ) ;
#6709=EDGE_LOOP ( 'NONE', ( #15716, #4983, #40703, #34939 ) ) ;
#6711=DIRECTION ( 'NONE',  ( 1.000000000000000000, 0.000000000000000000, -1.860490536778032451E-50 ) ) ;
#6728=LINE ( 'NONE', #7240, #8606 ) ;
#6733=FACE_OUTER_BOUND ( 'NONE', #4106, .T. ) ;
#6740=VECTOR ( 'NONE', #22946, 1000.000000000000000 ) ;
#6745=EDGE_CURVE ( 'NONE', #20029, #40480, #18895, .T. ) ;
#6748=ORIENTED_EDGE ( 'NONE', *, *, #36709, .F. ) ;
#6751=DIRECTION ( 'NONE',  ( 0.000000000000000000, 1.000000000000000000, 0.000000000000000000 ) ) ;
#6754=ORIENTED_EDGE ( 'NONE', *, *, #27997, .T. ) ;
#6759=ORIENTED_EDGE ( 'NONE', *, *, #25597, .T. ) ;
#6785=LINE ( 'NONE', #50082, #41688 ) ;
#6788=ORIENTED_EDGE ( 'NONE', *, *, #43538, .F. ) ;
#6792=PRODUCT_DEFINITION ( 'UNKNOWN', '', #48740, #20094 ) ;
#6806=CYLINDRICAL_SURFACE ( 'NONE', #38800, 4.000000000000003553 ) ;
#6810=ORIENTED_EDGE ( 'NONE', *, *, #3337, .F. ) ;
#6813=CARTESIAN_POINT ( 'NONE',  ( 167.0000000000000000, -168.9999999999999432, -115.0000000000001847 ) ) ;
#6815=ADVANCED_FACE ( 'NONE', ( #27059 ), #35295, .F. ) ;
#6819=DIRECTION ( 'NONE',  ( -0.000000000000000000, -1.000000000000000000, 2.537652627714643577E-15 ) ) ;
#6825=PLANE ( 'NONE',  #20068 ) ;
#6826=EDGE_CURVE ( 'NONE', #5803, #1861, #23479, .T. ) ;
#6836=ORIENTED_EDGE ( 'NONE', *, *, #41640, .F. ) ;
#6839=CYLINDRICAL_SURFACE ( 'NONE', #36611, 4.000000000000003553 ) ;
#6843=ORIENTED_EDGE ( 'NONE', *, *, #34749, .T. ) ;
#6845=DIRECTION ( 'NONE',  ( 0.000000000000000000, 0.000000000000000000, -1.000000000000000000 ) ) ;
#6849=VECTOR ( 'NONE', #13860, 1000.000000000000000 ) ;
#6851=ORIENTED_EDGE ( 'NONE', *, *, #36811, .T. ) ;
#6858=DIRECTION ( 'NONE',  ( 0.000000000000000000, -1.000000000000000000, 2.537652627714642000E-15 ) ) ;
#6861=CARTESIAN_POINT ( 'NONE',  ( 183.0000000000000000, -5.999999999999950262, 339.9999999999998295 ) ) ;
#6862=DIRECTION ( 'NONE',  ( 0.000000000000000000, 0.000000000000000000, 1.000000000000000000 ) ) ;
#6863=EDGE_CURVE ( 'NONE', #22911, #11669, #42953, .T. ) ;
#6873=VERTEX_POINT ( 'NONE', #39139 ) ;
#6875=ORIENTED_EDGE ( 'NONE', *, *, #29069, .F. ) ;
#6877=CARTESIAN_POINT ( 'NONE',  ( 358.3431457505076878, 165.0000000000000284, 339.9999999999998295 ) ) ;
#6882=VECTOR ( 'NONE', #44035, 1000.000000000000000 ) ;
#6887=VERTEX_POINT ( 'NONE', #46265 ) ;
#6889=DIRECTION ( 'NONE',  ( 0.000000000000000000, 1.000000000000000000, -2.537652627714642000E-15 ) ) ;
#6893=ORIENTED_EDGE ( 'NONE', *, *, #26918, .T. ) ;
#6894=CARTESIAN_POINT ( 'NONE',  ( 0.000000000000000000, -180.9999999999999716, -344.0000000000001705 ) ) ;
#6908=DIRECTION ( 'NONE',  ( 0.000000000000000000, 0.000000000000000000, -1.000000000000000000 ) ) ;
#6909=CARTESIAN_POINT ( 'NONE',  ( 341.6568542494922553, -165.0000000000001137, -340.0000000000002842 ) ) ;
#6914=ORIENTED_EDGE ( 'NONE', *, *, #10808, .F. ) ;
#6918=FACE_OUTER_BOUND ( 'NONE', #9421, .T. ) ;
#6922=VECTOR ( 'NONE', #22891, 1000.000000000000000 ) ;
#6923=CARTESIAN_POINT ( 'NONE',  ( 340.0000000000000568, 169.0000000000000000, 349.9999999999998295 ) ) ;
#6927=CARTESIAN_POINT ( 'NONE',  ( 168.9999999999999716, -164.9999999999999432, -344.0000000000001137 ) ) ;
#6931=ORIENTED_EDGE ( 'NONE', *, *, #4477, .T. ) ;
#6933=ORIENTED_EDGE ( 'NONE', *, *, #32149, .F. ) ;
#6937=VERTEX_POINT ( 'NONE', #12177 ) ;
#6939=DIRECTION ( 'NONE',  ( 0.000000000000000000, 0.000000000000000000, -1.000000000000000000 ) ) ;
#6944=ORIENTED_EDGE ( 'NONE', *, *, #49981, .F. ) ;
#6945=DIRECTION ( 'NONE',  ( -0.000000000000000000, -1.000000000000000000, 2.537652627714643577E-15 ) ) ;
#6950=LINE ( 'NONE', #37275, #37422 ) ;
#6952=ORIENTED_EDGE ( 'NONE', *, *, #38542, .F. ) ;
#6955=CARTESIAN_POINT ( 'NONE',  ( 344.0000000000000000, -165.0000000000001137, -340.0000000000003411 ) ) ;
#6958=ADVANCED_FACE ( 'NONE', ( #34519 ), #19094, .T. ) ;
#6960=VERTEX_POINT ( 'NONE', #1644 ) ;
#6970=ORIENTED_EDGE ( 'NONE', *, *, #24303, .F. ) ;
#6976=LINE ( 'NONE', #25985, #39781 ) ;
#6979=CARTESIAN_POINT ( 'NONE',  ( 181.0000000000000000, 165.0000000000000000, -360.0000000000002274 ) ) ;
#6985=CARTESIAN_POINT ( 'NONE',  ( 344.0000000000000000, 174.9999999999996589, -340.0000000000002842 ) ) ;
#6989=VECTOR ( 'NONE', #33249, 1000.000000000000000 ) ;
#6990=VECTOR ( 'NONE', #17626, 1000.000000000000000 ) ;
#7005=ORIENTED_EDGE ( 'NONE', *, *, #25734, .T. ) ;
#7017=CARTESIAN_POINT ( 'NONE',  ( 342.0000000000000568, 169.0000000000000000, 343.9999999999998863 ) ) ;
#7018=VECTOR ( 'NONE', #42228, 1000.000000000000000 ) ;
#7019=ORIENTED_EDGE ( 'NONE', *, *, #26508, .F. ) ;
#7023=CIRCLE ( 'NONE', #2084, 4.000000000000003553 ) ;
#7025=EDGE_CURVE ( 'NONE', #25245, #16715, #4973, .T. ) ;
#7027=EDGE_CURVE ( 'NONE', #24412, #17736, #1397, .T. ) ;
#7029=VECTOR ( 'NONE', #43294, 1000.000000000000000 ) ;
#7032=MECHANICAL_DESIGN_GEOMETRIC_PRESENTATION_REPRESENTATION('',(#14427),#17686);
#7042=DIRECTION ( 'NONE',  ( 0.000000000000000000, 0.000000000000000000, -1.000000000000000000 ) ) ;
#7043=ORIENTED_EDGE ( 'NONE', *, *, #3490, .T. ) ;
#7049=ORIENTED_EDGE ( 'NONE', *, *, #42164, .F. ) ;
#7065=AXIS2_PLACEMENT_3D ( 'NONE', #37030, #21087, #9547 ) ;
#7070=EDGE_LOOP ( 'NONE', ( #30297, #22034, #27610, #48993 ) ) ;
#7073=CARTESIAN_POINT ( 'NONE',  ( 342.0000000000000000, 175.0000000000000284, -94.00000000000019895 ) ) ;
#7075=CARTESIAN_POINT ( 'NONE',  ( 181.0000000000000284, -174.9999999999999716, -111.0000000000001563 ) ) ;
#7078=EDGE_CURVE ( 'NONE', #3283, #35970, #43964, .T. ) ;
#7087=CARTESIAN_POINT ( 'NONE',  ( 168.9999999999999716, -5.999999999999950262, -340.0000000000001137 ) ) ;
#7088=EDGE_LOOP ( 'NONE', ( #18910, #15695, #45340, #12088 ) ) ;
#7096=DIRECTION ( 'NONE',  ( 0.000000000000000000, 1.000000000000000000, 0.000000000000000000 ) ) ;
#7102=VECTOR ( 'NONE', #41042, 1000.000000000000000 ) ;
#7111=AXIS2_PLACEMENT_3D ( 'NONE', #17910, #49435, #25892 ) ;
#7115=VERTEX_POINT ( 'NONE', #9832 ) ;
#7122=ORIENTED_EDGE ( 'NONE', *, *, #24961, .T. ) ;
#7132=VERTEX_POINT ( 'NONE', #45704 ) ;
#7138=ORIENTED_EDGE ( 'NONE', *, *, #11475, .F. ) ;
#7143=CARTESIAN_POINT ( 'NONE',  ( 359.9999999999999432, -177.9999999999999147, -353.0000000000001137 ) ) ;
#7145=LINE ( 'NONE', #26129, #45450 ) ;
#7146=CARTESIAN_POINT ( 'NONE',  ( 356.0000000000001137, 169.0000000000000000, 349.9999999999998295 ) ) ;
#7150=LINE ( 'NONE', #220, #42524 ) ;
#7152=ORIENTED_EDGE ( 'NONE', *, *, #42796, .T. ) ;
#7153=ORIENTED_EDGE ( 'NONE', *, *, #14278, .F. ) ;
#7158=EDGE_CURVE ( 'NONE', #9291, #50718, #38060, .T. ) ;
#7173=EDGE_CURVE ( 'NONE', #24207, #33697, #45959, .T. ) ;
#7208=DIRECTION ( 'NONE',  ( 0.000000000000000000, -1.000000000000000000, 0.000000000000000000 ) ) ;
#7210=DIRECTION ( 'NONE',  ( 0.000000000000000000, 1.000000000000000000, 1.544785076050074834E-48 ) ) ;
#7211=DIRECTION ( 'NONE',  ( 0.000000000000000000, -0.000000000000000000, 1.000000000000000000 ) ) ;
#7212=ORIENTED_EDGE ( 'NONE', *, *, #9729, .T. ) ;
#7215=CARTESIAN_POINT ( 'NONE',  ( 341.9999999999999432, -181.0000000000001705, -356.0000000000003411 ) ) ;
#7217=ORIENTED_EDGE ( 'NONE', *, *, #1371, .F. ) ;
#7219=CARTESIAN_POINT ( 'NONE',  ( 181.0000000000000284, -174.9999999999999716, -99.00000000000014211 ) ) ;
#7227=VERTEX_POINT ( 'NONE', #3902 ) ;
#7230=DIRECTION ( 'NONE',  ( -9.711650524620651178E-33, 1.223873602809432483E-48, -1.000000000000000000 ) ) ;
#7231=LINE ( 'NONE', #39497, #27709 ) ;
#7232=CARTESIAN_POINT ( 'NONE',  ( 342.0000000000000568, 181.0000000000000568, 355.9999999999998295 ) ) ;
#7233=AXIS2_PLACEMENT_3D ( 'NONE', #50019, #14927, #47382 ) ;
#7235=DIRECTION ( 'NONE',  ( 1.000000000000000000, 0.000000000000000000, -4.758098676964956461E-16 ) ) ;
#7237=ORIENTED_EDGE ( 'NONE', *, *, #8244, .T. ) ;
#7240=CARTESIAN_POINT ( 'NONE',  ( -5.000000000000000000, -184.7999999999999545, -359.8000000000002387 ) ) ;
#7241=DIRECTION ( 'NONE',  ( 2.958228394578794708E-31, 0.000000000000000000, -1.000000000000000000 ) ) ;
#7242=EDGE_LOOP ( 'NONE', ( #23431, #35818, #42706, #49198 ) ) ;
#7243=FACE_BOUND ( 'NONE', #35835, .T. ) ;
#7248=CARTESIAN_POINT ( 'NONE',  ( 344.0000000000000568, 165.0000000000000000, 339.9999999999998295 ) ) ;
#7253=DIRECTION ( 'NONE',  ( 0.000000000000000000, 2.969158215481698263E-48, -1.000000000000000000 ) ) ;
#7262=CIRCLE ( 'NONE', #37614, 2.000000000000001776 ) ;
#7264=ORIENTED_EDGE ( 'NONE', *, *, #22227, .F. ) ;
#7266=LINE ( 'NONE', #22913, #46353 ) ;
#7274=CARTESIAN_POINT ( 'NONE',  ( 168.9999999999998863, -164.9999999999999432, 357.9999999999998863 ) ) ;
#7279=CARTESIAN_POINT ( 'NONE',  ( 350.0000000000000000, -174.9999999999999716, 349.9999999999998295 ) ) ;
#7283=CARTESIAN_POINT ( 'NONE',  ( 165.0000000000000284, 175.0000000000000284, 355.9999999999998863 ) ) ;
#7284=ORIENTED_EDGE ( 'NONE', *, *, #27754, .T. ) ;
#7300=LINE ( 'NONE', #11403, #6740 ) ;
#7303=AXIS2_PLACEMENT_3D ( 'NONE', #29237, #17918, #9984 ) ;
#7305=EDGE_CURVE ( 'NONE', #11492, #35493, #948, .T. ) ;
#7307=PLANE ( 'NONE',  #9822 ) ;
#7314=DIRECTION ( 'NONE',  ( 0.000000000000000000, 1.000000000000000000, 0.000000000000000000 ) ) ;
#7320=ORIENTED_EDGE ( 'NONE', *, *, #37487, .T. ) ;
#7328=CARTESIAN_POINT ( 'NONE',  ( 350.0000000000000000, -184.9999999999999716, -340.0000000000001705 ) ) ;
#7329=ORIENTED_EDGE ( 'NONE', *, *, #47497, .F. ) ;
#7333=EDGE_CURVE ( 'NONE', #22392, #41767, #40279, .T. ) ;
#7338=EDGE_CURVE ( 'NONE', #27092, #43206, #30868, .T. ) ;
#7339=ORIENTED_EDGE ( 'NONE', *, *, #15158, .F. ) ;
#7341=AXIS2_PLACEMENT_3D ( 'NONE', #22381, #37317, #21894 ) ;
#7342=FACE_OUTER_BOUND ( 'NONE', #47818, .T. ) ;
#7343=CARTESIAN_POINT ( 'NONE',  ( 339.9999999999998863, -180.9999999999999716, 359.9999999999998295 ) ) ;
#7345=ORIENTED_EDGE ( 'NONE', *, *, #41068, .T. ) ;
#7346=ORIENTED_EDGE ( 'NONE', *, *, #8284, .F. ) ;
#7347=CARTESIAN_POINT ( 'NONE',  ( 360.0000000000000000, 175.0000000000000284, -106.0000000000001990 ) ) ;
#7354=ORIENTED_EDGE ( 'NONE', *, *, #24488, .F. ) ;
#7362=DIRECTION ( 'NONE',  ( -1.000000000000000000, 0.000000000000000000, 0.000000000000000000 ) ) ;
#7367=ADVANCED_FACE ( 'NONE', ( #44151 ), #35986, .F. ) ;
#7368=EDGE_CURVE ( 'NONE', #43146, #9965, #32377, .T. ) ;
#7369=CARTESIAN_POINT ( 'NONE',  ( 169.0000000000000000, -174.9999999999999716, -111.0000000000001563 ) ) ;
#7372=ADVANCED_FACE ( 'NONE', ( #47975 ), #32123, .F. ) ;
#7378=VECTOR ( 'NONE', #38944, 1000.000000000000000 ) ;
#7381=DIRECTION ( 'NONE',  ( 0.000000000000000000, -1.000000000000000000, -0.000000000000000000 ) ) ;
#7384=DIRECTION ( 'NONE',  ( 6.203854594147707562E-25, -2.067951531382569187E-25, 1.000000000000000000 ) ) ;
#7396=AXIS2_PLACEMENT_3D ( 'NONE', #11302, #34406, #12068 ) ;
#7397=EDGE_LOOP ( 'NONE', ( #11686, #37902, #32542, #23820 ) ) ;
#7403=EDGE_LOOP ( 'NONE', ( #36373, #31760, #22102, #48163 ) ) ;
#7405=FACE_OUTER_BOUND ( 'NONE', #40165, .T. ) ;
#7409=EDGE_CURVE ( 'NONE', #17284, #3318, #45078, .T. ) ;
#7421=AXIS2_PLACEMENT_3D ( 'NONE', #39397, #12674, #28082 ) ;
#7424=AXIS2_PLACEMENT_3D ( 'NONE', #46404, #42826, #15902 ) ;
#7428=DIRECTION ( 'NONE',  ( -9.711650524620651178E-33, 1.223873602809432483E-48, -1.000000000000000000 ) ) ;
#7429=AXIS2_PLACEMENT_3D ( 'NONE', #37968, #25905, #26394 ) ;
#7445=LINE ( 'NONE', #22315, #13170 ) ;
#7447=VERTEX_POINT ( 'NONE', #50160 ) ;
#7451=VERTEX_POINT ( 'NONE', #18905 ) ;
#7461=DIRECTION ( 'NONE',  ( 0.000000000000000000, 5.664403186863042467E-17, 1.000000000000000000 ) ) ;
#7463=LINE ( 'NONE', #15407, #48287 ) ;
#7467=VECTOR ( 'NONE', #7831, 1000.000000000000000 ) ;
#7470=DIRECTION ( 'NONE',  ( 1.132880637372608740E-16, 4.718402560806925739E-50, 1.000000000000000000 ) ) ;
#7473=EDGE_CURVE ( 'NONE', #37912, #1398, #26873, .T. ) ;
#7481=CARTESIAN_POINT ( 'NONE',  ( 181.0000000000000284, -174.9999999999999716, -99.00000000000014211 ) ) ;
#7482=ADVANCED_FACE ( 'NONE', ( #25867 ), #10214, .F. ) ;
#7483=CARTESIAN_POINT ( 'NONE',  ( 342.8284271247462129, -167.0000000000000000, 341.9999999999998295 ) ) ;
#7501=DIRECTION ( 'NONE',  ( 0.000000000000000000, 1.000000000000000000, 0.000000000000000000 ) ) ;
#7512=ORIENTED_EDGE ( 'NONE', *, *, #21317, .F. ) ;
#7515=CARTESIAN_POINT ( 'NONE',  ( 339.9999999999999432, 169.0000000000000000, -358.0000000000002274 ) ) ;
#7520=PLANE ( 'NONE',  #34057 ) ;
#7535=ORIENTED_EDGE ( 'NONE', *, *, #46197, .F. ) ;
#7537=AXIS2_PLACEMENT_3D ( 'NONE', #29972, #29712, #45327 ) ;
#7540=VERTEX_POINT ( 'NONE', #18652 ) ;
#7543=CARTESIAN_POINT ( 'NONE',  ( 0.000000000000000000, -182.9999999999999716, -344.0000000000001705 ) ) ;
#7545=CARTESIAN_POINT ( 'NONE',  ( 344.0000000000000568, 185.0000000000000284, 359.9999999999998295 ) ) ;
#7559=VECTOR ( 'NONE', #32092, 1000.000000000000114 ) ;
#7560=CARTESIAN_POINT ( 'NONE',  ( 181.0000000000000568, 165.0000000000000000, 343.9999999999998863 ) ) ;
#7571=EDGE_CURVE ( 'NONE', #49828, #5729, #11234, .T. ) ;
#7573=FACE_OUTER_BOUND ( 'NONE', #50256, .T. ) ;
#7590=VECTOR ( 'NONE', #11288, 1000.000000000000000 ) ;
#7598=EDGE_LOOP ( 'NONE', ( #41810, #32059, #27601, #5144 ) ) ;
#7605=UNCERTAINTY_MEASURE_WITH_UNIT (LENGTH_MEASURE( 1.000000000000000082E-05 ), #22635, 'distance_accuracy_value', 'NONE');
#7616=EDGE_CURVE ( 'NONE', #38600, #25272, #38672, .T. ) ;
#7624=EDGE_LOOP ( 'NONE', ( #37751, #10665, #43068, #18772 ) ) ;
#7628=EDGE_CURVE ( 'NONE', #39919, #18651, #45177, .T. ) ;
#7630=MECHANICAL_DESIGN_GEOMETRIC_PRESENTATION_REPRESENTATION('',(#14986),#49363);
#7631=EDGE_CURVE ( 'NONE', #22898, #7540, #16090, .T. ) ;
#7632=ORIENTED_EDGE ( 'NONE', *, *, #45653, .T. ) ;
#7639=FACE_OUTER_BOUND ( 'NONE', #15679, .T. ) ;
#7645=PLANE ( 'NONE',  #19714 ) ;
#7648=DIRECTION ( 'NONE',  ( 0.000000000000000000, -1.000000000000000000, -3.186989995019654210E-49 ) ) ;
#7654=DIRECTION ( 'NONE',  ( 0.000000000000000000, 1.000000000000000000, 0.000000000000000000 ) ) ;
#7658=DIRECTION ( 'NONE',  ( 0.000000000000000000, 0.000000000000000000, 1.000000000000000000 ) ) ;
#7660=ORIENTED_EDGE ( 'NONE', *, *, #22451, .T. ) ;
#7665=CIRCLE ( 'NONE', #14194, 2.000000000000001776 ) ;
#7666=DIRECTION ( 'NONE',  ( 0.000000000000000000, 1.000000000000000000, 0.000000000000000000 ) ) ;
#7670=DIRECTION ( 'NONE',  ( 0.000000000000000000, 0.000000000000000000, 1.000000000000000000 ) ) ;
#7672=DIRECTION ( 'NONE',  ( -3.172065784643302499E-16, -1.000000000000000000, 2.537652627714642000E-15 ) ) ;
#7707=DIRECTION ( 'NONE',  ( -0.000000000000000000, -1.000000000000000000, 2.537652627714643577E-15 ) ) ;
#7708=VERTEX_POINT ( 'NONE', #46582 ) ;
#7713=LINE ( 'NONE', #12552, #20792 ) ;
#7716=DIRECTION ( 'NONE',  ( -7.793956916774524585E-48, 0.000000000000000000, -1.000000000000000000 ) ) ;
#7719=ORIENTED_EDGE ( 'NONE', *, *, #46232, .T. ) ;
#7720=LINE ( 'NONE', #23098, #29202 ) ;
#7721=FACE_BOUND ( 'NONE', #19713, .T. ) ;
#7726=CARTESIAN_POINT ( 'NONE',  ( 181.0000000000000000, 6.000000000000060396, 339.9999999999998295 ) ) ;
#7734=CARTESIAN_POINT ( 'NONE',  ( 355.9999999999999432, 174.9999999999996589, -358.0000000000003411 ) ) ;
#7735=ORIENTED_EDGE ( 'NONE', *, *, #19924, .T. ) ;
#7738=LINE ( 'NONE', #26221, #36586 ) ;
#7743=ORIENTED_EDGE ( 'NONE', *, *, #11410, .T. ) ;
#7750=DIRECTION ( 'NONE',  ( 1.000000000000000000, 0.000000000000000000, 0.000000000000000000 ) ) ;
#7755=LINE ( 'NONE', #31362, #3179 ) ;
#7760=AXIS2_PLACEMENT_3D ( 'NONE', #19523, #42871, #3368 ) ;
#7769=DIRECTION ( 'NONE',  ( -1.612977847700450206E-50, 0.000000000000000000, 1.000000000000000000 ) ) ;
#7777=CARTESIAN_POINT ( 'NONE',  ( 340.0000000000000568, 165.0000000000000000, 355.9999999999997726 ) ) ;
#7786=ORIENTED_EDGE ( 'NONE', *, *, #1831, .F. ) ;
#7791=CARTESIAN_POINT ( 'NONE',  ( 339.9999999999998863, -168.9999999999999432, 355.9999999999997726 ) ) ;
#7793=ORIENTED_EDGE ( 'NONE', *, *, #10803, .F. ) ;
#7799=VECTOR ( 'NONE', #49846, 1000.000000000000000 ) ;
#7800=ORIENTED_EDGE ( 'NONE', *, *, #10307, .T. ) ;
#7801=ORIENTED_EDGE ( 'NONE', *, *, #18621, .T. ) ;
#7803=VECTOR ( 'NONE', #43151, 1000.000000000000000 ) ;
#7808=CYLINDRICAL_SURFACE ( 'NONE', #31373, 2.000000000000001776 ) ;
#7813=DIRECTION ( 'NONE',  ( 0.000000000000000000, 0.000000000000000000, 1.000000000000000000 ) ) ;
#7816=PLANE ( 'NONE',  #13565 ) ;
#7817=CARTESIAN_POINT ( 'NONE',  ( 164.9999999999999716, -168.9999999999999432, -350.0000000000001705 ) ) ;
#7818=VERTEX_POINT ( 'NONE', #36633 ) ;
#7831=DIRECTION ( 'NONE',  ( 6.203854594147707562E-25, -2.067951531382569187E-25, 1.000000000000000000 ) ) ;
#7840=LINE ( 'NONE', #26819, #7799 ) ;
#7845=CARTESIAN_POINT ( 'NONE',  ( 181.0000000000000284, -9.999999999999953815, -95.00000000000014211 ) ) ;
#7847=ORIENTED_EDGE ( 'NONE', *, *, #30192, .F. ) ;
#7852=AXIS2_PLACEMENT_3D ( 'NONE', #1930, #32044, #36854 ) ;
#7854=AXIS2_PLACEMENT_3D ( 'NONE', #39988, #29189, #21224 ) ;
#7855=VERTEX_POINT ( 'NONE', #15014 ) ;
#7861=ORIENTED_EDGE ( 'NONE', *, *, #41074, .F. ) ;
#7863=LINE ( 'NONE', #30960, #39723 ) ;
#7882=CARTESIAN_POINT ( 'NONE',  ( 339.9999999999999432, -181.0000000000001421, -356.0000000000003411 ) ) ;
#7883=AXIS2_PLACEMENT_3D ( 'NONE', #12041, #27181, #14866 ) ;
#7888=VERTEX_POINT ( 'NONE', #49102 ) ;
#7896=CARTESIAN_POINT ( 'NONE',  ( 344.0000000000000000, 185.0000000000000000, 359.9999999999998295 ) ) ;
#7903=ORIENTED_EDGE ( 'NONE', *, *, #32396, .F. ) ;
#7906=VERTEX_POINT ( 'NONE', #33768 ) ;
#7912=DIRECTION ( 'NONE',  ( 0.000000000000000000, -1.000000000000000000, -0.000000000000000000 ) ) ;
#7913=CARTESIAN_POINT ( 'NONE',  ( 0.000000000000000000, -184.7999999999999545, -359.8000000000002387 ) ) ;
#7916=DIRECTION ( 'NONE',  ( 2.220446049250312588E-16, 0.7071067811865475727, 0.7071067811865474617 ) ) ;
#7917=VERTEX_POINT ( 'NONE', #18095 ) ;
#7926=ORIENTED_EDGE ( 'NONE', *, *, #40299, .F. ) ;
#7927=ORIENTED_EDGE ( 'NONE', *, *, #18014, .F. ) ;
#7928=VERTEX_POINT ( 'NONE', #34266 ) ;
#7931=ORIENTED_EDGE ( 'NONE', *, *, #4239, .T. ) ;
#7938=CARTESIAN_POINT ( 'NONE',  ( 0.000000000000000000, 175.0000000000000284, 346.2500000000002274 ) ) ;
#7945=CARTESIAN_POINT ( 'NONE',  ( 339.9999999999999432, 165.0000000000000000, -356.0000000000002274 ) ) ;
#7948=FACE_OUTER_BOUND ( 'NONE', #31414, .T. ) ;
#7951=DIRECTION ( 'NONE',  ( 0.000000000000000000, -1.000000000000000000, 0.000000000000000000 ) ) ;
#7952=ORIENTED_EDGE ( 'NONE', *, *, #7628, .T. ) ;
#7960=DIRECTION ( 'NONE',  ( -1.000000000000000000, -0.000000000000000000, -0.000000000000000000 ) ) ;
#7961=ORIENTED_EDGE ( 'NONE', *, *, #6863, .T. ) ;
#7962=LINE ( 'NONE', #36171, #50231 ) ;
#7967=ORIENTED_EDGE ( 'NONE', *, *, #43412, .T. ) ;
#7974=ORIENTED_EDGE ( 'NONE', *, *, #3272, .F. ) ;
#7979=VECTOR ( 'NONE', #49252, 1000.000000000000000 ) ;
#7981=DIRECTION ( 'NONE',  ( -1.586032880504786307E-16, 1.654361225106055350E-24, -1.000000000000000000 ) ) ;
#7989=CYLINDRICAL_SURFACE ( 'NONE', #22488, 4.000000000000003553 ) ;
#7991=DIRECTION ( 'NONE',  ( -1.000000000000000000, -0.000000000000000000, -0.000000000000000000 ) ) ;
#7992=EDGE_CURVE ( 'NONE', #42209, #9166, #31184, .T. ) ;
#8005=CARTESIAN_POINT ( 'NONE',  ( 344.0000000000000000, -164.9999999999999432, 339.9999999999998295 ) ) ;
#8008=DIRECTION ( 'NONE',  ( 0.000000000000000000, -1.000000000000000000, 0.000000000000000000 ) ) ;
#8011=DIRECTION ( 'NONE',  ( -0.000000000000000000, 1.000000000000000000, 0.000000000000000000 ) ) ;
#8013=EDGE_CURVE ( 'NONE', #48818, #16044, #12181, .T. ) ;
#8014=CYLINDRICAL_SURFACE ( 'NONE', #28099, 2.000000000000001776 ) ;
#8016=EDGE_CURVE ( 'NONE', #28737, #16142, #27014, .T. ) ;
#8019=ORIENTED_EDGE ( 'NONE', *, *, #4675, .T. ) ;
#8023=DIRECTION ( 'NONE',  ( 1.000000000000000000, 0.000000000000000000, 1.612977847700450206E-50 ) ) ;
#8027=ORIENTED_EDGE ( 'NONE', *, *, #48379, .T. ) ;
#8028=EDGE_CURVE ( 'NONE', #3051, #36488, #3716, .T. ) ;
#8029=DIRECTION ( 'NONE',  ( 0.000000000000000000, 5.664403186863042467E-17, 1.000000000000000000 ) ) ;
#8038=EDGE_CURVE ( 'NONE', #17953, #26847, #27065, .T. ) ;
#8041=DIRECTION ( 'NONE',  ( 1.000000000000000000, 0.000000000000000000, 0.000000000000000000 ) ) ;
#8043=EDGE_CURVE ( 'NONE', #43960, #48553, #23208, .T. ) ;
#8060=EDGE_CURVE ( 'NONE', #26993, #48818, #4475, .T. ) ;
#8064=EDGE_CURVE ( 'NONE', #46163, #28405, #42779, .T. ) ;
#8068=LINE ( 'NONE', #23189, #38362 ) ;
#8071=CARTESIAN_POINT ( 'NONE',  ( 358.0000000000000568, -167.8284271247462414, 342.8284271247461561 ) ) ;
#8074=ORIENTED_EDGE ( 'NONE', *, *, #41579, .T. ) ;
#8077=DIRECTION ( 'NONE',  ( 0.000000000000000000, 1.000000000000000000, 0.000000000000000000 ) ) ;
#8080=EDGE_CURVE ( 'NONE', #39358, #13701, #35207, .T. ) ;
#8086=DIRECTION ( 'NONE',  ( 0.000000000000000000, -1.000000000000000000, 3.469446951953611033E-15 ) ) ;
#8090=CLOSED_SHELL ( 'NONE', ( #17781, #1511, #16443, #1412, #28219, #30596, #32262, #13065, #1406, #38290, #27511, #40150, #38230, #433, #20518, #44413, #46795, #30209 ) ) ;
#8093=LINE ( 'NONE', #49851, #15649 ) ;
#8094=ORIENTED_EDGE ( 'NONE', *, *, #40299, .T. ) ;
#8098=CARTESIAN_POINT ( 'NONE',  ( -5.000000000000000000, -175.0000000000000284, -353.7500000000001705 ) ) ;
#8099=CARTESIAN_POINT ( 'NONE',  ( 181.0000000000000000, -174.9999999999999716, -358.0000000000001705 ) ) ;
#8104=ORIENTED_EDGE ( 'NONE', *, *, #16854, .F. ) ;
#8110=ORIENTED_EDGE ( 'NONE', *, *, #21721, .T. ) ;
#8114=LINE ( 'NONE', #42477, #17528 ) ;
#8115=ADVANCED_FACE ( 'NONE', ( #32690, #28840 ), #9343, .T. ) ;
#8125=CARTESIAN_POINT ( 'NONE',  ( 340.0000000000000568, 169.0000000000000000, 343.9999999999998295 ) ) ;
#8129=AXIS2_PLACEMENT_3D ( 'NONE', #19078, #12156, #3688 ) ;
#8130=ORIENTED_EDGE ( 'NONE', *, *, #20197, .F. ) ;
#8131=VECTOR ( 'NONE', #48179, 1000.000000000000000 ) ;
#8134=EDGE_CURVE ( 'NONE', #8840, #6226, #47999, .T. ) ;
#8142=ORIENTED_EDGE ( 'NONE', *, *, #30192, .T. ) ;
#8143=( NAMED_UNIT ( * ) PLANE_ANGLE_UNIT ( ) SI_UNIT ( $, .RADIAN. ) );
#8156=VECTOR ( 'NONE', #37117, 1000.000000000000000 ) ;
#8164=DIRECTION ( 'NONE',  ( 0.000000000000000000, -1.000000000000000000, 0.000000000000000000 ) ) ;
#8167=AXIS2_PLACEMENT_3D ( 'NONE', #11417, #637, #27592 ) ;
#8169=DIRECTION ( 'NONE',  ( 1.000000000000000000, 0.000000000000000000, 7.793956916774525800E-48 ) ) ;
#8172=VERTEX_POINT ( 'NONE', #28336 ) ;
#8180=CARTESIAN_POINT ( 'NONE',  ( -5.000000000000000000, -165.1999999999999602, 340.1999999999997044 ) ) ;
#8187=DIRECTION ( 'NONE',  ( 0.000000000000000000, 1.000000000000000000, 6.123233995736766036E-17 ) ) ;
#8197=ORIENTED_EDGE ( 'NONE', *, *, #13591, .T. ) ;
#8198=AXIS2_PLACEMENT_3D ( 'NONE', #36722, #1791, #13580 ) ;
#8202=CARTESIAN_POINT ( 'NONE',  ( 168.9999999999999716, -164.9999999999999432, -358.0000000000001705 ) ) ;
#8203=DIRECTION ( 'NONE',  ( 1.000000000000000000, 0.000000000000000000, 0.000000000000000000 ) ) ;
#8208=DIRECTION ( 'NONE',  ( -1.000000000000000000, 0.000000000000000000, -7.793956916774525800E-48 ) ) ;
#8209=VERTEX_POINT ( 'NONE', #40651 ) ;
#8214=LINE ( 'NONE', #761, #32292 ) ;
#8215=ORIENTED_EDGE ( 'NONE', *, *, #49247, .F. ) ;
#8220=DIRECTION ( 'NONE',  ( -1.000000000000000000, 0.000000000000000000, 0.000000000000000000 ) ) ;
#8228=CARTESIAN_POINT ( 'NONE',  ( 0.000000000000000000, 169.0000000000000000, 341.9999999999997726 ) ) ;
#8230=CARTESIAN_POINT ( 'NONE',  ( 0.000000000000000000, 169.0000000000000000, -340.0000000000001705 ) ) ;
#8233=AXIS2_PLACEMENT_3D ( 'NONE', #39734, #40734, #9423 ) ;
#8237=CARTESIAN_POINT ( 'NONE',  ( 356.0000000000000000, 175.0000000000000284, -106.0000000000001990 ) ) ;
#8240=DIRECTION ( 'NONE',  ( 0.000000000000000000, 0.000000000000000000, 1.000000000000000000 ) ) ;
#8242=CARTESIAN_POINT ( 'NONE',  ( 350.0000000000000000, 181.0000000000000284, -344.0000000000001705 ) ) ;
#8244=EDGE_CURVE ( 'NONE', #18475, #35109, #38066, .T. ) ;
#8247=ORIENTED_EDGE ( 'NONE', *, *, #46136, .F. ) ;
#8252=EDGE_LOOP ( 'NONE', ( #20325, #2814, #50459, #9150 ) ) ;
#8255=EDGE_CURVE ( 'NONE', #24755, #50534, #32739, .T. ) ;
#8258=CARTESIAN_POINT ( 'NONE',  ( 358.0000000000000000, 174.9999999999996589, -344.0000000000002842 ) ) ;
#8259=CIRCLE ( 'NONE', #45898, 2.000000000000001776 ) ;
#8262=VECTOR ( 'NONE', #11617, 1000.000000000000000 ) ;
#8266=VERTEX_POINT ( 'NONE', #42139 ) ;
#8267=CARTESIAN_POINT ( 'NONE',  ( 350.0000000000001137, 181.0000000000000284, 341.9999999999997726 ) ) ;
#8276=EDGE_CURVE ( 'NONE', #45035, #269, #14449, .T. ) ;
#8278=CARTESIAN_POINT ( 'NONE',  ( 359.9999999999999432, -169.0000000000001705, 344.0000000000000000 ) ) ;
#8280=LINE ( 'NONE', #15973, #8262 ) ;
#8281=CARTESIAN_POINT ( 'NONE',  ( 181.0000000000000284, -9.999999999999953815, -99.00000000000014211 ) ) ;
#8284=EDGE_CURVE ( 'NONE', #38138, #21789, #2154, .T. ) ;
#8293=VERTEX_POINT ( 'NONE', #45965 ) ;
#8295=EDGE_LOOP ( 'NONE', ( #17009, #9587, #45023, #474 ) ) ;
#8299=VECTOR ( 'NONE', #40851, 1000.000000000000000 ) ;
#8303=ADVANCED_FACE ( 'NONE', ( #25752 ), #48801, .T. ) ;
#8308=EDGE_CURVE ( 'NONE', #13701, #27139, #49040, .T. ) ;
#8309=CYLINDRICAL_SURFACE ( 'NONE', #47774, 4.000000000000003553 ) ;
#8311=VERTEX_POINT ( 'NONE', #25489 ) ;
#8316=FACE_OUTER_BOUND ( 'NONE', #15406, .T. ) ;
#8317=EDGE_LOOP ( 'NONE', ( #13925, #41557, #13560, #28285 ) ) ;
#8318=CARTESIAN_POINT ( 'NONE',  ( 181.0000000000000000, -97.49999999999998579, -340.0000000000001137 ) ) ;
#8324=VERTEX_POINT ( 'NONE', #21905 ) ;
#8332=AXIS2_PLACEMENT_3D ( 'NONE', #26921, #42815, #10759 ) ;
#8342=EDGE_LOOP ( 'NONE', ( #24557, #36009, #22961, #6138 ) ) ;
#8346=EDGE_CURVE ( 'NONE', #16242, #27082, #3392, .T. ) ;
#8353=LINE ( 'NONE', #31713, #21496 ) ;
#8356=FACE_OUTER_BOUND ( 'NONE', #34911, .T. ) ;
#8359=ORIENTED_EDGE ( 'NONE', *, *, #28826, .F. ) ;
#8368=( LENGTH_UNIT ( ) NAMED_UNIT ( * ) SI_UNIT ( .MILLI., .METRE. ) );
#8379=DIRECTION ( 'NONE',  ( 1.132880637372608740E-16, 4.718402560806925739E-50, 1.000000000000000000 ) ) ;
#8381=ORIENTED_EDGE ( 'NONE', *, *, #7158, .F. ) ;
#8383=CARTESIAN_POINT ( 'NONE',  ( 164.9999999999999716, -164.9999999999999432, -344.0000000000001137 ) ) ;
#8386=DIRECTION ( 'NONE',  ( 4.755310728521421461E-16, 0.000000000000000000, 1.000000000000000000 ) ) ;
#8387=LINE ( 'NONE', #9134, #44164 ) ;
#8391=DIRECTION ( 'NONE',  ( -1.000000000000000000, 0.000000000000000000, -0.000000000000000000 ) ) ;
#8393=EDGE_CURVE ( 'NONE', #34818, #35344, #11874, .T. ) ;
#8396=ORIENTED_EDGE ( 'NONE', *, *, #46363, .T. ) ;
#8408=EDGE_CURVE ( 'NONE', #5803, #24755, #336, .T. ) ;
#8413=CARTESIAN_POINT ( 'NONE',  ( 168.9999999999999716, 165.0000000000000000, -358.0000000000001705 ) ) ;
#8414=DIRECTION ( 'NONE',  ( 1.000000000000000000, 0.000000000000000000, -1.586032892321652482E-16 ) ) ;
#8417=CARTESIAN_POINT ( 'NONE',  ( 357.9999999999999432, -181.0000000000001421, -349.9999999999999432 ) ) ;
#8418=ORIENTED_EDGE ( 'NONE', *, *, #45999, .F. ) ;
#8419=PLANE ( 'NONE',  #18444 ) ;
#8420=DIRECTION ( 'NONE',  ( 1.333906992743555050E-23, -1.000000000000000000, 0.000000000000000000 ) ) ;
#8424=CARTESIAN_POINT ( 'NONE',  ( 164.9999999999999716, 175.0000000000000284, -344.0000000000001137 ) ) ;
#8428=CARTESIAN_POINT ( 'NONE',  ( 340.0000000000000568, 167.0000000000000000, 343.9999999999997726 ) ) ;
#8429=CIRCLE ( 'NONE', #32195, 4.000000000000003553 ) ;
#8430=DIRECTION ( 'NONE',  ( 0.000000000000000000, -2.537652627714643577E-15, -1.000000000000000000 ) ) ;
#8431=ORIENTED_EDGE ( 'NONE', *, *, #24961, .F. ) ;
#8435=CARTESIAN_POINT ( 'NONE',  ( 355.9999999999999432, -183.0000000000000000, 357.9999999999998295 ) ) ;
#8436=DIRECTION ( 'NONE',  ( -1.000000000000000000, 0.000000000000000000, 0.000000000000000000 ) ) ;
#8447=CARTESIAN_POINT ( 'NONE',  ( 355.9999999999999432, -165.0000000000001137, -106.0000000000001990 ) ) ;
#8449=DIRECTION ( 'NONE',  ( 3.172065745548403743E-16, 1.000000000000000000, 0.000000000000000000 ) ) ;
#8450=ORIENTED_EDGE ( 'NONE', *, *, #39309, .T. ) ;
#8455=DIRECTION ( 'NONE',  ( -0.000000000000000000, -0.000000000000000000, 1.000000000000000000 ) ) ;
#8464=VERTEX_POINT ( 'NONE', #31890 ) ;
#8468=EDGE_CURVE ( 'NONE', #2419, #41044, #1084, .T. ) ;
#8483=VERTEX_POINT ( 'NONE', #47485 ) ;
#8486=DIRECTION ( 'NONE',  ( 0.000000000000000000, 7.004339610132985974E-48, 1.000000000000000000 ) ) ;
#8487=ORIENTED_EDGE ( 'NONE', *, *, #37699, .T. ) ;
#8489=CYLINDRICAL_SURFACE ( 'NONE', #25125, 2.000000000000001776 ) ;
#8496=LINE ( 'NONE', #32349, #36249 ) ;
#8498=ORIENTED_EDGE ( 'NONE', *, *, #34484, .F. ) ;
#8499=CARTESIAN_POINT ( 'NONE',  ( 349.9999999999999432, -166.9999999999999432, 343.9999999999997726 ) ) ;
#8500=DIRECTION ( 'NONE',  ( 1.368455531567204171E-48, -1.000000000000000000, -2.265761274745217480E-16 ) ) ;
#8507=CYLINDRICAL_SURFACE ( 'NONE', #5242, 2.000000000000001776 ) ;
#8513=LINE ( 'NONE', #32616, #976 ) ;
#8520=PLANE ( 'NONE',  #47681 ) ;
#8522=DIRECTION ( 'NONE',  ( -1.586032880504786307E-16, 1.654361225106055350E-24, -1.000000000000000000 ) ) ;
#8528=ORIENTED_EDGE ( 'NONE', *, *, #20326, .T. ) ;
#8532=ORIENTED_EDGE ( 'NONE', *, *, #16861, .T. ) ;
#8536=CARTESIAN_POINT ( 'NONE',  ( -5.000000000000000000, -165.1999999999999602, -340.2000000000001592 ) ) ;
#8541=ORIENTED_EDGE ( 'NONE', *, *, #8691, .T. ) ;
#8543=CARTESIAN_POINT ( 'NONE',  ( -5.000000000000000000, -165.1999999999999602, -359.8000000000002387 ) ) ;
#8548=DIRECTION ( 'NONE',  ( 0.000000000000000000, 0.000000000000000000, -1.000000000000000000 ) ) ;
#8556=ORIENTED_EDGE ( 'NONE', *, *, #8308, .F. ) ;
#8562=CARTESIAN_POINT ( 'NONE',  ( 339.9999999999998863, -168.9999999999999432, 341.9999999999997726 ) ) ;
#8563=ORIENTED_EDGE ( 'NONE', *, *, #41926, .T. ) ;
#8568=FACE_OUTER_BOUND ( 'NONE', #33740, .T. ) ;
#8570=CARTESIAN_POINT ( 'NONE',  ( -5.000000000000000000, 175.0000000000000284, -346.2500000000002274 ) ) ;
#8575=DIRECTION ( 'NONE',  ( -1.000000000000000000, 3.172065784643302499E-16, 1.942330104924128867E-32 ) ) ;
#8580=CARTESIAN_POINT ( 'NONE',  ( 360.0000000000000000, 166.6568542494925964, -341.6568542494925396 ) ) ;
#8581=VERTEX_POINT ( 'NONE', #24189 ) ;
#8587=CARTESIAN_POINT ( 'NONE',  ( 0.000000000000000000, 165.0000000000000000, -344.0000000000001705 ) ) ;
#8593=EDGE_LOOP ( 'NONE', ( #33643, #26143, #11702, #30168 ) ) ;
#8596=DIRECTION ( 'NONE',  ( -1.586032892321652236E-16, -1.000000000000000000, -6.853681917100419162E-49 ) ) ;
#8604=DIRECTION ( 'NONE',  ( 0.000000000000000000, -1.000000000000000000, 0.000000000000000000 ) ) ;
#8606=VECTOR ( 'NONE', #30336, 1000.000000000000000 ) ;
#8607=ORIENTED_EDGE ( 'NONE', *, *, #376, .T. ) ;
#8608=ORIENTED_EDGE ( 'NONE', *, *, #44516, .T. ) ;
#8612=AXIS2_PLACEMENT_3D ( 'NONE', #16871, #48114, #36901 ) ;
#8618=EDGE_CURVE ( 'NONE', #32935, #50040, #45405, .T. ) ;
#8627=DIRECTION ( 'NONE',  ( 1.000000000000000000, -5.326388832052271710E-25, 1.587271980518778491E-16 ) ) ;
#8628=PLANE ( 'NONE',  #32685 ) ;
#8635=DIRECTION ( 'NONE',  ( 1.000000000000000000, -1.331116318405244905E-23, -4.759647537211363479E-16 ) ) ;
#8645=VERTEX_POINT ( 'NONE', #30053 ) ;
#8646=CARTESIAN_POINT ( 'NONE',  ( 350.0000000000000000, -164.9999999999999432, -356.0000000000002274 ) ) ;
#8648=( GEOMETRIC_REPRESENTATION_CONTEXT ( 3 ) GLOBAL_UNCERTAINTY_ASSIGNED_CONTEXT ( ( #46553 ) ) GLOBAL_UNIT_ASSIGNED_CONTEXT ( ( #52, #34965, #46188 ) ) REPRESENTATION_CONTEXT ( 'NONE', 'WORKASPACE' ) );
#8649=EDGE_CURVE ( 'NONE', #23178, #37052, #25408, .T. ) ;
#8654=ORIENTED_EDGE ( 'NONE', *, *, #50555, .F. ) ;
#8662=ORIENTED_EDGE ( 'NONE', *, *, #39685, .T. ) ;
#8666=FACE_OUTER_BOUND ( 'NONE', #3621, .T. ) ;
#8672=CARTESIAN_POINT ( 'NONE',  ( 181.0000000000000568, 165.0000000000000000, 343.9999999999998863 ) ) ;
#8686=CARTESIAN_POINT ( 'NONE',  ( 355.9999999999999432, -183.0000000000001421, 358.0000000000001705 ) ) ;
#8690=CIRCLE ( 'NONE', #11130, 2.000000000000001776 ) ;
#8691=EDGE_CURVE ( 'NONE', #14822, #32061, #17739, .T. ) ;
#8695=DIRECTION ( 'NONE',  ( 0.000000000000000000, 1.000000000000000000, 0.000000000000000000 ) ) ;
#8705=LINE ( 'NONE', #39499, #14236 ) ;
#8712=DIRECTION ( 'NONE',  ( 1.132880637372608740E-16, 4.718402560806925739E-50, 1.000000000000000000 ) ) ;
#8718=DIRECTION ( 'NONE',  ( 0.000000000000000000, -2.265761274745217480E-16, 1.000000000000000000 ) ) ;
#8719=VERTEX_POINT ( 'NONE', #35434 ) ;
#8721=CYLINDRICAL_SURFACE ( 'NONE', #29852, 3.749999999999975575 ) ;
#8724=( LENGTH_UNIT ( ) NAMED_UNIT ( * ) SI_UNIT ( .MILLI., .METRE. ) );
#8725=VERTEX_POINT ( 'NONE', #31582 ) ;
#8727=CIRCLE ( 'NONE', #25934, 4.000000000000003553 ) ;
#8729=FACE_OUTER_BOUND ( 'NONE', #45215, .T. ) ;
#8730=VECTOR ( 'NONE', #24841, 1000.000000000000000 ) ;
#8735=CARTESIAN_POINT ( 'NONE',  ( 5.551115123125782702E-14, -164.9999999999999432, 343.9999999999997726 ) ) ;
#8737=AXIS2_PLACEMENT_3D ( 'NONE', #21080, #4686, #5428 ) ;
#8739=ORIENTED_EDGE ( 'NONE', *, *, #32485, .T. ) ;
#8745=LINE ( 'NONE', #31074, #2979 ) ;
#8751=EDGE_CURVE ( 'NONE', #32061, #14517, #2, .T. ) ;
#8753=DIRECTION ( 'NONE',  ( -1.000000000000000000, 0.000000000000000000, -2.958228394578794270E-31 ) ) ;
#8755=DIRECTION ( 'NONE',  ( -1.586032892321652236E-16, -1.000000000000000000, -2.288264760618012091E-48 ) ) ;
#8759=ORIENTED_EDGE ( 'NONE', *, *, #50350, .F. ) ;
#8762=EDGE_CURVE ( 'NONE', #18285, #22723, #7463, .T. ) ;
#8763=PLANE ( 'NONE',  #30229 ) ;
#8766=CARTESIAN_POINT ( 'NONE',  ( 181.0000000000000000, -81.49999999999995737, -115.0000000000001563 ) ) ;
#8772=DIRECTION ( 'NONE',  ( -2.220446049250312588E-16, -0.7071067811865475727, 0.7071067811865474617 ) ) ;
#8775=VECTOR ( 'NONE', #20707, 1000.000000000000000 ) ;
#8782=CARTESIAN_POINT ( 'NONE',  ( 342.8284271247460993, -183.0000000000001137, -358.0000000000003411 ) ) ;
#8787=ORIENTED_EDGE ( 'NONE', *, *, #36574, .F. ) ;
#8790=DIRECTION ( 'NONE',  ( 1.132880637372608740E-16, 4.718402560806925739E-50, 1.000000000000000000 ) ) ;
#8798=DIRECTION ( 'NONE',  ( 1.000000000000000000, 0.000000000000000000, 0.000000000000000000 ) ) ;
#8800=FACE_OUTER_BOUND ( 'NONE', #21296, .T. ) ;
#8802=CARTESIAN_POINT ( 'NONE',  ( 181.0000000000000568, 175.0000000000000284, 355.9999999999998863 ) ) ;
#8809=ORIENTED_EDGE ( 'NONE', *, *, #28158, .T. ) ;
#8815=VERTEX_POINT ( 'NONE', #1281 ) ;
#8819=DIRECTION ( 'NONE',  ( 0.000000000000000000, -2.537652627714643577E-15, -1.000000000000000000 ) ) ;
#8820=AXIS2_PLACEMENT_3D ( 'NONE', #13722, #44754, #5773 ) ;
#8826=FACE_OUTER_BOUND ( 'NONE', #21803, .T. ) ;
#8829=DIRECTION ( 'NONE',  ( -1.000000000000000000, 0.000000000000000000, 0.000000000000000000 ) ) ;
#8830=ORIENTED_EDGE ( 'NONE', *, *, #48203, .F. ) ;
#8831=DIRECTION ( 'NONE',  ( -4.758098676964957447E-16, -1.000000000000000000, 7.143884938411937192E-48 ) ) ;
#8838=CARTESIAN_POINT ( 'NONE',  ( 360.0000000000000000, -166.6568542494924543, -341.6568542494926533 ) ) ;
#8840=VERTEX_POINT ( 'NONE', #36442 ) ;
#8844=ADVANCED_FACE ( 'NONE', ( #17171 ), #16171, .F. ) ;
#8847=ORIENTED_EDGE ( 'NONE', *, *, #18399, .F. ) ;
#8851=ORIENTED_EDGE ( 'NONE', *, *, #6207, .T. ) ;
#8852=VERTEX_POINT ( 'NONE', #24132 ) ;
#8853=ORIENTED_EDGE ( 'NONE', *, *, #21343, .F. ) ;
#8855=CARTESIAN_POINT ( 'NONE',  ( 356.0000000000000000, 174.9999999999996589, -340.0000000000002842 ) ) ;
#8856=ORIENTED_EDGE ( 'NONE', *, *, #45880, .F. ) ;
#8859=CYLINDRICAL_SURFACE ( 'NONE', #38825, 4.000000000000003553 ) ;
#8862=CARTESIAN_POINT ( 'NONE',  ( 181.0000000000000000, -184.9999999999999716, -358.0000000000001705 ) ) ;
#8865=CARTESIAN_POINT ( 'NONE',  ( 181.0000000000000284, -174.9999999999999716, -99.00000000000014211 ) ) ;
#8867=DIRECTION ( 'NONE',  ( 0.000000000000000000, 1.000000000000000000, 0.000000000000000000 ) ) ;
#8872=CARTESIAN_POINT ( 'NONE',  ( 350.0000000000000000, 169.0000000000000000, -344.0000000000001705 ) ) ;
#8878=DIRECTION ( 'NONE',  ( -1.612977847700450206E-50, 0.000000000000000000, -1.000000000000000000 ) ) ;
#8887=EDGE_LOOP ( 'NONE', ( #38105, #24327, #36526, #40885 ) ) ;
#8891=ORIENTED_EDGE ( 'NONE', *, *, #3186, .F. ) ;
#8895=ADVANCED_FACE ( 'NONE', ( #32074, #35691 ), #9214, .T. ) ;
#8900=EDGE_CURVE ( 'NONE', #19122, #42389, #8970, .T. ) ;
#8902=CARTESIAN_POINT ( 'NONE',  ( 356.0000000000000568, 175.0000000000000284, -94.00000000000019895 ) ) ;
#8909=CARTESIAN_POINT ( 'NONE',  ( 168.9999999999997158, -164.9999999999999432, 341.9999999999998863 ) ) ;
#8910=DIRECTION ( 'NONE',  ( 1.000000000000000000, 0.000000000000000000, 0.000000000000000000 ) ) ;
#8911=CIRCLE ( 'NONE', #44128, 4.000000000000003553 ) ;
#8914=VECTOR ( 'NONE', #26803, 1000.000000000000000 ) ;
#8933=CARTESIAN_POINT ( 'NONE',  ( 0.000000000000000000, -165.1999999999999602, -340.2000000000001592 ) ) ;
#8943=DIRECTION ( 'NONE',  ( 0.000000000000000000, 2.537652627714642000E-15, 1.000000000000000000 ) ) ;
#8947=DIRECTION ( 'NONE',  ( -3.172065784643302499E-16, -1.000000000000000000, 2.537652627714642000E-15 ) ) ;
#8948=EDGE_CURVE ( 'NONE', #35933, #34629, #29228, .T. ) ;
#8958=AXIS2_PLACEMENT_3D ( 'NONE', #44076, #8943, #19983 ) ;
#8964=EDGE_CURVE ( 'NONE', #36804, #34812, #46051, .T. ) ;
#8969=ORIENTED_EDGE ( 'NONE', *, *, #30339, .T. ) ;
#8970=LINE ( 'NONE', #40274, #10673 ) ;
#8973=CARTESIAN_POINT ( 'NONE',  ( 168.9999999999999716, -180.9999999999999716, -350.0000000000001705 ) ) ;
#8974=EDGE_CURVE ( 'NONE', #34532, #36302, #41526, .T. ) ;
#8977=ADVANCED_FACE ( 'NONE', ( #6371, #21515 ), #22019, .T. ) ;
#8987=AXIS2_PLACEMENT_3D ( 'NONE', #29225, #47662, #4849 ) ;
#8991=LINE ( 'NONE', #35453, #46678 ) ;
#8993=AXIS2_PLACEMENT_3D ( 'NONE', #50356, #15270, #18833 ) ;
#8995=ORIENTED_EDGE ( 'NONE', *, *, #3857, .F. ) ;
#9007=CARTESIAN_POINT ( 'NONE',  ( 169.0000000000000000, 2.775557561562891351E-14, -99.00000000000014211 ) ) ;
#9011=CARTESIAN_POINT ( 'NONE',  ( 360.0000000000000000, -166.6568542494925396, -341.6568542494927101 ) ) ;
#9017=DIRECTION ( 'NONE',  ( -4.758098676964957447E-16, -1.000000000000000000, 7.143884938411937192E-48 ) ) ;
#9019=CARTESIAN_POINT ( 'NONE',  ( 350.0000000000000000, -182.9999999999999716, -356.0000000000002274 ) ) ;
#9020=DIRECTION ( 'NONE',  ( 0.000000000000000000, -1.000000000000000000, 0.000000000000000000 ) ) ;
#9021=CARTESIAN_POINT ( 'NONE',  ( 350.0000000000000000, 181.0000000000000284, -360.0000000000002274 ) ) ;
#9034=PLANE ( 'NONE',  #32404 ) ;
#9046=CARTESIAN_POINT ( 'NONE',  ( 183.0000000000000000, -256.5000000000000568, -114.9999999999999574 ) ) ;
#9047=DIRECTION ( 'NONE',  ( -1.000000000000000000, 0.000000000000000000, -1.612977847700450206E-50 ) ) ;
#9052=FACE_OUTER_BOUND ( 'NONE', #18429, .T. ) ;
#9055=CARTESIAN_POINT ( 'NONE',  ( 356.0000000000000000, -169.0000000000001137, -349.9999999999999432 ) ) ;
#9063=VERTEX_POINT ( 'NONE', #3019 ) ;
#9064=LINE ( 'NONE', #32163, #17650 ) ;
#9068=FACE_OUTER_BOUND ( 'NONE', #43190, .T. ) ;
#9071=CARTESIAN_POINT ( 'NONE',  ( 167.0000000000000000, 2.775557561562891351E-14, -99.00000000000014211 ) ) ;
#9072=DIRECTION ( 'NONE',  ( 1.000000000000000000, -4.996003610813203446E-16, -7.930164450086814785E-16 ) ) ;
#9075=VECTOR ( 'NONE', #40164, 1000.000000000000000 ) ;
#9077=CIRCLE ( 'NONE', #38573, 3.749999999999975575 ) ;
#9078=CARTESIAN_POINT ( 'NONE',  ( 356.0000000000000000, 165.0000000000000000, -108.0000000000002132 ) ) ;
#9079=EDGE_CURVE ( 'NONE', #39109, #20342, #38701, .T. ) ;
#9089=EDGE_CURVE ( 'NONE', #921, #33108, #18667, .T. ) ;
#9090=PLANE ( 'NONE',  #33641 ) ;
#9099=EDGE_CURVE ( 'NONE', #40964, #19479, #37659, .T. ) ;
#9104=DIRECTION ( 'NONE',  ( 0.000000000000000000, 0.000000000000000000, 1.000000000000000000 ) ) ;
#9107=CARTESIAN_POINT ( 'NONE',  ( 358.3431457505075741, 185.0000000000000568, 359.9999999999998295 ) ) ;
#9110=EDGE_CURVE ( 'NONE', #44276, #10712, #27848, .T. ) ;
#9122=EDGE_LOOP ( 'NONE', ( #12637, #17179 ) ) ;
#9124=PLANE ( 'NONE',  #27676 ) ;
#9134=CARTESIAN_POINT ( 'NONE',  ( 185.0000000000000000, -174.9999999999999716, -344.0000000000001137 ) ) ;
#9138=ORIENTED_EDGE ( 'NONE', *, *, #4842, .F. ) ;
#9141=ORIENTED_EDGE ( 'NONE', *, *, #28449, .F. ) ;
#9143=PLANE ( 'NONE',  #35510 ) ;
#9149=CARTESIAN_POINT ( 'NONE',  ( 358.0000000000001137, 180.9999999999999716, 355.9999999999997726 ) ) ;
#9150=ORIENTED_EDGE ( 'NONE', *, *, #43382, .T. ) ;
#9157=DIRECTION ( 'NONE',  ( 1.000000000000000000, -7.930164457481157120E-16, 1.587271980518778491E-16 ) ) ;
#9164=AXIS2_PLACEMENT_3D ( 'NONE', #15191, #30853, #30334 ) ;
#9166=VERTEX_POINT ( 'NONE', #44767 ) ;
#9167=ORIENTED_EDGE ( 'NONE', *, *, #10781, .F. ) ;
#9170=ADVANCED_FACE ( 'NONE', ( #37114 ), #1942, .F. ) ;
#9172=ORIENTED_EDGE ( 'NONE', *, *, #41912, .T. ) ;
#9179=CARTESIAN_POINT ( 'NONE',  ( 0.000000000000000000, 165.2000000000000171, -359.8000000000002387 ) ) ;
#9185=EDGE_CURVE ( 'NONE', #18651, #22117, #6545, .T. ) ;
#9191=CARTESIAN_POINT ( 'NONE',  ( 185.0000000000000000, -268.4999999999999432, -349.9999999999999432 ) ) ;
#9199=CARTESIAN_POINT ( 'NONE',  ( 168.9999999999999716, -164.9999999999999432, -360.0000000000002274 ) ) ;
#9200=DIRECTION ( 'NONE',  ( 0.000000000000000000, 1.000000000000000000, 4.687818848539279227E-49 ) ) ;
#9202=EDGE_LOOP ( 'NONE', ( #25961, #12881, #32664, #49823 ) ) ;
#9207=VERTEX_POINT ( 'NONE', #41948 ) ;
#9214=PLANE ( 'NONE',  #41805 ) ;
#9224=DIRECTION ( 'NONE',  ( -0.000000000000000000, -1.000000000000000000, 2.537652627714643577E-15 ) ) ;
#9231=AXIS2_PLACEMENT_3D ( 'NONE', #18812, #42171, #46493 ) ;
#9237=LINE ( 'NONE', #37228, #38691 ) ;
#9239=VERTEX_POINT ( 'NONE', #29388 ) ;
#9241=CARTESIAN_POINT ( 'NONE',  ( 168.9999999999999716, 8.000000000000062172, 339.9999999999998295 ) ) ;
#9253=AXIS2_PLACEMENT_3D ( 'NONE', #40798, #17448, #33119 ) ;
#9262=DIRECTION ( 'NONE',  ( 0.000000000000000000, 1.000000000000000000, 3.186989995019654210E-49 ) ) ;
#9271=AXIS2_PLACEMENT_3D ( 'NONE', #31293, #495, #24353 ) ;
#9286=VERTEX_POINT ( 'NONE', #3904 ) ;
#9287=DIRECTION ( 'NONE',  ( 0.000000000000000000, -2.265761274745217480E-16, 1.000000000000000000 ) ) ;
#9290=DIRECTION ( 'NONE',  ( 1.000000000000000000, 0.000000000000000000, 7.793956916774525800E-48 ) ) ;
#9291=VERTEX_POINT ( 'NONE', #23662 ) ;
#9294=DIRECTION ( 'NONE',  ( -7.793956916774524585E-48, 0.000000000000000000, -1.000000000000000000 ) ) ;
#9295=FACE_OUTER_BOUND ( 'NONE', #4957, .T. ) ;
#9297=CARTESIAN_POINT ( 'NONE',  ( 356.0000000000001137, 181.0000000000000284, 349.9999999999998863 ) ) ;
#9303=ORIENTED_EDGE ( 'NONE', *, *, #25020, .F. ) ;
#9308=CARTESIAN_POINT ( 'NONE',  ( 350.0000000000000000, -168.9999999999999432, -358.0000000000002274 ) ) ;
#9309=ORIENTED_EDGE ( 'NONE', *, *, #45252, .F. ) ;
#9310=( GEOMETRIC_REPRESENTATION_CONTEXT ( 3 ) GLOBAL_UNCERTAINTY_ASSIGNED_CONTEXT ( ( #4002 ) ) GLOBAL_UNIT_ASSIGNED_CONTEXT ( ( #34161, #27203, #11553 ) ) REPRESENTATION_CONTEXT ( 'NONE', 'WORKASPACE' ) );
#9311=CARTESIAN_POINT ( 'NONE',  ( 359.9999999999999432, 174.9999999999996589, -356.0000000000003411 ) ) ;
#9315=CARTESIAN_POINT ( 'NONE',  ( -5.000000000000000000, 0.000000000000000000, 0.000000000000000000 ) ) ;
#9320=DIRECTION ( 'NONE',  ( 0.000000000000000000, 1.000000000000000000, -2.969158215481698263E-48 ) ) ;
#9327=EDGE_CURVE ( 'NONE', #11298, #14780, #19299, .T. ) ;
#9331=ORIENTED_EDGE ( 'NONE', *, *, #24960, .F. ) ;
#9337=ADVANCED_FACE ( 'NONE', ( #38577 ), #19041, .F. ) ;
#9343=PLANE ( 'NONE',  #4057 ) ;
#9346=ORIENTED_EDGE ( 'NONE', *, *, #42207, .F. ) ;
#9351=ORIENTED_EDGE ( 'NONE', *, *, #13688, .F. ) ;
#9361=EDGE_LOOP ( 'NONE', ( #48661, #23097, #22922, #12239, #36221, #37777, #5611, #8853 ) ) ;
#9369=ORIENTED_EDGE ( 'NONE', *, *, #31964, .F. ) ;
#9373=CARTESIAN_POINT ( 'NONE',  ( 169.0000000000000284, 175.0000000000000284, 355.9999999999998863 ) ) ;
#9393=ORIENTED_EDGE ( 'NONE', *, *, #28688, .T. ) ;
#9395=AXIS2_PLACEMENT_3D ( 'NONE', #22191, #9876, #22433 ) ;
#9397=VECTOR ( 'NONE', #22567, 1000.000000000000000 ) ;
#9400=CARTESIAN_POINT ( 'NONE',  ( 350.0000000000000000, -168.9999999999999432, -344.0000000000001705 ) ) ;
#9408=LINE ( 'NONE', #17358, #30664 ) ;
#9409=AXIS2_PLACEMENT_3D ( 'NONE', #23557, #39215, #19702 ) ;
#9412=EDGE_CURVE ( 'NONE', #40195, #16306, #44401, .T. ) ;
#9421=EDGE_LOOP ( 'NONE', ( #22636, #11887, #27217, #7354 ) ) ;
#9422=VERTEX_POINT ( 'NONE', #24435 ) ;
#9423=DIRECTION ( 'NONE',  ( 1.000000000000000000, 0.000000000000000000, 0.000000000000000000 ) ) ;
#9436=FACE_OUTER_BOUND ( 'NONE', #32893, .T. ) ;
#9446=CIRCLE ( 'NONE', #14353, 2.000000000000001776 ) ;
#9448=ORIENTED_EDGE ( 'NONE', *, *, #5640, .F. ) ;
#9450=FACE_OUTER_BOUND ( 'NONE', #2836, .T. ) ;
#9455=ORIENTED_EDGE ( 'NONE', *, *, #27646, .F. ) ;
#9460=VECTOR ( 'NONE', #390, 1000.000000000000000 ) ;
#9461=ORIENTED_EDGE ( 'NONE', *, *, #38597, .F. ) ;
#9464=VECTOR ( 'NONE', #46576, 1000.000000000000000 ) ;
#9469=VECTOR ( 'NONE', #4655, 1000.000000000000000 ) ;
#9474=DIRECTION ( 'NONE',  ( 0.000000000000000000, 0.000000000000000000, -1.000000000000000000 ) ) ;
#9477=VECTOR ( 'NONE', #3420, 1000.000000000000000 ) ;
#9481=LINE ( 'NONE', #9730, #7102 ) ;
#9482=VERTEX_POINT ( 'NONE', #47977 ) ;
#9488=ORIENTED_EDGE ( 'NONE', *, *, #36880, .T. ) ;
#9489=LINE ( 'NONE', #10257, #9756 ) ;
#9492=ORIENTED_EDGE ( 'NONE', *, *, #43322, .T. ) ;
#9493=ORIENTED_EDGE ( 'NONE', *, *, #23991, .F. ) ;
#9497=CIRCLE ( 'NONE', #42279, 4.000000000000003553 ) ;
#9501=FACE_OUTER_BOUND ( 'NONE', #4830, .T. ) ;
#9503=LINE ( 'NONE', #3568, #15464 ) ;
#9510=LINE ( 'NONE', #29773, #18229 ) ;
#9511=ORIENTED_EDGE ( 'NONE', *, *, #6239, .T. ) ;
#9515=CARTESIAN_POINT ( 'NONE',  ( 168.9999999999999716, -97.49999999999998579, -340.0000000000001137 ) ) ;
#9519=AXIS2_PLACEMENT_3D ( 'NONE', #28286, #20826, #20328 ) ;
#9530=ORIENTED_EDGE ( 'NONE', *, *, #737, .T. ) ;
#9533=CARTESIAN_POINT ( 'NONE',  ( -5.000000000000000000, -184.7999999999999545, -359.8000000000002387 ) ) ;
#9541=VECTOR ( 'NONE', #15669, 1000.000000000000000 ) ;
#9542=ORIENTED_EDGE ( 'NONE', *, *, #39388, .T. ) ;
#9547=DIRECTION ( 'NONE',  ( 0.000000000000000000, 2.265761274745217480E-16, -1.000000000000000000 ) ) ;
#9549=CYLINDRICAL_SURFACE ( 'NONE', #24356, 4.000000000000003553 ) ;
#9552=DIRECTION ( 'NONE',  ( 2.775557561562891351E-16, 0.7071067811865477948, 0.7071067811865473507 ) ) ;
#9560=CARTESIAN_POINT ( 'NONE',  ( 339.9999999999999432, -180.9999999999999716, -340.0000000000001705 ) ) ;
#9564=AXIS2_PLACEMENT_3D ( 'NONE', #37454, #33342, #2272 ) ;
#9569=FACE_BOUND ( 'NONE', #46022, .T. ) ;
#9571=ADVANCED_FACE ( 'NONE', ( #6679 ), #34163, .F. ) ;
#9573=CARTESIAN_POINT ( 'NONE',  ( 164.9999999999999716, -5.999999999999950262, -340.0000000000001137 ) ) ;
#9574=DIRECTION ( 'NONE',  ( -1.612977847700450206E-50, 0.000000000000000000, -1.000000000000000000 ) ) ;
#9580=CIRCLE ( 'NONE', #26798, 2.000000000000001776 ) ;
#9582=FACE_OUTER_BOUND ( 'NONE', #31883, .T. ) ;
#9585=CARTESIAN_POINT ( 'NONE',  ( 356.0000000000003411, 165.0000000000000000, -92.00000000000019895 ) ) ;
#9587=ORIENTED_EDGE ( 'NONE', *, *, #44110, .T. ) ;
#9594=ORIENTED_EDGE ( 'NONE', *, *, #12105, .T. ) ;
#9596=DIRECTION ( 'NONE',  ( 0.000000000000000000, 0.000000000000000000, -1.000000000000000000 ) ) ;
#9597=AXIS2_PLACEMENT_3D ( 'NONE', #35007, #19564, #31397 ) ;
#9598=CARTESIAN_POINT ( 'NONE',  ( 0.000000000000000000, -165.1999999999999602, 340.1999999999997044 ) ) ;
#9603=CARTESIAN_POINT ( 'NONE',  ( 168.9999999999999716, -272.5000000000000000, -94.99999999999988631 ) ) ;
#9605=DIRECTION ( 'NONE',  ( -0.000000000000000000, -0.000000000000000000, 1.000000000000000000 ) ) ;
#9609=ORIENTED_EDGE ( 'NONE', *, *, #17355, .F. ) ;
#9618=DIRECTION ( 'NONE',  ( 0.000000000000000000, -2.265761274745217480E-16, 1.000000000000000000 ) ) ;
#9634=LINE ( 'NONE', #40936, #39609 ) ;
#9636=DIRECTION ( 'NONE',  ( 0.000000000000000000, 0.000000000000000000, 1.000000000000000000 ) ) ;
#9637=DIRECTION ( 'NONE',  ( -1.586032880504786307E-16, 1.654361225106055350E-24, -1.000000000000000000 ) ) ;
#9644=DIRECTION ( 'NONE',  ( 0.000000000000000000, 1.544785076050074834E-48, 1.000000000000000000 ) ) ;
#9650=ORIENTED_EDGE ( 'NONE', *, *, #498, .F. ) ;
#9654=CARTESIAN_POINT ( 'NONE',  ( 168.9999999999999716, -254.4999999999999432, -339.9999999999998863 ) ) ;
#9664=CARTESIAN_POINT ( 'NONE',  ( 168.9999999999999716, -77.49999999999995737, -115.0000000000001563 ) ) ;
#9665=EDGE_CURVE ( 'NONE', #15345, #24207, #3773, .T. ) ;
#9669=DIRECTION ( 'NONE',  ( 1.000000000000000000, -4.758098676964956461E-16, -8.975803739141899931E-48 ) ) ;
#9677=LINE ( 'NONE', #20460, #5375 ) ;
#9679=CARTESIAN_POINT ( 'NONE',  ( 166.9999999999999716, -164.9999999999999432, 355.9999999999998863 ) ) ;
#9682=DIRECTION ( 'NONE',  ( 0.000000000000000000, 0.000000000000000000, 1.000000000000000000 ) ) ;
#9683=CARTESIAN_POINT ( 'NONE',  ( 181.0000000000001705, -166.9999999999999432, -115.0000000000001847 ) ) ;
#9693=LINE ( 'NONE', #45065, #14232 ) ;
#9696=CARTESIAN_POINT ( 'NONE',  ( 350.0000000000001137, 181.0000000000000284, 343.9999999999997726 ) ) ;
#9698=ADVANCED_FACE ( 'NONE', ( #39712 ), #20195, .F. ) ;
#9699=EDGE_LOOP ( 'NONE', ( #38299, #17940, #42655, #33434 ) ) ;
#9701=DIRECTION ( 'NONE',  ( -1.000000000000000000, 0.000000000000000000, -2.958228394578794270E-31 ) ) ;
#9703=DIRECTION ( 'NONE',  ( -1.000000000000000000, 0.000000000000000000, -2.958228394578794270E-31 ) ) ;
#9708=VERTEX_POINT ( 'NONE', #38268 ) ;
#9711=CIRCLE ( 'NONE', #13800, 2.000000000000001776 ) ;
#9712=EDGE_LOOP ( 'NONE', ( #16727, #32001, #47507, #6952 ) ) ;
#9718=DIRECTION ( 'NONE',  ( -1.000000000000000000, 4.996003610813203446E-16, 7.930164450086814785E-16 ) ) ;
#9719=CARTESIAN_POINT ( 'NONE',  ( 181.0000000000000000, -174.9999999999999716, -358.0000000000001705 ) ) ;
#9721=CARTESIAN_POINT ( 'NONE',  ( 349.9999999999999432, -180.9999999999999716, 359.9999999999997726 ) ) ;
#9723=DIRECTION ( 'NONE',  ( 1.000000000000000000, 0.000000000000000000, 1.612977847700450206E-50 ) ) ;
#9724=CARTESIAN_POINT ( 'NONE',  ( 341.6568542494922553, 165.0000000000000284, -339.9999999999999432 ) ) ;
#9729=EDGE_CURVE ( 'NONE', #26100, #47737, #50689, .T. ) ;
#9730=CARTESIAN_POINT ( 'NONE',  ( 350.0000000000001137, 181.0000000000000284, 357.9999999999997726 ) ) ;
#9735=DIRECTION ( 'NONE',  ( 1.132880637372608740E-16, 4.718402560806925739E-50, 1.000000000000000000 ) ) ;
#9741=ORIENTED_EDGE ( 'NONE', *, *, #33399, .T. ) ;
#9756=VECTOR ( 'NONE', #21804, 1000.000000000000000 ) ;
#9762=EDGE_LOOP ( 'NONE', ( #16186, #34761, #9461, #49324, #23687, #33579, #24922, #17561 ) ) ;
#9767=ORIENTED_EDGE ( 'NONE', *, *, #13609, .F. ) ;
#9769=ORIENTED_EDGE ( 'NONE', *, *, #1733, .F. ) ;
#9780=DIRECTION ( 'NONE',  ( 1.000000000000000000, -4.996003610813203446E-16, -1.586032878436834529E-16 ) ) ;
#9789=FACE_OUTER_BOUND ( 'NONE', #28115, .T. ) ;
#9794=EDGE_LOOP ( 'NONE', ( #44512, #29118, #15117, #27789 ) ) ;
#9796=CARTESIAN_POINT ( 'NONE',  ( 0.000000000000000000, -168.9999999999999432, -356.0000000000002274 ) ) ;
#9803=EDGE_LOOP ( 'NONE', ( #24500, #35219, #43473, #1925 ) ) ;
#9807=CARTESIAN_POINT ( 'NONE',  ( 165.0000000000000000, -174.9999999999999716, -99.00000000000014211 ) ) ;
#9810=CARTESIAN_POINT ( 'NONE',  ( 360.0000000000000568, -166.6568542494925396, 341.6568542494923122 ) ) ;
#9812=ORIENTED_EDGE ( 'NONE', *, *, #2208, .T. ) ;
#9815=LINE ( 'NONE', #25479, #45519 ) ;
#9816=EDGE_CURVE ( 'NONE', #22449, #9166, #48607, .T. ) ;
#9817=EDGE_CURVE ( 'NONE', #1522, #8172, #40960, .T. ) ;
#9821=EDGE_CURVE ( 'NONE', #40512, #25153, #5179, .T. ) ;
#9822=AXIS2_PLACEMENT_3D ( 'NONE', #11409, #49837, #42442 ) ;
#9826=ORIENTED_EDGE ( 'NONE', *, *, #15222, .T. ) ;
#9828=FACE_OUTER_BOUND ( 'NONE', #42596, .T. ) ;
#9832=CARTESIAN_POINT ( 'NONE',  ( 339.9999999999999432, -182.9999999999999716, -356.0000000000002274 ) ) ;
#9842=PLANE ( 'NONE',  #30817 ) ;
#9847=ORIENTED_EDGE ( 'NONE', *, *, #36191, .T. ) ;
#9852=EDGE_CURVE ( 'NONE', #15608, #25523, #30679, .T. ) ;
#9860=ORIENTED_EDGE ( 'NONE', *, *, #45089, .T. ) ;
#9862=CIRCLE ( 'NONE', #33617, 2.000000000000001776 ) ;
#9865=ORIENTED_EDGE ( 'NONE', *, *, #19874, .T. ) ;
#9870=ORIENTED_EDGE ( 'NONE', *, *, #11133, .F. ) ;
#9873=CYLINDRICAL_SURFACE ( 'NONE', #21922, 4.000000000000003553 ) ;
#9875=EDGE_CURVE ( 'NONE', #9063, #9286, #41460, .T. ) ;
#9876=DIRECTION ( 'NONE',  ( 0.000000000000000000, 2.537652627714642000E-15, 1.000000000000000000 ) ) ;
#9888=LINE ( 'NONE', #41181, #46592 ) ;
#9904=DIRECTION ( 'NONE',  ( 1.000000000000000000, 0.000000000000000000, 0.000000000000000000 ) ) ;
#9910=VERTEX_POINT ( 'NONE', #11180 ) ;
#9911=ORIENTED_EDGE ( 'NONE', *, *, #10448, .F. ) ;
#9927=ORIENTED_EDGE ( 'NONE', *, *, #39600, .T. ) ;
#9928=CIRCLE ( 'NONE', #14021, 2.000000000000001776 ) ;
#9932=PLANE ( 'NONE',  #41906 ) ;
#9937=VECTOR ( 'NONE', #35011, 1000.000000000000000 ) ;
#9941=FACE_BOUND ( 'NONE', #37580, .T. ) ;
#9945=CARTESIAN_POINT ( 'NONE',  ( 0.000000000000000000, 175.0000000000000284, 350.0000000000002274 ) ) ;
#9957=CARTESIAN_POINT ( 'NONE',  ( 349.9999999999999432, -164.9999999999999432, 355.9999999999997726 ) ) ;
#9961=AXIS2_PLACEMENT_3D ( 'NONE', #14523, #48874, #30175 ) ;
#9965=VERTEX_POINT ( 'NONE', #43226 ) ;
#9972=VERTEX_POINT ( 'NONE', #39644 ) ;
#9973=CARTESIAN_POINT ( 'NONE',  ( 181.0000000000000284, 2.775557561562891351E-14, -111.0000000000001563 ) ) ;
#9975=CARTESIAN_POINT ( 'NONE',  ( 168.9999999999999716, -93.49999999999997158, -115.0000000000001563 ) ) ;
#9978=CYLINDRICAL_SURFACE ( 'NONE', #13472, 4.000000000000003553 ) ;
#9984=DIRECTION ( 'NONE',  ( 1.000000000000000000, 0.000000000000000000, 0.000000000000000000 ) ) ;
#9997=ORIENTED_EDGE ( 'NONE', *, *, #3987, .F. ) ;
#10002=MECHANICAL_DESIGN_GEOMETRIC_PRESENTATION_REPRESENTATION('',(#46960),#16568);
#10003=EDGE_LOOP ( 'NONE', ( #12347, #29026, #40817, #10752, #8995, #46287, #43627, #35979 ) ) ;
#10006=EDGE_CURVE ( 'NONE', #7917, #9972, #43474, .T. ) ;
#10016=CARTESIAN_POINT ( 'NONE',  ( 344.0000000000000000, 174.9999999999996589, -344.0000000000002842 ) ) ;
#10021=CARTESIAN_POINT ( 'NONE',  ( 356.0000000000001137, 183.0000000000000284, 357.9999999999998295 ) ) ;
#10023=DIRECTION ( 'NONE',  ( 1.860490536778032451E-50, 0.000000000000000000, -1.000000000000000000 ) ) ;
#10028=AXIS2_PLACEMENT_3D ( 'NONE', #44974, #21396, #45475 ) ;
#10032=ORIENTED_EDGE ( 'NONE', *, *, #3320, .T. ) ;
#10038=VECTOR ( 'NONE', #45235, 1000.000000000000000 ) ;
#10044=ORIENTED_EDGE ( 'NONE', *, *, #8013, .T. ) ;
#10049=FACE_OUTER_BOUND ( 'NONE', #30015, .T. ) ;
#10054=DIRECTION ( 'NONE',  ( 0.000000000000000000, 5.664403186863042467E-17, 1.000000000000000000 ) ) ;
#10055=DIRECTION ( 'NONE',  ( 1.132880637372608740E-16, 4.718402560806925739E-50, 1.000000000000000000 ) ) ;
#10061=DIRECTION ( 'NONE',  ( -7.793956916774525800E-48, 0.000000000000000000, -1.000000000000000000 ) ) ;
#10062=DIRECTION ( 'NONE',  ( -1.000000000000000000, 4.996003610813203446E-16, -1.033975765691284410E-24 ) ) ;
#10063=VECTOR ( 'NONE', #9780, 1000.000000000000000 ) ;
#10064=CARTESIAN_POINT ( 'NONE',  ( 358.3431457505076310, -164.9999999999999432, 339.9999999999998295 ) ) ;
#10066=CARTESIAN_POINT ( 'NONE',  ( 0.000000000000000000, 181.0000000000000284, -344.0000000000001705 ) ) ;
#10077=DIRECTION ( 'NONE',  ( 0.000000000000000000, 0.000000000000000000, -1.000000000000000000 ) ) ;
#10080=DIRECTION ( 'NONE',  ( 0.000000000000000000, 1.000000000000000000, 0.000000000000000000 ) ) ;
#10082=VECTOR ( 'NONE', #31039, 1000.000000000000000 ) ;
#10097=DIRECTION ( 'NONE',  ( 0.000000000000000000, 1.000000000000000000, 0.000000000000000000 ) ) ;
#10102=DIRECTION ( 'NONE',  ( -0.000000000000000000, -6.123233995736766036E-17, 1.000000000000000000 ) ) ;
#10104=FACE_OUTER_BOUND ( 'NONE', #20894, .T. ) ;
#10108=VERTEX_POINT ( 'NONE', #3721 ) ;
#10109=VECTOR ( 'NONE', #15907, 1000.000000000000000 ) ;
#10118=FACE_OUTER_BOUND ( 'NONE', #44471, .T. ) ;
#10119=ORIENTED_EDGE ( 'NONE', *, *, #31508, .T. ) ;
#10122=DIRECTION ( 'NONE',  ( 0.000000000000000000, -1.544785076050074834E-48, -1.000000000000000000 ) ) ;
#10125=PLANE ( 'NONE',  #3076 ) ;
#10135=EDGE_CURVE ( 'NONE', #16798, #5037, #23489, .T. ) ;
#10136=LINE ( 'NONE', #45257, #35449 ) ;
#10138=AXIS2_PLACEMENT_3D ( 'NONE', #29397, #10153, #30415 ) ;
#10149=EDGE_CURVE ( 'NONE', #50401, #11765, #18491, .T. ) ;
#10150=DIRECTION ( 'NONE',  ( 0.000000000000000000, 0.000000000000000000, -1.000000000000000000 ) ) ;
#10153=DIRECTION ( 'NONE',  ( 0.000000000000000000, 0.000000000000000000, -1.000000000000000000 ) ) ;
#10154=CARTESIAN_POINT ( 'NONE',  ( 349.9999999999999432, -166.9999999999999432, 343.9999999999997726 ) ) ;
#10155=ORIENTED_EDGE ( 'NONE', *, *, #21122, .F. ) ;
#10157=ORIENTED_EDGE ( 'NONE', *, *, #31822, .T. ) ;
#10161=EDGE_LOOP ( 'NONE', ( #50373, #5305, #21441, #23555 ) ) ;
#10163=DIRECTION ( 'NONE',  ( 3.172065745548403743E-16, 1.000000000000000000, 0.000000000000000000 ) ) ;
#10169=EDGE_CURVE ( 'NONE', #38591, #28471, #28844, .T. ) ;
#10170=CARTESIAN_POINT ( 'NONE',  ( 164.9999999999999716, -168.9999999999999432, -350.0000000000001705 ) ) ;
#10172=CARTESIAN_POINT ( 'NONE',  ( 168.9999999999999716, -93.49999999999998579, -340.0000000000001137 ) ) ;
#10174=ORIENTED_EDGE ( 'NONE', *, *, #19751, .T. ) ;
#10176=DIRECTION ( 'NONE',  ( -0.000000000000000000, -1.000000000000000000, -0.000000000000000000 ) ) ;
#10178=( NAMED_UNIT ( * ) SI_UNIT ( $, .STERADIAN. ) SOLID_ANGLE_UNIT ( ) );
#10181=LINE ( 'NONE', #37156, #48316 ) ;
#10185=ADVANCED_FACE ( 'NONE', ( #4984, #28342 ), #9842, .T. ) ;
#10196=DIRECTION ( 'NONE',  ( 6.203854594147707562E-25, -2.067951531382569187E-25, 1.000000000000000000 ) ) ;
#10199=CARTESIAN_POINT ( 'NONE',  ( 356.0000000000002842, -165.0000000000001137, -110.0000000000002132 ) ) ;
#10204=AXIS2_PLACEMENT_3D ( 'NONE', #26408, #25410, #49211 ) ;
#10211=CARTESIAN_POINT ( 'NONE',  ( 164.9999999999999716, -272.5000000000000000, -98.99999999999990052 ) ) ;
#10212=CIRCLE ( 'NONE', #27432, 4.000000000000003553 ) ;
#10213=ORIENTED_EDGE ( 'NONE', *, *, #47118, .F. ) ;
#10214=PLANE ( 'NONE',  #45141 ) ;
#10215=CARTESIAN_POINT ( 'NONE',  ( 349.9999999999999432, -180.9999999999999716, 339.9999999999997726 ) ) ;
#10221=ORIENTED_EDGE ( 'NONE', *, *, #16836, .T. ) ;
#10223=CIRCLE ( 'NONE', #38111, 2.000000000000001776 ) ;
#10224=CYLINDRICAL_SURFACE ( 'NONE', #37752, 4.000000000000003553 ) ;
#10234=LINE ( 'NONE', #47989, #47863 ) ;
#10237=VECTOR ( 'NONE', #30736, 1000.000000000000000 ) ;
#10238=VERTEX_POINT ( 'NONE', #22653 ) ;
#10254=DIRECTION ( 'NONE',  ( -1.000000000000000000, -0.000000000000000000, -0.000000000000000000 ) ) ;
#10257=CARTESIAN_POINT ( 'NONE',  ( 350.0000000000000000, -168.9999999999999432, -340.0000000000001705 ) ) ;
#10278=VECTOR ( 'NONE', #30203, 1000.000000000000000 ) ;
#10288=ORIENTED_EDGE ( 'NONE', *, *, #14234, .F. ) ;
#10289=CARTESIAN_POINT ( 'NONE',  ( 356.0000000000002274, 183.0000000000000284, -358.0000000000001705 ) ) ;
#10290=CARTESIAN_POINT ( 'NONE',  ( 344.0000000000000568, 165.0000000000000000, 339.9999999999998295 ) ) ;
#10294=LINE ( 'NONE', #26440, #46984 ) ;
#10299=VECTOR ( 'NONE', #40692, 1000.000000000000000 ) ;
#10302=EDGE_CURVE ( 'NONE', #15862, #11298, #2881, .T. ) ;
#10304=LINE ( 'NONE', #25964, #12511 ) ;
#10307=EDGE_CURVE ( 'NONE', #37848, #49781, #10362, .T. ) ;
#10310=DIRECTION ( 'NONE',  ( 0.000000000000000000, -2.265761274745217480E-16, 1.000000000000000000 ) ) ;
#10311=CARTESIAN_POINT ( 'NONE',  ( 181.0000000000000284, -182.9999999999999716, -115.0000000000001279 ) ) ;
#10313=DIRECTION ( 'NONE',  ( -1.000000000000000000, 0.000000000000000000, -0.000000000000000000 ) ) ;
#10314=CARTESIAN_POINT ( 'NONE',  ( 343.9999999999999432, 185.0000000000002558, -360.0000000000003411 ) ) ;
#10315=ADVANCED_FACE ( 'NONE', ( #45210 ), #18282, .F. ) ;
#10319=ORIENTED_EDGE ( 'NONE', *, *, #31508, .F. ) ;
#10321=VECTOR ( 'NONE', #13755, 1000.000000000000000 ) ;
#10324=CARTESIAN_POINT ( 'NONE',  ( 350.0000000000000000, 169.0000000000000000, -356.0000000000002274 ) ) ;
#10328=CARTESIAN_POINT ( 'NONE',  ( 350.0000000000001137, 181.0000000000000284, 341.9999999999997726 ) ) ;
#10331=MECHANICAL_DESIGN_GEOMETRIC_PRESENTATION_REPRESENTATION('',(#29995),#2125);
#10336=VECTOR ( 'NONE', #47689, 1000.000000000000000 ) ;
#10344=DIRECTION ( 'NONE',  ( -1.587271980518778491E-16, 5.169878828456422968E-26, 1.000000000000000000 ) ) ;
#10355=ORIENTED_EDGE ( 'NONE', *, *, #12681, .T. ) ;
#10361=ORIENTED_EDGE ( 'NONE', *, *, #4911, .T. ) ;
#10362=LINE ( 'NONE', #34473, #21842 ) ;
#10364=VECTOR ( 'NONE', #22973, 1000.000000000000000 ) ;
#10392=FACE_OUTER_BOUND ( 'NONE', #27905, .T. ) ;
#10401=CARTESIAN_POINT ( 'NONE',  ( 350.0000000000000000, -164.9999999999999432, -360.0000000000002274 ) ) ;
#10413=CARTESIAN_POINT ( 'NONE',  ( 185.0000000000000000, -184.9999999999999716, -356.0000000000014211 ) ) ;
#10426=CYLINDRICAL_SURFACE ( 'NONE', #38281, 2.000000000000001776 ) ;
#10427=CARTESIAN_POINT ( 'NONE',  ( 166.9999999999999716, -272.5000000000000000, -99.00000000000014211 ) ) ;
#10428=CARTESIAN_POINT ( 'NONE',  ( 355.9999999999999432, -185.0000000000002558, -360.0000000000003411 ) ) ;
#10432=( BOUNDED_CURVE ( )  B_SPLINE_CURVE ( 3, ( #48959, #29519, #45135, #10021 ),
 .UNSPECIFIED., .F., .F. ) 
 B_SPLINE_CURVE_WITH_KNOTS ( ( 4, 4 ),
 ( 1.570796326794883235, 3.141592653589794004 ),
 .UNSPECIFIED. ) 
 CURVE ( )  GEOMETRIC_REPRESENTATION_ITEM ( )  RATIONAL_B_SPLINE_CURVE ( ( 1.000000000000000000, 0.8047378541243617178, 0.8047378541243617178, 1.000000000000000000 ) ) 
 REPRESENTATION_ITEM ( '' )  );
#10435=ORIENTED_EDGE ( 'NONE', *, *, #19414, .F. ) ;
#10439=CARTESIAN_POINT ( 'NONE',  ( 166.9999999999999716, 165.0000000000000000, -344.0000000000001137 ) ) ;
#10440=DIRECTION ( 'NONE',  ( 0.000000000000000000, 0.000000000000000000, 1.000000000000000000 ) ) ;
#10448=EDGE_CURVE ( 'NONE', #25186, #17816, #38585, .T. ) ;
#10452=EDGE_LOOP ( 'NONE', ( #23340, #5444, #17413, #39603 ) ) ;
#10453=CARTESIAN_POINT ( 'NONE',  ( 350.0000000000001137, 183.0000000000000284, 355.9999999999997726 ) ) ;
#10456=EDGE_CURVE ( 'NONE', #28373, #19760, #19051, .T. ) ;
#10460=CYLINDRICAL_SURFACE ( 'NONE', #37135, 4.000000000000003553 ) ;
#10462=LINE ( 'NONE', #13544, #39327 ) ;
#10465=CARTESIAN_POINT ( 'NONE',  ( 350.0000000000000000, 175.0000000000000568, -350.0000000000001705 ) ) ;
#10466=CARTESIAN_POINT ( 'NONE',  ( 340.0000000000000568, 169.0000000000000000, 343.9999999999997726 ) ) ;
#10475=FACE_OUTER_BOUND ( 'NONE', #45479, .T. ) ;
#10496=ADVANCED_FACE ( 'NONE', ( #20579 ), #16729, .F. ) ;
#10504=ORIENTED_EDGE ( 'NONE', *, *, #6745, .F. ) ;
#10512=CARTESIAN_POINT ( 'NONE',  ( -5.000000000000000000, -184.7999999999999545, 340.1999999999997044 ) ) ;
#10520=ORIENTED_EDGE ( 'NONE', *, *, #44350, .T. ) ;
#10521=EDGE_CURVE ( 'NONE', #48821, #17870, #33162, .T. ) ;
#10524=ADVANCED_FACE ( 'NONE', ( #48742 ), #48488, .F. ) ;
#10527=CLOSED_SHELL ( 'NONE', ( #1724, #30696, #21741, #34122, #49410, #6815, #41560, #14250, #8115, #11460, #24630, #23401, #29705, #29430, #40561, #49652, #39784, #46766 ) ) ;
#10528=ORIENTED_EDGE ( 'NONE', *, *, #18636, .F. ) ;
#10529=EDGE_CURVE ( 'NONE', #31210, #33108, #34976, .T. ) ;
#10534=DIRECTION ( 'NONE',  ( 6.203854594147707562E-25, -2.067951531382569187E-25, 1.000000000000000000 ) ) ;
#10535=DIRECTION ( 'NONE',  ( 1.132880637372608740E-16, 4.718402560806925739E-50, 1.000000000000000000 ) ) ;
#10536=ORIENTED_EDGE ( 'NONE', *, *, #3239, .T. ) ;
#10537=VERTEX_POINT ( 'NONE', #32905 ) ;
#10546=ORIENTED_EDGE ( 'NONE', *, *, #21182, .F. ) ;
#10556=AXIS2_PLACEMENT_3D ( 'NONE', #3603, #46162, #18233 ) ;
#10557=( NAMED_UNIT ( * ) PLANE_ANGLE_UNIT ( ) SI_UNIT ( $, .RADIAN. ) );
#10558=ADVANCED_FACE ( 'NONE', ( #13128, #39853 ), #24945, .T. ) ;
#10561=ORIENTED_EDGE ( 'NONE', *, *, #50415, .F. ) ;
#10567=CARTESIAN_POINT ( 'NONE',  ( 168.9999999999999716, -268.4999999999999432, -339.9999999999998863 ) ) ;
#10568=FACE_OUTER_BOUND ( 'NONE', #17572, .T. ) ;
#10575=CARTESIAN_POINT ( 'NONE',  ( 349.9999999999999432, -180.9999999999999716, 357.9999999999997726 ) ) ;
#10581=CARTESIAN_POINT ( 'NONE',  ( 181.0000000000000000, -254.4999999999999432, -339.9999999999998863 ) ) ;
#10583=EDGE_CURVE ( 'NONE', #19479, #35494, #5679, .T. ) ;
#10586=EDGE_CURVE ( 'NONE', #43944, #40512, #6950, .T. ) ;
#10587=CIRCLE ( 'NONE', #17151, 4.000000000000003553 ) ;
#10588=EDGE_CURVE ( 'NONE', #28991, #218, #30058, .T. ) ;
#10594=DIRECTION ( 'NONE',  ( 0.000000000000000000, -1.000000000000000000, 2.537652627714642000E-15 ) ) ;
#10595=CIRCLE ( 'NONE', #5687, 2.000000000000001776 ) ;
#10596=FACE_OUTER_BOUND ( 'NONE', #45122, .T. ) ;
#10597=CIRCLE ( 'NONE', #11408, 4.000000000000003553 ) ;
#10599=ORIENTED_EDGE ( 'NONE', *, *, #25378, .F. ) ;
#10601=CARTESIAN_POINT ( 'NONE',  ( 339.9999999999999432, 169.0000000000000000, -344.0000000000001705 ) ) ;
#10612=DIRECTION ( 'NONE',  ( 1.000000000000000000, 0.000000000000000000, -0.000000000000000000 ) ) ;
#10615=EDGE_LOOP ( 'NONE', ( #21316, #23122, #48569, #41107 ) ) ;
#10619=CARTESIAN_POINT ( 'NONE',  ( 359.9999999999999432, -174.9999999999999432, 355.9999999999998295 ) ) ;
#10624=VECTOR ( 'NONE', #9701, 1000.000000000000000 ) ;
#10643=CARTESIAN_POINT ( 'NONE',  ( 339.9999999999999432, -180.9999999999999716, -344.0000000000001705 ) ) ;
#10656=AXIS2_PLACEMENT_3D ( 'NONE', #33843, #25883, #2522 ) ;
#10665=ORIENTED_EDGE ( 'NONE', *, *, #25201, .T. ) ;
#10670=FACE_OUTER_BOUND ( 'NONE', #31781, .T. ) ;
#10671=DIRECTION ( 'NONE',  ( 0.000000000000000000, -1.000000000000000000, 0.000000000000000000 ) ) ;
#10673=VECTOR ( 'NONE', #8220, 1000.000000000000000 ) ;
#10675=CARTESIAN_POINT ( 'NONE',  ( 0.000000000000000000, 175.0000000000000284, -346.2500000000002274 ) ) ;
#10683=ORIENTED_EDGE ( 'NONE', *, *, #8964, .T. ) ;
#10696=AXIS2_PLACEMENT_3D ( 'NONE', #30735, #50161, #38689 ) ;
#10697=CARTESIAN_POINT ( 'NONE',  ( 185.0000000000000284, -174.9999999999999716, -111.0000000000001563 ) ) ;
#10698=EDGE_LOOP ( 'NONE', ( #28094, #3684, #21917, #40204 ) ) ;
#10703=FACE_OUTER_BOUND ( 'NONE', #46615, .T. ) ;
#10707=ORIENTED_EDGE ( 'NONE', *, *, #13656, .F. ) ;
#10709=EDGE_CURVE ( 'NONE', #29620, #40413, #23490, .T. ) ;
#10712=VERTEX_POINT ( 'NONE', #42086 ) ;
#10719=DIRECTION ( 'NONE',  ( -0.000000000000000000, -0.000000000000000000, 1.000000000000000000 ) ) ;
#10738=( BOUNDED_CURVE ( )  B_SPLINE_CURVE ( 3, ( #32737, #37370, #24793, #501 ),
 .UNSPECIFIED., .F., .F. ) 
 B_SPLINE_CURVE_WITH_KNOTS ( ( 4, 4 ),
 ( 3.169317492284500903E-16, 1.570796326794903663 ),
 .UNSPECIFIED. ) 
 CURVE ( )  GEOMETRIC_REPRESENTATION_ITEM ( )  RATIONAL_B_SPLINE_CURVE ( ( 1.000000000000000000, 0.8047378541243634942, 0.8047378541243634942, 1.000000000000000000 ) ) 
 REPRESENTATION_ITEM ( '' )  );
#10749=CARTESIAN_POINT ( 'NONE',  ( 350.0000000000000000, -166.9999999999999432, -356.0000000000002274 ) ) ;
#10752=ORIENTED_EDGE ( 'NONE', *, *, #12170, .F. ) ;
#10756=DIRECTION ( 'NONE',  ( 0.000000000000000000, 0.000000000000000000, -1.000000000000000000 ) ) ;
#10759=DIRECTION ( 'NONE',  ( -1.000000000000000000, 0.000000000000000000, 0.000000000000000000 ) ) ;
#10761=VECTOR ( 'NONE', #2897, 1000.000000000000000 ) ;
#10767=ADVANCED_FACE ( 'NONE', ( #38522 ), #12072, .F. ) ;
#10769=ORIENTED_EDGE ( 'NONE', *, *, #37161, .T. ) ;
#10773=CARTESIAN_POINT ( 'NONE',  ( 339.9999999999998863, -181.0000000000001990, -356.0000000000003411 ) ) ;
#10781=EDGE_CURVE ( 'NONE', #48255, #13701, #19762, .T. ) ;
#10784=CARTESIAN_POINT ( 'NONE',  ( 183.0000000000000000, 6.000000000000060396, 339.9999999999998295 ) ) ;
#10785=CARTESIAN_POINT ( 'NONE',  ( 169.0000000000000000, -174.9999999999999716, -97.00000000000014211 ) ) ;
#10789=LINE ( 'NONE', #50242, #42099 ) ;
#10791=ORIENTED_EDGE ( 'NONE', *, *, #23813, .T. ) ;
#10794=DIRECTION ( 'NONE',  ( 1.942330104924128867E-32, 0.000000000000000000, 1.000000000000000000 ) ) ;
#10796=VERTEX_POINT ( 'NONE', #19495 ) ;
#10803=EDGE_CURVE ( 'NONE', #18563, #21707, #7720, .T. ) ;
#10806=CARTESIAN_POINT ( 'NONE',  ( 350.0000000000001137, 165.0000000000000000, 343.9999999999997726 ) ) ;
#10808=EDGE_CURVE ( 'NONE', #8324, #14373, #11050, .T. ) ;
#10809=ADVANCED_FACE ( 'NONE', ( #23359 ), #42587, .T. ) ;
#10822=DIRECTION ( 'NONE',  ( -0.000000000000000000, -0.000000000000000000, 1.000000000000000000 ) ) ;
#10824=PLANE ( 'NONE',  #29868 ) ;
#10832=ORIENTED_EDGE ( 'NONE', *, *, #40011, .F. ) ;
#10834=VECTOR ( 'NONE', #28609, 1000.000000000000000 ) ;
#10835=LINE ( 'NONE', #31370, #20438 ) ;
#10844=VERTEX_POINT ( 'NONE', #46667 ) ;
#10860=DIRECTION ( 'NONE',  ( 0.000000000000000000, 1.000000000000000000, -2.537652627714642000E-15 ) ) ;
#10861=EDGE_LOOP ( 'NONE', ( #49701, #30502, #32988, #7346 ) ) ;
#10863=CARTESIAN_POINT ( 'NONE',  ( 358.0000000000000000, -169.0000000000001137, -349.9999999999998863 ) ) ;
#10864=DIRECTION ( 'NONE',  ( 0.000000000000000000, 5.664403186863042467E-17, 1.000000000000000000 ) ) ;
#10867=EDGE_CURVE ( 'NONE', #16553, #32197, #21876, .T. ) ;
#10869=ORIENTED_EDGE ( 'NONE', *, *, #28043, .T. ) ;
#10872=VECTOR ( 'NONE', #23058, 1000.000000000000000 ) ;
#10874=EDGE_CURVE ( 'NONE', #43954, #3318, #36187, .T. ) ;
#10875=ORIENTED_EDGE ( 'NONE', *, *, #37487, .F. ) ;
#10877=ORIENTED_EDGE ( 'NONE', *, *, #46137, .T. ) ;
#10886=VECTOR ( 'NONE', #16522, 1000.000000000000000 ) ;
#10895=CYLINDRICAL_SURFACE ( 'NONE', #49494, 4.000000000000003553 ) ;
#10896=CARTESIAN_POINT ( 'NONE',  ( -5.000000000000000000, 184.8000000000000114, 340.1999999999997044 ) ) ;
#10899=LINE ( 'NONE', #2690, #27128 ) ;
#10913=VECTOR ( 'NONE', #22440, 1000.000000000000000 ) ;
#10916=LINE ( 'NONE', #46284, #37240 ) ;
#10920=ORIENTED_EDGE ( 'NONE', *, *, #23584, .T. ) ;
#10926=CARTESIAN_POINT ( 'NONE',  ( 181.0000000000000000, 175.0000000000000284, -360.0000000000001705 ) ) ;
#10932=LINE ( 'NONE', #26591, #2501 ) ;
#10936=VERTEX_POINT ( 'NONE', #4624 ) ;
#10937=ORIENTED_EDGE ( 'NONE', *, *, #23023, .T. ) ;
#10949=VECTOR ( 'NONE', #30200, 1000.000000000000000 ) ;
#10952=DIRECTION ( 'NONE',  ( 0.000000000000000000, -1.000000000000000000, 0.000000000000000000 ) ) ;
#10963=VECTOR ( 'NONE', #42927, 1000.000000000000000 ) ;
#10968=CARTESIAN_POINT ( 'NONE',  ( 0.000000000000000000, -180.9999999999999716, -358.0000000000002274 ) ) ;
#10969=DIRECTION ( 'NONE',  ( -1.586032880504786307E-16, 1.654361225106055350E-24, -1.000000000000000000 ) ) ;
#10973=( LENGTH_UNIT ( ) NAMED_UNIT ( * ) SI_UNIT ( .MILLI., .METRE. ) );
#10974=ORIENTED_EDGE ( 'NONE', *, *, #10709, .T. ) ;
#10975=VERTEX_POINT ( 'NONE', #41030 ) ;
#10976=EDGE_CURVE ( 'NONE', #17617, #15072, #20222, .T. ) ;
#10980=AXIS2_PLACEMENT_3D ( 'NONE', #9973, #13310, #48172 ) ;
#10985=LINE ( 'NONE', #38213, #28435 ) ;
#10986=VERTEX_POINT ( 'NONE', #5874 ) ;
#10990=DIRECTION ( 'NONE',  ( -1.586032880504786307E-16, 1.654361225106055350E-24, -1.000000000000000000 ) ) ;
#10994=DIRECTION ( 'NONE',  ( 0.000000000000000000, 0.000000000000000000, 1.000000000000000000 ) ) ;
#11001=ORIENTED_EDGE ( 'NONE', *, *, #933, .F. ) ;
#11002=DIRECTION ( 'NONE',  ( 0.000000000000000000, 1.000000000000000000, 0.000000000000000000 ) ) ;
#11012=ORIENTED_EDGE ( 'NONE', *, *, #41707, .T. ) ;
#11030=ORIENTED_EDGE ( 'NONE', *, *, #1749, .T. ) ;
#11035=( BOUNDED_CURVE ( )  B_SPLINE_CURVE ( 3, ( #4422, #16226, #47483, #15455 ),
 .UNSPECIFIED., .F., .F. ) 
 B_SPLINE_CURVE_WITH_KNOTS ( ( 4, 4 ),
 ( 3.141592653590070672, 4.712388980384703885 ),
 .UNSPECIFIED. ) 
 CURVE ( )  GEOMETRIC_REPRESENTATION_ITEM ( )  RATIONAL_B_SPLINE_CURVE ( ( 1.000000000000000000, 0.8047378541244271100, 0.8047378541244271100, 1.000000000000000000 ) ) 
 REPRESENTATION_ITEM ( '' )  );
#11040=VERTEX_POINT ( 'NONE', #25635 ) ;
#11042=DIRECTION ( 'NONE',  ( 0.000000000000000000, 2.537652627714642000E-15, 1.000000000000000000 ) ) ;
#11049=ORIENTED_EDGE ( 'NONE', *, *, #19864, .T. ) ;
#11050=LINE ( 'NONE', #31587, #5416 ) ;
#11052=VERTEX_POINT ( 'NONE', #44845 ) ;
#11053=LINE ( 'NONE', #34420, #25112 ) ;
#11056=ORIENTED_EDGE ( 'NONE', *, *, #22216, .T. ) ;
#11058=DIRECTION ( 'NONE',  ( -0.000000000000000000, -1.000000000000000000, -0.000000000000000000 ) ) ;
#11066=CARTESIAN_POINT ( 'NONE',  ( 358.0000000000000000, -169.0000000000001137, -344.0000000000002842 ) ) ;
#11067=EDGE_CURVE ( 'NONE', #17053, #50485, #30896, .T. ) ;
#11070=EDGE_CURVE ( 'NONE', #18711, #4028, #26780, .T. ) ;
#11084=EDGE_CURVE ( 'NONE', #20395, #20947, #15381, .T. ) ;
#11089=STYLED_ITEM('',(#50747),#22493);
#11094=VERTEX_POINT ( 'NONE', #18167 ) ;
#11095=LINE ( 'NONE', #41889, #39375 ) ;
#11096=CARTESIAN_POINT ( 'NONE',  ( 339.9999999999999432, -168.9999999999999432, -358.0000000000002274 ) ) ;
#11097=EDGE_CURVE ( 'NONE', #41339, #10712, #14577, .T. ) ;
#11103=EDGE_CURVE ( 'NONE', #20217, #17284, #50702, .T. ) ;
#11109=EDGE_CURVE ( 'NONE', #9910, #8725, #14831, .T. ) ;
#11117=ORIENTED_EDGE ( 'NONE', *, *, #24960, .T. ) ;
#11120=CARTESIAN_POINT ( 'NONE',  ( 4.999999999999999112, 175.0000000000000284, -350.0000000000002274 ) ) ;
#11122=ORIENTED_EDGE ( 'NONE', *, *, #6120, .F. ) ;
#11125=VECTOR ( 'NONE', #13095, 1000.000000000000000 ) ;
#11126=CARTESIAN_POINT ( 'NONE',  ( 166.9999999999999716, -256.4999999999999432, -349.9999999999999432 ) ) ;
#11130=AXIS2_PLACEMENT_3D ( 'NONE', #39726, #7654, #3527 ) ;
#11132=VERTEX_POINT ( 'NONE', #27148 ) ;
#11133=EDGE_CURVE ( 'NONE', #27742, #49858, #10985, .T. ) ;
#11136=ORIENTED_EDGE ( 'NONE', *, *, #32928, .F. ) ;
#11144=EDGE_CURVE ( 'NONE', #24745, #48433, #34346, .T. ) ;
#11145=VECTOR ( 'NONE', #21959, 1000.000000000000000 ) ;
#11153=ORIENTED_EDGE ( 'NONE', *, *, #50000, .T. ) ;
#11156=LINE ( 'NONE', #27051, #8914 ) ;
#11180=CARTESIAN_POINT ( 'NONE',  ( 360.0000000000001137, 169.0000000000000000, 343.9999999999998295 ) ) ;
#11183=DIRECTION ( 'NONE',  ( 0.000000000000000000, 0.000000000000000000, -1.000000000000000000 ) ) ;
#11185=ORIENTED_EDGE ( 'NONE', *, *, #3918, .T. ) ;
#11189=LINE ( 'NONE', #7328, #15267 ) ;
#11192=VERTEX_POINT ( 'NONE', #48366 ) ;
#11193=CARTESIAN_POINT ( 'NONE',  ( 0.000000000000000000, -180.9999999999999716, -342.0000000000001705 ) ) ;
#11194=DIRECTION ( 'NONE',  ( 0.000000000000000000, 0.000000000000000000, -1.000000000000000000 ) ) ;
#11201=ORIENTED_EDGE ( 'NONE', *, *, #49342, .T. ) ;
#11203=EDGE_LOOP ( 'NONE', ( #20133, #11503, #38606, #31756, #11153, #29546, #36713, #32702 ) ) ;
#11204=CARTESIAN_POINT ( 'NONE',  ( 0.000000000000000000, 167.0000000000000000, 355.9999999999997726 ) ) ;
#11208=ORIENTED_EDGE ( 'NONE', *, *, #39641, .T. ) ;
#11209=ORIENTED_EDGE ( 'NONE', *, *, #34056, .F. ) ;
#11213=LINE ( 'NONE', #22492, #12998 ) ;
#11216=LINE ( 'NONE', #14538, #27591 ) ;
#11224=ORIENTED_EDGE ( 'NONE', *, *, #25597, .F. ) ;
#11228=CARTESIAN_POINT ( 'NONE',  ( 344.0000000000000000, 167.0000000000001990, -342.0000000000002842 ) ) ;
#11230=EDGE_CURVE ( 'NONE', #18563, #28991, #19942, .T. ) ;
#11231=VECTOR ( 'NONE', #46299, 1000.000000000000000 ) ;
#11232=DIRECTION ( 'NONE',  ( -1.000000000000000000, 0.000000000000000000, -1.612977847700450206E-50 ) ) ;
#11234=LINE ( 'NONE', #14815, #23082 ) ;
#11236=DIRECTION ( 'NONE',  ( 1.000000000000000000, 0.000000000000000000, -4.758098676964956461E-16 ) ) ;
#11249=DIRECTION ( 'NONE',  ( 0.000000000000000000, -0.000000000000000000, 1.000000000000000000 ) ) ;
#11250=EDGE_CURVE ( 'NONE', #40512, #18367, #43546, .T. ) ;
#11254=CARTESIAN_POINT ( 'NONE',  ( 349.9999999999999432, -180.9999999999999716, 357.9999999999997726 ) ) ;
#11256=PLANE ( 'NONE',  #17746 ) ;
#11258=ORIENTED_EDGE ( 'NONE', *, *, #25879, .T. ) ;
#11259=EDGE_LOOP ( 'NONE', ( #18527, #35353, #15772, #36057 ) ) ;
#11263=ORIENTED_EDGE ( 'NONE', *, *, #15820, .F. ) ;
#11266=DIRECTION ( 'NONE',  ( 0.000000000000000000, 5.664403186863042467E-17, 1.000000000000000000 ) ) ;
#11269=PLANE ( 'NONE',  #47894 ) ;
#11270=DIRECTION ( 'NONE',  ( -1.000000000000000000, 0.000000000000000000, 1.860490536778032451E-50 ) ) ;
#11274=EDGE_CURVE ( 'NONE', #30452, #24759, #35876, .T. ) ;
#11276=DIRECTION ( 'NONE',  ( 0.000000000000000000, 0.000000000000000000, 1.000000000000000000 ) ) ;
#11277=CARTESIAN_POINT ( 'NONE',  ( 181.0000000000000000, -270.4999999999999432, -349.9999999999999432 ) ) ;
#11278=( BOUNDED_CURVE ( )  B_SPLINE_CURVE ( 3, ( #6313, #41708, #21955, #2696 ),
 .UNSPECIFIED., .F., .F. ) 
 B_SPLINE_CURVE_WITH_KNOTS ( ( 4, 4 ),
 ( 3.141592653589793116, 4.712388980384689674 ),
 .UNSPECIFIED. ) 
 CURVE ( )  GEOMETRIC_REPRESENTATION_ITEM ( )  RATIONAL_B_SPLINE_CURVE ( ( 1.000000000000000000, 0.8047378541243649375, 0.8047378541243649375, 1.000000000000000000 ) ) 
 REPRESENTATION_ITEM ( '' )  );
#11280=DIRECTION ( 'NONE',  ( 3.172065745548403743E-16, 1.000000000000000000, 0.000000000000000000 ) ) ;
#11282=FACE_OUTER_BOUND ( 'NONE', #29594, .T. ) ;
#11287=ORIENTED_EDGE ( 'NONE', *, *, #44046, .F. ) ;
#11288=DIRECTION ( 'NONE',  ( -0.000000000000000000, -1.000000000000000000, 2.537652627714643577E-15 ) ) ;
#11292=DIRECTION ( 'NONE',  ( 0.000000000000000000, -1.000000000000000000, 0.000000000000000000 ) ) ;
#11297=AXIS2_PLACEMENT_3D ( 'NONE', #21730, #17632, #41740 ) ;
#11298=VERTEX_POINT ( 'NONE', #20966 ) ;
#11302=CARTESIAN_POINT ( 'NONE',  ( 340.0000000000000568, 181.0000000000000284, 343.9999999999997726 ) ) ;
#11306=EDGE_LOOP ( 'NONE', ( #441, #4479, #2873, #38032 ) ) ;
#11309=LINE ( 'NONE', #48554, #23117 ) ;
#11313=VERTEX_POINT ( 'NONE', #28418 ) ;
#11314=CARTESIAN_POINT ( 'NONE',  ( 169.0000000000000284, 175.0000000000000284, 343.9999999999998863 ) ) ;
#11322=ORIENTED_EDGE ( 'NONE', *, *, #18621, .F. ) ;
#11335=LINE ( 'NONE', #35211, #42964 ) ;
#11337=ORIENTED_EDGE ( 'NONE', *, *, #34666, .T. ) ;
#11342=( NAMED_UNIT ( * ) SI_UNIT ( $, .STERADIAN. ) SOLID_ANGLE_UNIT ( ) );
#11351=DIRECTION ( 'NONE',  ( 1.132880637372608740E-16, 4.718402560806925739E-50, 1.000000000000000000 ) ) ;
#11352=DIRECTION ( 'NONE',  ( -1.000000000000000000, -0.000000000000000000, -0.000000000000000000 ) ) ;
#11353=ORIENTED_EDGE ( 'NONE', *, *, #22820, .T. ) ;
#11354=DIRECTION ( 'NONE',  ( -1.000000000000000000, 0.000000000000000000, 0.000000000000000000 ) ) ;
#11356=CARTESIAN_POINT ( 'NONE',  ( 181.0000000000000000, -182.9999999999999716, -340.0000000000001137 ) ) ;
#11363=ORIENTED_EDGE ( 'NONE', *, *, #32837, .F. ) ;
#11366=CARTESIAN_POINT ( 'NONE',  ( 344.0000000000000000, 185.0000000000000284, -360.0000000000002274 ) ) ;
#11368=EDGE_LOOP ( 'NONE', ( #2819, #29190, #47311, #38314 ) ) ;
#11370=ORIENTED_EDGE ( 'NONE', *, *, #44123, .F. ) ;
#11374=LINE ( 'NONE', #2895, #45514 ) ;
#11376=DIRECTION ( 'NONE',  ( -4.758098676964956461E-16, -1.000000000000000000, 0.000000000000000000 ) ) ;
#11379=ORIENTED_EDGE ( 'NONE', *, *, #38427, .F. ) ;
#11381=CARTESIAN_POINT ( 'NONE',  ( 356.0000000000001137, 185.0000000000000284, 359.9999999999998295 ) ) ;
#11399=CARTESIAN_POINT ( 'NONE',  ( 168.9999999999999716, -272.4999999999999432, -355.9999999999999432 ) ) ;
#11403=CARTESIAN_POINT ( 'NONE',  ( 166.9999999999999716, -81.49999999999997158, -340.0000000000001137 ) ) ;
#11408=AXIS2_PLACEMENT_3D ( 'NONE', #2502, #41502, #37928 ) ;
#11409=CARTESIAN_POINT ( 'NONE',  ( 357.9999999999999432, 174.9999999999996589, -356.0000000000003411 ) ) ;
#11410=EDGE_CURVE ( 'NONE', #24755, #35217, #2408, .T. ) ;
#11411=DIRECTION ( 'NONE',  ( 0.000000000000000000, -1.000000000000000000, -3.186989995019654210E-49 ) ) ;
#11412=ORIENTED_EDGE ( 'NONE', *, *, #48984, .F. ) ;
#11417=CARTESIAN_POINT ( 'NONE',  ( 181.0000000000000284, -180.9999999999999716, -115.0000000000001279 ) ) ;
#11426=VERTEX_POINT ( 'NONE', #22164 ) ;
#11429=LINE ( 'NONE', #35559, #3615 ) ;
#11433=ORIENTED_EDGE ( 'NONE', *, *, #10588, .T. ) ;
#11436=VECTOR ( 'NONE', #8208, 1000.000000000000000 ) ;
#11446=DIRECTION ( 'NONE',  ( 1.000000000000000000, -4.758098676964957447E-16, -1.586032892321651989E-16 ) ) ;
#11447=AXIS2_PLACEMENT_3D ( 'NONE', #29299, #36770, #1600 ) ;
#11454=DIRECTION ( 'NONE',  ( 1.000000000000000000, -4.758098676964957447E-16, 2.958228394578795584E-31 ) ) ;
#11457=ADVANCED_FACE ( 'NONE', ( #26273 ), #34230, .F. ) ;
#11460=ADVANCED_FACE ( 'NONE', ( #26517 ), #3150, .F. ) ;
#11462=EDGE_CURVE ( 'NONE', #39156, #26957, #16241, .T. ) ;
#11471=AXIS2_PLACEMENT_3D ( 'NONE', #36568, #23982, #15765 ) ;
#11475=EDGE_CURVE ( 'NONE', #29839, #25245, #3668, .T. ) ;
#11479=CYLINDRICAL_SURFACE ( 'NONE', #10696, 2.000000000000001776 ) ;
#11492=VERTEX_POINT ( 'NONE', #50575 ) ;
#11496=EDGE_CURVE ( 'NONE', #46434, #3051, #16165, .T. ) ;
#11497=( BOUNDED_CURVE ( )  B_SPLINE_CURVE ( 3, ( #8686, #48880, #34052, #33799 ),
 .UNSPECIFIED., .F., .F. ) 
 B_SPLINE_CURVE_WITH_KNOTS ( ( 4, 4 ),
 ( 6.280369834734837385E-16, 1.570796326794924758 ),
 .UNSPECIFIED. ) 
 CURVE ( )  GEOMETRIC_REPRESENTATION_ITEM ( )  RATIONAL_B_SPLINE_CURVE ( ( 1.000000000000000000, 0.8047378541243583872, 0.8047378541243583872, 1.000000000000000000 ) ) 
 REPRESENTATION_ITEM ( '' )  );
#11499=ORIENTED_EDGE ( 'NONE', *, *, #35251, .F. ) ;
#11501=CARTESIAN_POINT ( 'NONE',  ( 350.0000000000001137, 169.0000000000000000, 359.9999999999997726 ) ) ;
#11502=DIRECTION ( 'NONE',  ( 1.000000000000000000, 0.000000000000000000, -1.586032892321651989E-16 ) ) ;
#11503=ORIENTED_EDGE ( 'NONE', *, *, #15272, .T. ) ;
#11505=CARTESIAN_POINT ( 'NONE',  ( 349.9999999999999432, -182.9999999999999716, 355.9999999999997726 ) ) ;
#11506=EDGE_LOOP ( 'NONE', ( #31069, #11799, #8027, #12826, #39281, #42263, #9530, #8528 ) ) ;
#11519=LINE ( 'NONE', #27172, #21071 ) ;
#11523=CARTESIAN_POINT ( 'NONE',  ( -5.000000000000000000, 165.2000000000000171, -340.2000000000001592 ) ) ;
#11526=DIRECTION ( 'NONE',  ( 0.000000000000000000, 0.000000000000000000, -1.000000000000000000 ) ) ;
#11530=VECTOR ( 'NONE', #7951, 1000.000000000000000 ) ;
#11545=VERTEX_POINT ( 'NONE', #4695 ) ;
#11548=CARTESIAN_POINT ( 'NONE',  ( 0.000000000000000000, 169.0000000000000000, 359.9999999999997726 ) ) ;
#11550=CARTESIAN_POINT ( 'NONE',  ( -5.000000000000000000, 165.2000000000000171, 340.1999999999997044 ) ) ;
#11551=CARTESIAN_POINT ( 'NONE',  ( 4.999999999999999112, -175.0000000000000284, -350.0000000000002274 ) ) ;
#11553=( NAMED_UNIT ( * ) SI_UNIT ( $, .STERADIAN. ) SOLID_ANGLE_UNIT ( ) );
#11555=AXIS2_PLACEMENT_3D ( 'NONE', #22012, #29722, #34094 ) ;
#11568=DIRECTION ( 'NONE',  ( -1.586032892321652236E-16, -1.000000000000000000, -6.853681917100419162E-49 ) ) ;
#11572=ORIENTED_EDGE ( 'NONE', *, *, #3490, .F. ) ;
#11574=FACE_OUTER_BOUND ( 'NONE', #7403, .T. ) ;
#11576=PLANE ( 'NONE',  #1351 ) ;
#11579=DIRECTION ( 'NONE',  ( -4.759647537211363479E-16, 5.772796816983493182E-42, -1.000000000000000000 ) ) ;
#11580=EDGE_CURVE ( 'NONE', #19058, #15809, #18587, .T. ) ;
#11587=VERTEX_POINT ( 'NONE', #20585 ) ;
#11592=DIRECTION ( 'NONE',  ( 3.172065745548403743E-16, 1.000000000000000000, 0.000000000000000000 ) ) ;
#11600=VECTOR ( 'NONE', #49654, 1000.000000000000000 ) ;
#11617=DIRECTION ( 'NONE',  ( 1.000000000000000000, 0.000000000000000000, 0.000000000000000000 ) ) ;
#11619=UNCERTAINTY_MEASURE_WITH_UNIT (LENGTH_MEASURE( 1.000000000000000082E-05 ), #8724, 'distance_accuracy_value', 'NONE');
#11621=AXIS2_PLACEMENT_3D ( 'NONE', #17369, #9669, #6070 ) ;
#11622=EDGE_LOOP ( 'NONE', ( #10044, #17983, #47493, #42144 ) ) ;
#11623=EDGE_LOOP ( 'NONE', ( #21465, #30913, #28501, #21446 ) ) ;
#11625=CARTESIAN_POINT ( 'NONE',  ( 339.9999999999999432, -169.0000000000001137, -344.0000000000002842 ) ) ;
#11630=CARTESIAN_POINT ( 'NONE',  ( 358.0000000000000000, 165.0000000000000000, -106.0000000000001990 ) ) ;
#11634=EDGE_LOOP ( 'NONE', ( #6748, #7122, #27921, #204 ) ) ;
#11645=LINE ( 'NONE', #27298, #10963 ) ;
#11650=VERTEX_POINT ( 'NONE', #33168 ) ;
#11660=DIRECTION ( 'NONE',  ( 1.132880637372608740E-16, 4.718402560806925739E-50, 1.000000000000000000 ) ) ;
#11662=STYLED_ITEM('',(#50747),#38377);
#11665=DIRECTION ( 'NONE',  ( 0.000000000000000000, 0.000000000000000000, 1.000000000000000000 ) ) ;
#11669=VERTEX_POINT ( 'NONE', #40349 ) ;
#11671=DIRECTION ( 'NONE',  ( 0.000000000000000000, -0.000000000000000000, 1.000000000000000000 ) ) ;
#11678=VERTEX_POINT ( 'NONE', #25193 ) ;
#11682=DIRECTION ( 'NONE',  ( 0.000000000000000000, -1.000000000000000000, 2.537652627714643577E-15 ) ) ;
#11685=EDGE_LOOP ( 'NONE', ( #41933, #6386, #33913, #47716, #3158, #7138, #16904, #32036 ) ) ;
#11686=ORIENTED_EDGE ( 'NONE', *, *, #13992, .F. ) ;
#11688=CARTESIAN_POINT ( 'NONE',  ( -5.000000000000000000, 184.8000000000000114, -340.2000000000001592 ) ) ;
#11692=VECTOR ( 'NONE', #34199, 1000.000000000000000 ) ;
#11696=ORIENTED_EDGE ( 'NONE', *, *, #38792, .F. ) ;
#11697=PLANE ( 'NONE',  #5759 ) ;
#11700=UNCERTAINTY_MEASURE_WITH_UNIT (LENGTH_MEASURE( 1.000000000000000082E-05 ), #951, 'distance_accuracy_value', 'NONE');
#11702=ORIENTED_EDGE ( 'NONE', *, *, #48789, .T. ) ;
#11714=CARTESIAN_POINT ( 'NONE',  ( 343.9999999999999432, -185.0000000000001421, -360.0000000000003979 ) ) ;
#11722=EDGE_CURVE ( 'NONE', #22827, #1115, #37028, .T. ) ;
#11726=EDGE_LOOP ( 'NONE', ( #37971, #32681, #14504, #36088 ) ) ;
#11735=ORIENTED_EDGE ( 'NONE', *, *, #25201, .F. ) ;
#11738=ADVANCED_FACE ( 'NONE', ( #12882 ), #32395, .F. ) ;
#11741=ORIENTED_EDGE ( 'NONE', *, *, #37602, .T. ) ;
#11743=DIRECTION ( 'NONE',  ( 0.000000000000000000, -1.000000000000000000, -0.000000000000000000 ) ) ;
#11745=EDGE_CURVE ( 'NONE', #12553, #14822, #36077, .T. ) ;
#11752=ORIENTED_EDGE ( 'NONE', *, *, #20969, .T. ) ;
#11753=DIRECTION ( 'NONE',  ( 0.000000000000000000, 1.000000000000000000, 1.544785076050074834E-48 ) ) ;
#11758=CIRCLE ( 'NONE', #10138, 2.000000000000001776 ) ;
#11765=VERTEX_POINT ( 'NONE', #6444 ) ;
#11778=DIRECTION ( 'NONE',  ( 1.000000000000000000, 0.000000000000000000, 0.000000000000000000 ) ) ;
#11784=CIRCLE ( 'NONE', #33117, 2.000000000000001776 ) ;
#11799=ORIENTED_EDGE ( 'NONE', *, *, #12370, .T. ) ;
#11822=EDGE_CURVE ( 'NONE', #47056, #50485, #38286, .T. ) ;
#11823=VECTOR ( 'NONE', #8695, 1000.000000000000000 ) ;
#11827=ORIENTED_EDGE ( 'NONE', *, *, #15312, .F. ) ;
#11829=LINE ( 'NONE', #4636, #38255 ) ;
#11833=CARTESIAN_POINT ( 'NONE',  ( 343.9999999999999432, -181.0000000000001421, -349.9999999999998863 ) ) ;
#11839=CARTESIAN_POINT ( 'NONE',  ( 356.0000000000002274, 185.0000000000000284, -360.0000000000002274 ) ) ;
#11842=VERTEX_POINT ( 'NONE', #14908 ) ;
#11850=DIRECTION ( 'NONE',  ( 1.000000000000000000, 0.000000000000000000, 0.000000000000000000 ) ) ;
#11854=CARTESIAN_POINT ( 'NONE',  ( 181.0000000000000000, -95.49999999999998579, -350.0000000000001705 ) ) ;
#11858=EDGE_LOOP ( 'NONE', ( #27871, #26653, #48685, #31166, #11012, #843, #11337, #22832 ) ) ;
#11860=VECTOR ( 'NONE', #50207, 1000.000000000000000 ) ;
#11861=ORIENTED_EDGE ( 'NONE', *, *, #39399, .T. ) ;
#11862=DIRECTION ( 'NONE',  ( 0.000000000000000000, -2.265761274745217480E-16, 1.000000000000000000 ) ) ;
#11865=ORIENTED_EDGE ( 'NONE', *, *, #47561, .F. ) ;
#11874=LINE ( 'NONE', #19046, #42604 ) ;
#11877=ADVANCED_FACE ( 'NONE', ( #39282 ), #39540, .F. ) ;
#11878=ORIENTED_EDGE ( 'NONE', *, *, #47402, .F. ) ;
#11887=ORIENTED_EDGE ( 'NONE', *, *, #4642, .T. ) ;
#11891=DIRECTION ( 'NONE',  ( -1.000000000000000000, 0.000000000000000000, -1.612977847700450206E-50 ) ) ;
#11900=CARTESIAN_POINT ( 'NONE',  ( 357.1715728752537871, 183.0000000000000000, -358.0000000000001705 ) ) ;
#11910=FACE_OUTER_BOUND ( 'NONE', #21833, .T. ) ;
#11913=DIRECTION ( 'NONE',  ( -1.132880637372608740E-16, -4.718402560806925739E-50, -1.000000000000000000 ) ) ;
#11917=CARTESIAN_POINT ( 'NONE',  ( 5.551115123125782702E-14, -168.9999999999999432, 357.9999999999997726 ) ) ;
#11937=ORIENTED_EDGE ( 'NONE', *, *, #16528, .T. ) ;
#11948=CIRCLE ( 'NONE', #6190, 4.000000000000003553 ) ;
#11949=VERTEX_POINT ( 'NONE', #19248 ) ;
#11950=ORIENTED_EDGE ( 'NONE', *, *, #17102, .F. ) ;
#11952=ORIENTED_EDGE ( 'NONE', *, *, #1438, .F. ) ;
#11957=DIRECTION ( 'NONE',  ( 0.000000000000000000, 0.000000000000000000, 1.000000000000000000 ) ) ;
#11978=CARTESIAN_POINT ( 'NONE',  ( 349.9999999999999432, -168.9999999999999432, 357.9999999999997726 ) ) ;
#11982=AXIS2_PLACEMENT_3D ( 'NONE', #19512, #8500, #32095 ) ;
#11983=CARTESIAN_POINT ( 'NONE',  ( 0.000000000000000000, 165.0000000000000000, 355.9999999999997726 ) ) ;
#11986=AXIS2_PLACEMENT_3D ( 'NONE', #537, #46420, #23610 ) ;
#11987=EDGE_LOOP ( 'NONE', ( #23294, #24631, #43234, #31912 ) ) ;
#11999=FACE_OUTER_BOUND ( 'NONE', #44225, .T. ) ;
#12006=ADVANCED_FACE ( 'NONE', ( #3865 ), #42597, .F. ) ;
#12009=CARTESIAN_POINT ( 'NONE',  ( 185.0000000000000000, -5.999999999999950262, -340.0000000000001137 ) ) ;
#12011=CARTESIAN_POINT ( 'NONE',  ( 169.0000000000000000, -174.9999999999999716, -113.0000000000001563 ) ) ;
#12013=ORIENTED_EDGE ( 'NONE', *, *, #14300, .F. ) ;
#12015=DIRECTION ( 'NONE',  ( -1.586032880504786307E-16, 1.654361225106055350E-24, -1.000000000000000000 ) ) ;
#12025=AXIS2_PLACEMENT_3D ( 'NONE', #18799, #34483, #50061 ) ;
#12033=DIRECTION ( 'NONE',  ( -0.000000000000000000, 1.000000000000000000, 0.000000000000000000 ) ) ;
#12039=ADVANCED_FACE ( 'NONE', ( #46427 ), #38779, .T. ) ;
#12041=CARTESIAN_POINT ( 'NONE',  ( 181.0000000000000000, -184.9999999999999716, -350.0000000000001705 ) ) ;
#12046=FACE_OUTER_BOUND ( 'NONE', #2204, .T. ) ;
#12056=LINE ( 'NONE', #8, #2498 ) ;
#12058=ORIENTED_EDGE ( 'NONE', *, *, #4186, .F. ) ;
#12063=EDGE_CURVE ( 'NONE', #24745, #15166, #20773, .T. ) ;
#12065=CARTESIAN_POINT ( 'NONE',  ( 164.9999999999999716, -174.9999999999999716, -356.0000000000001705 ) ) ;
#12068=DIRECTION ( 'NONE',  ( 0.000000000000000000, 0.000000000000000000, -1.000000000000000000 ) ) ;
#12072=PLANE ( 'NONE',  #11986 ) ;
#12075=ORIENTED_EDGE ( 'NONE', *, *, #1922, .F. ) ;
#12076=VECTOR ( 'NONE', #19965, 1000.000000000000000 ) ;
#12086=( BOUNDED_CURVE ( )  B_SPLINE_CURVE ( 3, ( #39571, #39076, #30862, #46453 ),
 .UNSPECIFIED., .F., .F. ) 
 B_SPLINE_CURVE_WITH_KNOTS ( ( 4, 4 ),
 ( 4.712388980384689674, 6.283185307179586232 ),
 .UNSPECIFIED. ) 
 CURVE ( )  GEOMETRIC_REPRESENTATION_ITEM ( )  RATIONAL_B_SPLINE_CURVE ( ( 1.000000000000000000, 0.8047378541243649375, 0.8047378541243649375, 1.000000000000000000 ) ) 
 REPRESENTATION_ITEM ( '' )  );
#12088=ORIENTED_EDGE ( 'NONE', *, *, #29294, .T. ) ;
#12098=LINE ( 'NONE', #44376, #14662 ) ;
#12099=CARTESIAN_POINT ( 'NONE',  ( 183.0000000000000568, 175.0000000000000284, 343.9999999999998863 ) ) ;
#12103=DIRECTION ( 'NONE',  ( 0.000000000000000000, 2.537652627714642000E-15, 1.000000000000000000 ) ) ;
#12105=EDGE_CURVE ( 'NONE', #28712, #35844, #43869, .T. ) ;
#12107=EDGE_CURVE ( 'NONE', #48410, #34818, #6535, .T. ) ;
#12114=DIRECTION ( 'NONE',  ( -1.654361225106055350E-24, -1.654361225106055350E-24, 1.000000000000000000 ) ) ;
#12116=LINE ( 'NONE', #46705, #30266 ) ;
#12122=ORIENTED_EDGE ( 'NONE', *, *, #11580, .T. ) ;
#12131=AXIS2_PLACEMENT_3D ( 'NONE', #37855, #34502, #41168 ) ;
#12140=CARTESIAN_POINT ( 'NONE',  ( 181.0000000000000000, -272.5000000000000000, -98.99999999999990052 ) ) ;
#12143=ORIENTED_EDGE ( 'NONE', *, *, #16124, .F. ) ;
#12145=CARTESIAN_POINT ( 'NONE',  ( 183.0000000000000000, -164.9999999999999432, 343.9999999999998863 ) ) ;
#12151=DIRECTION ( 'NONE',  ( 0.000000000000000000, 5.664403186863042467E-17, 1.000000000000000000 ) ) ;
#12153=CARTESIAN_POINT ( 'NONE',  ( 356.0000000000000000, 167.0000000000001990, -342.0000000000002842 ) ) ;
#12155=ORIENTED_EDGE ( 'NONE', *, *, #24881, .T. ) ;
#12156=DIRECTION ( 'NONE',  ( -1.586032892321651989E-16, 3.736034562988530447E-32, -1.000000000000000000 ) ) ;
#12157=CARTESIAN_POINT ( 'NONE',  ( 0.000000000000000000, 181.0000000000000284, 343.9999999999997726 ) ) ;
#12166=EDGE_CURVE ( 'NONE', #39344, #19058, #13818, .T. ) ;
#12170=EDGE_CURVE ( 'NONE', #29662, #26951, #22035, .T. ) ;
#12174=EDGE_LOOP ( 'NONE', ( #1540, #15895, #18865, #33980, #35113, #27016, #11122, #35300 ) ) ;
#12177=CARTESIAN_POINT ( 'NONE',  ( 165.0000000000000000, -174.9999999999999716, -111.0000000000001563 ) ) ;
#12178=ORIENTED_EDGE ( 'NONE', *, *, #8691, .F. ) ;
#12181=LINE ( 'NONE', #46525, #4884 ) ;
#12182=CARTESIAN_POINT ( 'NONE',  ( 0.000000000000000000, 184.8000000000000114, -359.8000000000002387 ) ) ;
#12183=ORIENTED_EDGE ( 'NONE', *, *, #21794, .F. ) ;
#12198=DIRECTION ( 'NONE',  ( 1.000000000000000000, 0.000000000000000000, 7.793956916774525800E-48 ) ) ;
#12204=VERTEX_POINT ( 'NONE', #26139 ) ;
#12208=VECTOR ( 'NONE', #29378, 1000.000000000000000 ) ;
#12219=LINE ( 'NONE', #3235, #35746 ) ;
#12223=DIRECTION ( 'NONE',  ( 1.586032892321651989E-16, -8.666415220619855873E-32, 1.000000000000000000 ) ) ;
#12226=FACE_OUTER_BOUND ( 'NONE', #35569, .T. ) ;
#12237=DIRECTION ( 'NONE',  ( 7.793956916774525800E-48, 0.000000000000000000, 1.000000000000000000 ) ) ;
#12239=ORIENTED_EDGE ( 'NONE', *, *, #39309, .F. ) ;
#12242=VECTOR ( 'NONE', #4530, 1000.000000000000000 ) ;
#12244=VERTEX_POINT ( 'NONE', #37222 ) ;
#12246=CARTESIAN_POINT ( 'NONE',  ( 168.9999999999999716, -252.4999999999999432, -339.9999999999998863 ) ) ;
#12248=STYLED_ITEM('',(#50747),#4281);
#12253=DIRECTION ( 'NONE',  ( 0.000000000000000000, 0.000000000000000000, 1.000000000000000000 ) ) ;
#12257=ORIENTED_EDGE ( 'NONE', *, *, #33825, .F. ) ;
#12261=ORIENTED_EDGE ( 'NONE', *, *, #4808, .T. ) ;
#12265=CARTESIAN_POINT ( 'NONE',  ( 169.0000000000000000, -272.5000000000000000, -96.99999999999988631 ) ) ;
#12268=DIRECTION ( 'NONE',  ( 0.000000000000000000, 0.000000000000000000, -1.000000000000000000 ) ) ;
#12271=FACE_OUTER_BOUND ( 'NONE', #25143, .T. ) ;
#12272=PLANE ( 'NONE',  #7852 ) ;
#12276=CYLINDRICAL_SURFACE ( 'NONE', #7233, 4.000000000000003553 ) ;
#12278=FACE_OUTER_BOUND ( 'NONE', #38970, .T. ) ;
#12285=CARTESIAN_POINT ( 'NONE',  ( 339.9999999999999432, 169.0000000000000000, -344.0000000000001137 ) ) ;
#12301=VERTEX_POINT ( 'NONE', #17689 ) ;
#12303=CARTESIAN_POINT ( 'NONE',  ( 183.0000000000000000, -164.9999999999999432, 355.9999999999998863 ) ) ;
#12304=ORIENTED_EDGE ( 'NONE', *, *, #15856, .T. ) ;
#12308=EDGE_CURVE ( 'NONE', #37848, #23455, #32812, .T. ) ;
#12310=ORIENTED_EDGE ( 'NONE', *, *, #49933, .F. ) ;
#12311=DIRECTION ( 'NONE',  ( 0.000000000000000000, 1.000000000000000000, 0.000000000000000000 ) ) ;
#12313=VECTOR ( 'NONE', #6482, 1000.000000000000000 ) ;
#12314=ORIENTED_EDGE ( 'NONE', *, *, #13704, .F. ) ;
#12316=ORIENTED_EDGE ( 'NONE', *, *, #50105, .F. ) ;
#12320=VECTOR ( 'NONE', #8203, 1000.000000000000000 ) ;
#12323=CARTESIAN_POINT ( 'NONE',  ( 341.9999999999999432, -168.9999999999999147, 343.9999999999998295 ) ) ;
#12325=CARTESIAN_POINT ( 'NONE',  ( 350.0000000000000000, 185.0000000000000284, -344.0000000000001705 ) ) ;
#12330=ORIENTED_EDGE ( 'NONE', *, *, #14183, .T. ) ;
#12336=DIRECTION ( 'NONE',  ( 0.000000000000000000, -2.969158215481698263E-48, 1.000000000000000000 ) ) ;
#12340=EDGE_CURVE ( 'NONE', #25272, #5007, #22542, .T. ) ;
#12344=CARTESIAN_POINT ( 'NONE',  ( 339.9999999999998863, -166.9999999999999432, 343.9999999999997726 ) ) ;
#12347=ORIENTED_EDGE ( 'NONE', *, *, #24268, .F. ) ;
#12348=VECTOR ( 'NONE', #9703, 1000.000000000000000 ) ;
#12370=EDGE_CURVE ( 'NONE', #46883, #17305, #15863, .T. ) ;
#12375=ORIENTED_EDGE ( 'NONE', *, *, #18636, .T. ) ;
#12377=FACE_OUTER_BOUND ( 'NONE', #30112, .T. ) ;
#12384=DIRECTION ( 'NONE',  ( 4.758098676964954489E-16, 1.000000000000000000, 1.751623080406021339E-46 ) ) ;
#12385=VECTOR ( 'NONE', #47508, 1000.000000000000000 ) ;
#12386=DIRECTION ( 'NONE',  ( 1.000000000000000000, 0.000000000000000000, 0.000000000000000000 ) ) ;
#12387=ORIENTED_EDGE ( 'NONE', *, *, #23670, .F. ) ;
#12391=CARTESIAN_POINT ( 'NONE',  ( 5.551115123125782702E-14, -182.9999999999999716, 343.9999999999997726 ) ) ;
#12396=AXIS2_PLACEMENT_3D ( 'NONE', #45579, #2746, #18898 ) ;
#12414=CARTESIAN_POINT ( 'NONE',  ( 181.0000000000000000, 175.0000000000000284, -358.0000000000001705 ) ) ;
#12417=DIRECTION ( 'NONE',  ( 0.000000000000000000, 0.000000000000000000, -1.000000000000000000 ) ) ;
#12419=ORIENTED_EDGE ( 'NONE', *, *, #39681, .F. ) ;
#12427=EDGE_LOOP ( 'NONE', ( #846, #19104, #16504, #43224, #26453, #1469, #39989, #22761 ) ) ;
#12430=EDGE_CURVE ( 'NONE', #19251, #23733, #35280, .T. ) ;
#12432=ORIENTED_EDGE ( 'NONE', *, *, #21750, .F. ) ;
#12433=EDGE_LOOP ( 'NONE', ( #23272, #31365, #35067, #44053 ) ) ;
#12445=ORIENTED_EDGE ( 'NONE', *, *, #24038, .T. ) ;
#12447=ORIENTED_EDGE ( 'NONE', *, *, #21750, .T. ) ;
#12449=PLANE ( 'NONE',  #4960 ) ;
#12461=CYLINDRICAL_SURFACE ( 'NONE', #32809, 2.000000000000001776 ) ;
#12464=ORIENTED_EDGE ( 'NONE', *, *, #16810, .T. ) ;
#12466=FACE_OUTER_BOUND ( 'NONE', #11306, .T. ) ;
#12474=CARTESIAN_POINT ( 'NONE',  ( 183.0000000000000000, -184.9999999999999716, -356.0000000000001705 ) ) ;
#12484=ORIENTED_EDGE ( 'NONE', *, *, #31861, .T. ) ;
#12492=CYLINDRICAL_SURFACE ( 'NONE', #31154, 2.000000000000001776 ) ;
#12500=DIRECTION ( 'NONE',  ( -1.000000000000000000, 0.000000000000000000, -2.958228394578794270E-31 ) ) ;
#12501=EDGE_CURVE ( 'NONE', #13237, #7540, #49118, .T. ) ;
#12505=CARTESIAN_POINT ( 'NONE',  ( 168.9999999999999716, -272.4999999999999432, -355.9999999999999432 ) ) ;
#12507=ORIENTED_EDGE ( 'NONE', *, *, #47578, .F. ) ;
#12511=VECTOR ( 'NONE', #41093, 1000.000000000000000 ) ;
#12515=LINE ( 'NONE', #39992, #33815 ) ;
#12520=DIRECTION ( 'NONE',  ( 0.000000000000000000, 0.000000000000000000, 1.000000000000000000 ) ) ;
#12529=DIRECTION ( 'NONE',  ( 0.000000000000000000, -1.000000000000000000, 0.000000000000000000 ) ) ;
#12530=LINE ( 'NONE', #19469, #27307 ) ;
#12533=EDGE_CURVE ( 'NONE', #44854, #39344, #20218, .T. ) ;
#12534=( BOUNDED_CURVE ( )  B_SPLINE_CURVE ( 3, ( #27815, #8071, #117, #31419 ),
 .UNSPECIFIED., .F., .F. ) 
 B_SPLINE_CURVE_WITH_KNOTS ( ( 4, 4 ),
 ( 1.570796326794897002, 3.141592653589793560 ),
 .UNSPECIFIED. ) 
 CURVE ( )  GEOMETRIC_REPRESENTATION_ITEM ( )  RATIONAL_B_SPLINE_CURVE ( ( 1.000000000000000000, 0.8047378541243649375, 0.8047378541243649375, 1.000000000000000000 ) ) 
 REPRESENTATION_ITEM ( '' )  );
#12537=LINE ( 'NONE', #34905, #12320 ) ;
#12539=ORIENTED_EDGE ( 'NONE', *, *, #20259, .F. ) ;
#12541=DIRECTION ( 'NONE',  ( 1.000000000000000000, 0.000000000000000000, 0.000000000000000000 ) ) ;
#12545=FACE_OUTER_BOUND ( 'NONE', #14702, .T. ) ;
#12552=CARTESIAN_POINT ( 'NONE',  ( 181.0000000000000000, -184.9999999999999716, -340.0000000000001137 ) ) ;
#12553=VERTEX_POINT ( 'NONE', #8428 ) ;
#12555=DIRECTION ( 'NONE',  ( 1.000000000000000000, 0.000000000000000000, 7.793956916774525800E-48 ) ) ;
#12556=AXIS2_PLACEMENT_3D ( 'NONE', #7560, #19084, #34775 ) ;
#12560=STYLED_ITEM('',(#50747),#39637);
#12565=ORIENTED_EDGE ( 'NONE', *, *, #2492, .T. ) ;
#12568=CARTESIAN_POINT ( 'NONE',  ( 169.0000000000000284, 175.0000000000000284, 357.9999999999998863 ) ) ;
#12575=VECTOR ( 'NONE', #35081, 1000.000000000000000 ) ;
#12581=EDGE_LOOP ( 'NONE', ( #28517, #4103, #28912, #19218, #37639, #15913, #40112, #9769 ) ) ;
#12583=DIRECTION ( 'NONE',  ( 3.172065745548403743E-16, 1.000000000000000000, 0.000000000000000000 ) ) ;
#12586=AXIS2_PLACEMENT_3D ( 'NONE', #43914, #32129, #39335 ) ;
#12588=DIRECTION ( 'NONE',  ( 0.000000000000000000, 1.000000000000000000, 6.123233995736766036E-17 ) ) ;
#12595=LINE ( 'NONE', #59, #5966 ) ;
#12596=EDGE_CURVE ( 'NONE', #11052, #39773, #28696, .T. ) ;
#12603=LINE ( 'NONE', #9019, #40193 ) ;
#12610=DIRECTION ( 'NONE',  ( 1.860490536778032451E-50, 0.000000000000000000, -1.000000000000000000 ) ) ;
#12620=EDGE_LOOP ( 'NONE', ( #12991, #38558, #30169, #36581, #36706, #41099, #152, #47658 ) ) ;
#12623=AXIS2_PLACEMENT_3D ( 'NONE', #1342, #37019, #29287 ) ;
#12627=CARTESIAN_POINT ( 'NONE',  ( -5.000000000000000000, 165.2000000000000171, -359.8000000000002387 ) ) ;
#12635=EDGE_LOOP ( 'NONE', ( #14524, #27363, #36284, #34942, #141, #21201, #25703, #27988 ) ) ;
#12637=ORIENTED_EDGE ( 'NONE', *, *, #16431, .F. ) ;
#12639=( NAMED_UNIT ( * ) SI_UNIT ( $, .STERADIAN. ) SOLID_ANGLE_UNIT ( ) );
#12640=ADVANCED_FACE ( 'NONE', ( #38158 ), #18123, .F. ) ;
#12643=ORIENTED_EDGE ( 'NONE', *, *, #29778, .T. ) ;
#12645=ORIENTED_EDGE ( 'NONE', *, *, #23388, .F. ) ;
#12651=DIRECTION ( 'NONE',  ( 0.000000000000000000, 1.000000000000000000, 0.000000000000000000 ) ) ;
#12655=ORIENTED_EDGE ( 'NONE', *, *, #20197, .T. ) ;
#12656=DIRECTION ( 'NONE',  ( -3.172065784643302499E-16, -1.000000000000000000, 0.000000000000000000 ) ) ;
#12660=EDGE_CURVE ( 'NONE', #32832, #9482, #10181, .T. ) ;
#12661=EDGE_CURVE ( 'NONE', #23671, #21333, #6335, .T. ) ;
#12665=DIRECTION ( 'NONE',  ( 1.000000000000000000, 0.000000000000000000, 0.000000000000000000 ) ) ;
#12667=ORIENTED_EDGE ( 'NONE', *, *, #45529, .T. ) ;
#12669=EDGE_CURVE ( 'NONE', #3854, #8266, #14016, .T. ) ;
#12672=ORIENTED_EDGE ( 'NONE', *, *, #10808, .T. ) ;
#12674=DIRECTION ( 'NONE',  ( 0.000000000000000000, -1.000000000000000000, -3.186989995019654210E-49 ) ) ;
#12677=CARTESIAN_POINT ( 'NONE',  ( 181.0000000000000000, -164.9999999999999432, -340.0000000000001705 ) ) ;
#12679=ORIENTED_EDGE ( 'NONE', *, *, #18678, .T. ) ;
#12681=EDGE_CURVE ( 'NONE', #8852, #49105, #9862, .T. ) ;
#12684=AXIS2_PLACEMENT_3D ( 'NONE', #17409, #33576, #14307 ) ;
#12690=CARTESIAN_POINT ( 'NONE',  ( 166.9999999999999716, -272.4999999999999432, -343.9999999999987494 ) ) ;
#12692=CARTESIAN_POINT ( 'NONE',  ( 360.0000000000001137, 183.3431457505076594, 358.3431457505074604 ) ) ;
#12695=ORIENTED_EDGE ( 'NONE', *, *, #38597, .T. ) ;
#12707=ORIENTED_EDGE ( 'NONE', *, *, #43107, .F. ) ;
#12709=AXIS2_PLACEMENT_3D ( 'NONE', #42931, #3942, #111 ) ;
#12710=EDGE_CURVE ( 'NONE', #49781, #8266, #42236, .T. ) ;
#12715=CARTESIAN_POINT ( 'NONE',  ( 168.9999999999999716, -93.49999999999998579, -350.0000000000001705 ) ) ;
#12730=CIRCLE ( 'NONE', #43047, 4.000000000000003553 ) ;
#12733=ADVANCED_FACE ( 'NONE', ( #38407 ), #42723, .F. ) ;
#12734=ORIENTED_EDGE ( 'NONE', *, *, #44738, .T. ) ;
#12736=AXIS2_PLACEMENT_3D ( 'NONE', #2987, #18632, #22991 ) ;
#12742=DIRECTION ( 'NONE',  ( 0.000000000000000000, 0.000000000000000000, -1.000000000000000000 ) ) ;
#12745=ORIENTED_EDGE ( 'NONE', *, *, #30361, .T. ) ;
#12750=EDGE_LOOP ( 'NONE', ( #26872, #36251, #33828, #22671 ) ) ;
#12753=CYLINDRICAL_SURFACE ( 'NONE', #18365, 2.000000000000001776 ) ;
#12755=VERTEX_POINT ( 'NONE', #11204 ) ;
#12758=CARTESIAN_POINT ( 'NONE',  ( 339.9999999999999432, 175.0000000000000284, -106.0000000000001990 ) ) ;
#12762=ORIENTED_EDGE ( 'NONE', *, *, #20315, .T. ) ;
#12765=VERTEX_POINT ( 'NONE', #19394 ) ;
#12778=DIRECTION ( 'NONE',  ( 0.000000000000000000, -2.537652627714643577E-15, -1.000000000000000000 ) ) ;
#12786=UNCERTAINTY_MEASURE_WITH_UNIT (LENGTH_MEASURE( 1.000000000000000082E-05 ), #47510, 'distance_accuracy_value', 'NONE');
#12787=ADVANCED_FACE ( 'NONE', ( #49870 ), #11697, .F. ) ;
#12790=ORIENTED_EDGE ( 'NONE', *, *, #39821, .F. ) ;
#12791=CARTESIAN_POINT ( 'NONE',  ( 5.551115123125782702E-14, -180.9999999999999716, 343.9999999999997726 ) ) ;
#12796=EDGE_CURVE ( 'NONE', #38055, #48807, #10932, .T. ) ;
#12799=VECTOR ( 'NONE', #43484, 1000.000000000000000 ) ;
#12801=AXIS2_PLACEMENT_3D ( 'NONE', #38776, #7210, #15414 ) ;
#12803=ORIENTED_EDGE ( 'NONE', *, *, #27754, .F. ) ;
#12807=ADVANCED_FACE ( 'NONE', ( #35577 ), #20396, .F. ) ;
#12809=CARTESIAN_POINT ( 'NONE',  ( 185.0000000000000284, -174.9999999999999716, -111.0000000000001563 ) ) ;
#12811=ORIENTED_EDGE ( 'NONE', *, *, #38113, .T. ) ;
#12813=ORIENTED_EDGE ( 'NONE', *, *, #10169, .T. ) ;
#12826=ORIENTED_EDGE ( 'NONE', *, *, #23878, .T. ) ;
#12841=CARTESIAN_POINT ( 'NONE',  ( -5.000000000000000000, 165.2000000000000171, 340.1999999999997044 ) ) ;
#12847=DIRECTION ( 'NONE',  ( 1.000000000000000000, 0.000000000000000000, 0.000000000000000000 ) ) ;
#12852=CARTESIAN_POINT ( 'NONE',  ( 350.0000000000000000, -182.9999999999999716, -344.0000000000001705 ) ) ;
#12856=EDGE_CURVE ( 'NONE', #11949, #14610, #660, .T. ) ;
#12857=ADVANCED_FACE ( 'NONE', ( #20150 ), #12449, .T. ) ;
#12862=VERTEX_POINT ( 'NONE', #16562 ) ;
#12866=CARTESIAN_POINT ( 'NONE',  ( 344.0000000000000000, -165.0000000000001137, 340.0000000000000568 ) ) ;
#12868=ORIENTED_EDGE ( 'NONE', *, *, #13491, .T. ) ;
#12878=DIRECTION ( 'NONE',  ( 0.000000000000000000, -1.000000000000000000, -1.544785076050074834E-48 ) ) ;
#12881=ORIENTED_EDGE ( 'NONE', *, *, #14596, .T. ) ;
#12882=FACE_OUTER_BOUND ( 'NONE', #49322, .T. ) ;
#12883=CARTESIAN_POINT ( 'NONE',  ( 183.0000000000000000, -174.9999999999999716, -344.0000000000001137 ) ) ;
#12888=FACE_OUTER_BOUND ( 'NONE', #4674, .T. ) ;
#12892=ORIENTED_EDGE ( 'NONE', *, *, #8028, .T. ) ;
#12904=CARTESIAN_POINT ( 'NONE',  ( 344.0000000000000568, 167.0000000000000000, 341.9999999999998295 ) ) ;
#12907=ORIENTED_EDGE ( 'NONE', *, *, #46643, .F. ) ;
#12928=EDGE_CURVE ( 'NONE', #1045, #28535, #36996, .T. ) ;
#12935=LINE ( 'NONE', #28595, #19355 ) ;
#12937=ORIENTED_EDGE ( 'NONE', *, *, #48034, .F. ) ;
#12938=VERTEX_POINT ( 'NONE', #33379 ) ;
#12939=ORIENTED_EDGE ( 'NONE', *, *, #37161, .F. ) ;
#12940=EDGE_CURVE ( 'NONE', #40195, #34478, #20527, .T. ) ;
#12942=CARTESIAN_POINT ( 'NONE',  ( 0.000000000000000000, -168.9999999999999432, -344.0000000000001705 ) ) ;
#12955=DIRECTION ( 'NONE',  ( -1.586032892321652236E-16, -1.000000000000000000, -6.853681917100419162E-49 ) ) ;
#12964=AXIS2_PLACEMENT_3D ( 'NONE', #41686, #2683, #21941 ) ;
#12973=ADVANCED_FACE ( 'NONE', ( #37494 ), #14613, .T. ) ;
#12979=FACE_OUTER_BOUND ( 'NONE', #30678, .T. ) ;
#12981=ORIENTED_EDGE ( 'NONE', *, *, #29289, .F. ) ;
#12986=CARTESIAN_POINT ( 'NONE',  ( 181.0000000000000000, 175.0000000000000284, -342.0000000000001137 ) ) ;
#12987=ORIENTED_EDGE ( 'NONE', *, *, #50285, .F. ) ;
#12991=ORIENTED_EDGE ( 'NONE', *, *, #26219, .F. ) ;
#12992=DIRECTION ( 'NONE',  ( -1.000000000000000000, 0.000000000000000000, 1.860490536778032451E-50 ) ) ;
#12998=VECTOR ( 'NONE', #26602, 1000.000000000000000 ) ;
#13002=ADVANCED_FACE ( 'NONE', ( #23327, #7948 ), #38998, .T. ) ;
#13007=ORIENTED_EDGE ( 'NONE', *, *, #35263, .F. ) ;
#13008=VERTEX_POINT ( 'NONE', #46125 ) ;
#13011=ADVANCED_FACE ( 'NONE', ( #26922 ), #22564, .T. ) ;
#13012=EDGE_CURVE ( 'NONE', #31089, #3248, #15124, .T. ) ;
#13013=CYLINDRICAL_SURFACE ( 'NONE', #7854, 4.000000000000003553 ) ;
#13020=LINE ( 'NONE', #1988, #6663 ) ;
#13026=EDGE_CURVE ( 'NONE', #11765, #28419, #4089, .T. ) ;
#13033=DIRECTION ( 'NONE',  ( 0.000000000000000000, -0.000000000000000000, -1.000000000000000000 ) ) ;
#13040=AXIS2_PLACEMENT_3D ( 'NONE', #24737, #4724, #43961 ) ;
#13041=CARTESIAN_POINT ( 'NONE',  ( 350.0000000000001137, 169.0000000000000000, 357.9999999999997726 ) ) ;
#13044=LINE ( 'NONE', #1516, #22999 ) ;
#13051=DIRECTION ( 'NONE',  ( 0.000000000000000000, -2.265761274745217480E-16, 1.000000000000000000 ) ) ;
#13054=AXIS2_PLACEMENT_3D ( 'NONE', #17544, #32451, #4732 ) ;
#13058=ORIENTED_EDGE ( 'NONE', *, *, #43776, .F. ) ;
#13064=LINE ( 'NONE', #20766, #31345 ) ;
#13065=ADVANCED_FACE ( 'NONE', ( #12046 ), #38249, .F. ) ;
#13069=CARTESIAN_POINT ( 'NONE',  ( 356.0000000000000000, -167.0000000000001137, -342.0000000000002842 ) ) ;
#13075=CARTESIAN_POINT ( 'NONE',  ( 0.000000000000000000, 167.0000000000000000, 355.9999999999997726 ) ) ;
#13091=ORIENTED_EDGE ( 'NONE', *, *, #35251, .T. ) ;
#13095=DIRECTION ( 'NONE',  ( -1.000000000000000000, 0.000000000000000000, -2.958228394578794270E-31 ) ) ;
#13098=EDGE_LOOP ( 'NONE', ( #7952, #25814, #50368, #9303, #6205, #21528, #12745, #39807 ) ) ;
#13117=ORIENTED_EDGE ( 'NONE', *, *, #26154, .F. ) ;
#13118=DIRECTION ( 'NONE',  ( 1.860490536778032451E-50, 0.000000000000000000, -1.000000000000000000 ) ) ;
#13122=AXIS2_PLACEMENT_3D ( 'NONE', #6073, #29677, #37652 ) ;
#13128=FACE_BOUND ( 'NONE', #32439, .T. ) ;
#13130=EDGE_CURVE ( 'NONE', #24963, #41575, #38499, .T. ) ;
#13131=EDGE_LOOP ( 'NONE', ( #18873, #20759 ) ) ;
#13133=DIRECTION ( 'NONE',  ( 0.000000000000000000, -2.265761274745217480E-16, 1.000000000000000000 ) ) ;
#13134=CARTESIAN_POINT ( 'NONE',  ( 164.9999999999999716, -184.9999999999999716, -344.0000000000001137 ) ) ;
#13140=CARTESIAN_POINT ( 'NONE',  ( 356.0000000000000000, -167.0000000000001137, -342.0000000000002842 ) ) ;
#13144=EDGE_CURVE ( 'NONE', #31478, #16715, #48247, .T. ) ;
#13147=VERTEX_POINT ( 'NONE', #27944 ) ;
#13152=DIRECTION ( 'NONE',  ( 0.000000000000000000, 0.000000000000000000, -1.000000000000000000 ) ) ;
#13154=VERTEX_POINT ( 'NONE', #12285 ) ;
#13170=VECTOR ( 'NONE', #45389, 1000.000000000000000 ) ;
#13171=CARTESIAN_POINT ( 'NONE',  ( 181.0000000000000284, -174.9999999999999716, -111.0000000000001563 ) ) ;
#13172=( LENGTH_UNIT ( ) NAMED_UNIT ( * ) SI_UNIT ( .MILLI., .METRE. ) );
#13175=EDGE_LOOP ( 'NONE', ( #39247, #46129, #48068, #12987 ) ) ;
#13181=ORIENTED_EDGE ( 'NONE', *, *, #35712, .F. ) ;
#13186=EDGE_LOOP ( 'NONE', ( #45701, #22460, #23186, #5083 ) ) ;
#13191=AXIS2_PLACEMENT_3D ( 'NONE', #7279, #27294, #50587 ) ;
#13200=EDGE_LOOP ( 'NONE', ( #4740, #19371, #15664, #39710 ) ) ;
#13204=ORIENTED_EDGE ( 'NONE', *, *, #24409, .T. ) ;
#13208=CARTESIAN_POINT ( 'NONE',  ( 181.0000000000000000, -256.4999999999999432, -349.9999999999999432 ) ) ;
#13214=LINE ( 'NONE', #21413, #6989 ) ;
#13217=LINE ( 'NONE', #21170, #12208 ) ;
#13221=CARTESIAN_POINT ( 'NONE',  ( 168.9999999999999716, -164.9999999999999432, -115.0000000000001847 ) ) ;
#13222=VECTOR ( 'NONE', #10612, 1000.000000000000000 ) ;
#13225=CARTESIAN_POINT ( 'NONE',  ( 344.0000000000000568, 169.0000000000000000, 349.9999999999998295 ) ) ;
#13231=VERTEX_POINT ( 'NONE', #20740 ) ;
#13237=VERTEX_POINT ( 'NONE', #27690 ) ;
#13238=DIRECTION ( 'NONE',  ( 1.860490536778032451E-50, 0.000000000000000000, 1.000000000000000000 ) ) ;
#13242=ORIENTED_EDGE ( 'NONE', *, *, #37547, .T. ) ;
#13255=FACE_OUTER_BOUND ( 'NONE', #3109, .T. ) ;
#13266=EDGE_CURVE ( 'NONE', #14822, #29017, #39756, .T. ) ;
#13269=FACE_BOUND ( 'NONE', #39205, .T. ) ;
#13274=EDGE_CURVE ( 'NONE', #11426, #2228, #1753, .T. ) ;
#13276=CARTESIAN_POINT ( 'NONE',  ( 350.0000000000000000, -164.9999999999999432, 359.9999999999997726 ) ) ;
#13277=LINE ( 'NONE', #2245, #33092 ) ;
#13279=ORIENTED_EDGE ( 'NONE', *, *, #2969, .F. ) ;
#13286=MECHANICAL_DESIGN_GEOMETRIC_PRESENTATION_REPRESENTATION('',(#39544),#16668);
#13287=ADVANCED_FACE ( 'NONE', ( #25857, #5586 ), #21491, .T. ) ;
#13292=CARTESIAN_POINT ( 'NONE',  ( -5.000000000000000000, -184.7999999999999545, 359.7999999999997840 ) ) ;
#13294=EDGE_CURVE ( 'NONE', #35576, #18285, #10597, .T. ) ;
#13297=PLANE ( 'NONE',  #25179 ) ;
#13302=ORIENTED_EDGE ( 'NONE', *, *, #13978, .F. ) ;
#13304=VERTEX_POINT ( 'NONE', #6100 ) ;
#13307=VERTEX_POINT ( 'NONE', #21999 ) ;
#13308=DIRECTION ( 'NONE',  ( 0.000000000000000000, 0.000000000000000000, 1.000000000000000000 ) ) ;
#13310=DIRECTION ( 'NONE',  ( -0.000000000000000000, -1.000000000000000000, -0.000000000000000000 ) ) ;
#13311=VECTOR ( 'NONE', #23434, 1000.000000000000000 ) ;
#13321=VECTOR ( 'NONE', #23652, 1000.000000000000000 ) ;
#13323=ORIENTED_EDGE ( 'NONE', *, *, #3186, .T. ) ;
#13325=VECTOR ( 'NONE', #48943, 1000.000000000000000 ) ;
#13335=CARTESIAN_POINT ( 'NONE',  ( 181.0000000000000568, 175.0000000000000284, 339.9999999999998863 ) ) ;
#13336=CARTESIAN_POINT ( 'NONE',  ( 166.9999999999999716, -81.49999999999997158, -115.0000000000001563 ) ) ;
#13347=ORIENTED_EDGE ( 'NONE', *, *, #32223, .T. ) ;
#13352=EDGE_CURVE ( 'NONE', #46080, #46658, #17647, .T. ) ;
#13355=EDGE_CURVE ( 'NONE', #45423, #3850, #44822, .T. ) ;
#13361=AXIS2_PLACEMENT_3D ( 'NONE', #8766, #12336, #32106 ) ;
#13372=CARTESIAN_POINT ( 'NONE',  ( 344.0000000000000568, 167.0000000000000000, 341.9999999999998295 ) ) ;
#13377=VERTEX_POINT ( 'NONE', #18893 ) ;
#13392=ORIENTED_EDGE ( 'NONE', *, *, #18171, .F. ) ;
#13394=ORIENTED_EDGE ( 'NONE', *, *, #25238, .F. ) ;
#13400=ORIENTED_EDGE ( 'NONE', *, *, #17678, .T. ) ;
#13401=LINE ( 'NONE', #36787, #6199 ) ;
#13405=DIRECTION ( 'NONE',  ( -1.000000000000000000, 0.000000000000000000, 0.000000000000000000 ) ) ;
#13410=DIRECTION ( 'NONE',  ( 0.000000000000000000, 1.000000000000000000, 0.000000000000000000 ) ) ;
#13413=CARTESIAN_POINT ( 'NONE',  ( 341.9999999999999432, 174.9999999999996589, -356.0000000000003411 ) ) ;
#13420=VERTEX_POINT ( 'NONE', #23257 ) ;
#13422=VERTEX_POINT ( 'NONE', #46330 ) ;
#13425=LINE ( 'NONE', #40642, #37316 ) ;
#13428=ORIENTED_EDGE ( 'NONE', *, *, #3554, .F. ) ;
#13434=CARTESIAN_POINT ( 'NONE',  ( 339.9999999999998863, -180.9999999999999716, 339.9999999999997726 ) ) ;
#13441=EDGE_LOOP ( 'NONE', ( #26361, #45805, #41824, #40753 ) ) ;
#13443=CARTESIAN_POINT ( 'NONE',  ( 0.000000000000000000, 184.8000000000000114, -340.2000000000001592 ) ) ;
#13445=LINE ( 'NONE', #44967, #26310 ) ;
#13447=EDGE_LOOP ( 'NONE', ( #31735, #10288, #47367, #40265 ) ) ;
#13454=ORIENTED_EDGE ( 'NONE', *, *, #32507, .F. ) ;
#13470=FACE_OUTER_BOUND ( 'NONE', #9712, .T. ) ;
#13471=DIRECTION ( 'NONE',  ( 0.000000000000000000, 0.000000000000000000, 1.000000000000000000 ) ) ;
#13472=AXIS2_PLACEMENT_3D ( 'NONE', #28289, #43923, #8798 ) ;
#13483=CARTESIAN_POINT ( 'NONE',  ( 341.6568542494923690, 185.0000000000000568, -360.0000000000001705 ) ) ;
#13487=VECTOR ( 'NONE', #44997, 1000.000000000000000 ) ;
#13491=EDGE_CURVE ( 'NONE', #49245, #39424, #23780, .T. ) ;
#13494=ORIENTED_EDGE ( 'NONE', *, *, #12340, .T. ) ;
#13496=ORIENTED_EDGE ( 'NONE', *, *, #46870, .T. ) ;
#13498=CARTESIAN_POINT ( 'NONE',  ( 168.9999999999999716, -168.9999999999999432, -340.0000000000001137 ) ) ;
#13500=DIRECTION ( 'NONE',  ( 1.000000000000000000, 0.000000000000000000, 0.000000000000000000 ) ) ;
#13502=AXIS2_PLACEMENT_3D ( 'NONE', #8672, #11753, #12253 ) ;
#13503=ORIENTED_EDGE ( 'NONE', *, *, #7027, .F. ) ;
#13504=VERTEX_POINT ( 'NONE', #27637 ) ;
#13505=VECTOR ( 'NONE', #25587, 1000.000000000000000 ) ;
#13507=CARTESIAN_POINT ( 'NONE',  ( 356.0000000000000000, 175.0000000000000284, -110.0000000000002132 ) ) ;
#13511=LINE ( 'NONE', #44798, #24740 ) ;
#13513=( BOUNDED_CURVE ( )  B_SPLINE_CURVE ( 3, ( #36144, #26283, #21928, #33985 ),
 .UNSPECIFIED., .F., .F. ) 
 B_SPLINE_CURVE_WITH_KNOTS ( ( 4, 4 ),
 ( 5.551115123125777022E-14, 1.570796326794896558 ),
 .UNSPECIFIED. ) 
 CURVE ( )  GEOMETRIC_REPRESENTATION_ITEM ( )  RATIONAL_B_SPLINE_CURVE ( ( 1.000000000000000000, 0.8047378541243781491, 0.8047378541243781491, 1.000000000000000000 ) ) 
 REPRESENTATION_ITEM ( '' )  );
#13514=VERTEX_POINT ( 'NONE', #24039 ) ;
#13518=ORIENTED_EDGE ( 'NONE', *, *, #14196, .T. ) ;
#13519=EDGE_CURVE ( 'NONE', #46863, #19251, #945, .T. ) ;
#13526=CARTESIAN_POINT ( 'NONE',  ( 185.0000000000000000, -184.9999999999999716, -356.0000000000001705 ) ) ;
#13532=CARTESIAN_POINT ( 'NONE',  ( 183.0000000000000000, -81.50000000000000000, -340.0000000000001137 ) ) ;
#13535=VECTOR ( 'NONE', #36197, 1000.000000000000000 ) ;
#13537=CARTESIAN_POINT ( 'NONE',  ( 181.0000000000000284, -174.9999999999999716, -113.0000000000001563 ) ) ;
#13542=ORIENTED_EDGE ( 'NONE', *, *, #1102, .T. ) ;
#13544=CARTESIAN_POINT ( 'NONE',  ( 181.0000000000000284, 2.775557561562891351E-14, -97.00000000000014211 ) ) ;
#13548=LINE ( 'NONE', #21500, #49393 ) ;
#13556=ORIENTED_EDGE ( 'NONE', *, *, #27593, .F. ) ;
#13560=ORIENTED_EDGE ( 'NONE', *, *, #49690, .T. ) ;
#13565=AXIS2_PLACEMENT_3D ( 'NONE', #27569, #24220, #39882 ) ;
#13576=ORIENTED_EDGE ( 'NONE', *, *, #31226, .T. ) ;
#13579=ORIENTED_EDGE ( 'NONE', *, *, #9817, .F. ) ;
#13580=DIRECTION ( 'NONE',  ( 0.000000000000000000, 0.000000000000000000, 1.000000000000000000 ) ) ;
#13581=( BOUNDED_CURVE ( )  B_SPLINE_CURVE ( 3, ( #28514, #44139, #9011, #24665 ),
 .UNSPECIFIED., .F., .F. ) 
 B_SPLINE_CURVE_WITH_KNOTS ( ( 4, 4 ),
 ( 3.140184917367520258E-16, 1.570796326794896780 ),
 .UNSPECIFIED. ) 
 CURVE ( )  GEOMETRIC_REPRESENTATION_ITEM ( )  RATIONAL_B_SPLINE_CURVE ( ( 1.000000000000000000, 0.8047378541243649375, 0.8047378541243649375, 1.000000000000000000 ) ) 
 REPRESENTATION_ITEM ( '' )  );
#13582=PLANE ( 'NONE',  #15202 ) ;
#13586=VECTOR ( 'NONE', #33808, 1000.000000000000000 ) ;
#13590=DIRECTION ( 'NONE',  ( 1.000000000000000000, -1.331116318405244905E-23, -4.759647537211363479E-16 ) ) ;
#13591=EDGE_CURVE ( 'NONE', #20650, #28031, #8387, .T. ) ;
#13592=ADVANCED_FACE ( 'NONE', ( #16081 ), #16584, .F. ) ;
#13600=CARTESIAN_POINT ( 'NONE',  ( 168.9999999999999716, -252.5000000000000000, -114.9999999999999574 ) ) ;
#13607=DIRECTION ( 'NONE',  ( 2.220446049250312588E-16, 0.7071067811865475727, -0.7071067811865474617 ) ) ;
#13608=CARTESIAN_POINT ( 'NONE',  ( 168.9999999999999716, -272.4999999999999432, -343.9999999999999432 ) ) ;
#13609=EDGE_CURVE ( 'NONE', #28419, #33773, #28627, .T. ) ;
#13611=ADVANCED_FACE ( 'NONE', ( #12226 ), #43269, .F. ) ;
#13614=EDGE_CURVE ( 'NONE', #30474, #8581, #1449, .T. ) ;
#13616=VECTOR ( 'NONE', #29502, 1000.000000000000000 ) ;
#13617=ORIENTED_EDGE ( 'NONE', *, *, #2147, .F. ) ;
#13619=EDGE_CURVE ( 'NONE', #33463, #40720, #10587, .T. ) ;
#13634=EDGE_LOOP ( 'NONE', ( #8215, #41683, #12178, #21390, #14473, #45286, #8856, #43300 ) ) ;
#13639=ORIENTED_EDGE ( 'NONE', *, *, #18399, .T. ) ;
#13651=EDGE_CURVE ( 'NONE', #48972, #23500, #6305, .T. ) ;
#13652=ORIENTED_EDGE ( 'NONE', *, *, #10529, .T. ) ;
#13656=EDGE_CURVE ( 'NONE', #45648, #15688, #2387, .T. ) ;
#13658=CYLINDRICAL_SURFACE ( 'NONE', #40499, 4.000000000000003553 ) ;
#13663=DIRECTION ( 'NONE',  ( 1.860490536778032451E-50, 0.000000000000000000, -1.000000000000000000 ) ) ;
#13670=CARTESIAN_POINT ( 'NONE',  ( -5.000000000000000000, -165.1999999999999602, 340.1999999999997044 ) ) ;
#13674=CYLINDRICAL_SURFACE ( 'NONE', #25807, 2.000000000000001776 ) ;
#13675=PLANE ( 'NONE',  #36363 ) ;
#13677=ADVANCED_FACE ( 'NONE', ( #25289 ), #48846, .F. ) ;
#13679=ORIENTED_EDGE ( 'NONE', *, *, #13355, .F. ) ;
#13682=DIRECTION ( 'NONE',  ( 9.711650524620651178E-33, -1.223873602809432483E-48, 1.000000000000000000 ) ) ;
#13688=EDGE_CURVE ( 'NONE', #12938, #36125, #9888, .T. ) ;
#13692=DIRECTION ( 'NONE',  ( -5.473822126268816076E-48, 1.000000000000000000, 1.654361225106055350E-24 ) ) ;
#13696=PLANE ( 'NONE',  #24152 ) ;
#13697=LINE ( 'NONE', #48556, #25922 ) ;
#13699=ADVANCED_FACE ( 'NONE', ( #48336 ), #2198, .F. ) ;
#13701=VERTEX_POINT ( 'NONE', #324 ) ;
#13704=EDGE_CURVE ( 'NONE', #30746, #31478, #12116, .T. ) ;
#13705=EDGE_CURVE ( 'NONE', #3658, #21143, #12086, .T. ) ;
#13707=ORIENTED_EDGE ( 'NONE', *, *, #4065, .F. ) ;
#13713=EDGE_LOOP ( 'NONE', ( #37142, #10769, #31318, #42080 ) ) ;
#13715=CYLINDRICAL_SURFACE ( 'NONE', #32389, 2.000000000000001776 ) ;
#13718=EDGE_CURVE ( 'NONE', #43146, #35494, #26991, .T. ) ;
#13719=FACE_OUTER_BOUND ( 'NONE', #18003, .T. ) ;
#13722=CARTESIAN_POINT ( 'NONE',  ( 168.9999999999999716, -256.4999999999999432, -349.9999999999999432 ) ) ;
#13727=( BOUNDED_CURVE ( )  B_SPLINE_CURVE ( 3, ( #23899, #35467, #315, #15954 ),
 .UNSPECIFIED., .F., .F. ) 
 B_SPLINE_CURVE_WITH_KNOTS ( ( 4, 4 ),
 ( 3.141592653589793116, 4.712388980384700332 ),
 .UNSPECIFIED. ) 
 CURVE ( )  GEOMETRIC_REPRESENTATION_ITEM ( )  RATIONAL_B_SPLINE_CURVE ( ( 1.000000000000000000, 0.8047378541243626060, 0.8047378541243626060, 1.000000000000000000 ) ) 
 REPRESENTATION_ITEM ( '' )  );
#13732=FACE_OUTER_BOUND ( 'NONE', #41282, .T. ) ;
#13734=CARTESIAN_POINT ( 'NONE',  ( 181.0000000000000000, -268.5000000000000000, -114.9999999999999147 ) ) ;
#13739=DIRECTION ( 'NONE',  ( 0.000000000000000000, 1.000000000000000000, -1.544785076050074834E-48 ) ) ;
#13751=LINE ( 'NONE', #47862, #6882 ) ;
#13755=DIRECTION ( 'NONE',  ( 0.000000000000000000, -1.000000000000000000, -3.186989995019654210E-49 ) ) ;
#13761=CARTESIAN_POINT ( 'NONE',  ( 0.000000000000000000, -182.9999999999999716, -356.0000000000002274 ) ) ;
#13765=DIRECTION ( 'NONE',  ( 0.000000000000000000, 1.000000000000000000, 0.000000000000000000 ) ) ;
#13775=ADVANCED_FACE ( 'NONE', ( #7243, #46961 ), #34979, .T. ) ;
#13778=LINE ( 'NONE', #25851, #15402 ) ;
#13782=DIRECTION ( 'NONE',  ( 2.242130092700023170E-16, -0.7071067811865475727, 0.7071067811865474617 ) ) ;
#13796=ORIENTED_EDGE ( 'NONE', *, *, #39072, .T. ) ;
#13798=EDGE_CURVE ( 'NONE', #35927, #1398, #40923, .T. ) ;
#13799=PLANE ( 'NONE',  #11555 ) ;
#13800=AXIS2_PLACEMENT_3D ( 'NONE', #5972, #41380, #37311 ) ;
#13805=DIRECTION ( 'NONE',  ( 0.000000000000000000, -1.000000000000000000, -3.186989995019654210E-49 ) ) ;
#13814=LINE ( 'NONE', #5116, #19566 ) ;
#13815=EDGE_LOOP ( 'NONE', ( #28967, #4364, #1304, #13347 ) ) ;
#13818=LINE ( 'NONE', #45108, #49088 ) ;
#13825=FACE_OUTER_BOUND ( 'NONE', #695, .T. ) ;
#13829=ADVANCED_FACE ( 'NONE', ( #47714 ), #16707, .T. ) ;
#13836=CARTESIAN_POINT ( 'NONE',  ( 343.9999999999993747, 183.0000000000000568, 357.9999999999998295 ) ) ;
#13839=VECTOR ( 'NONE', #18681, 1000.000000000000000 ) ;
#13860=DIRECTION ( 'NONE',  ( 1.000000000000000000, 0.000000000000000000, -0.000000000000000000 ) ) ;
#13862=DIRECTION ( 'NONE',  ( -1.000000000000000000, 3.172065745548403743E-16, -1.587271980518778491E-16 ) ) ;
#13870=CIRCLE ( 'NONE', #39290, 2.000000000000001776 ) ;
#13882=FACE_OUTER_BOUND ( 'NONE', #25310, .T. ) ;
#13892=CARTESIAN_POINT ( 'NONE',  ( 356.0000000000000000, -164.9999999999999432, 339.9999999999998295 ) ) ;
#13902=DIRECTION ( 'NONE',  ( -1.000000000000000000, 0.000000000000000000, 0.000000000000000000 ) ) ;
#13904=ORIENTED_EDGE ( 'NONE', *, *, #14543, .F. ) ;
#13906=FACE_OUTER_BOUND ( 'NONE', #49585, .T. ) ;
#13907=LINE ( 'NONE', #20618, #40573 ) ;
#13910=CYLINDRICAL_SURFACE ( 'NONE', #42882, 2.000000000000001776 ) ;
#13913=ORIENTED_EDGE ( 'NONE', *, *, #12501, .F. ) ;
#13914=VECTOR ( 'NONE', #40982, 1000.000000000000000 ) ;
#13916=DIRECTION ( 'NONE',  ( -1.000000000000000000, 0.000000000000000000, -2.958228394578794270E-31 ) ) ;
#13922=EDGE_CURVE ( 'NONE', #48356, #49781, #20437, .T. ) ;
#13925=ORIENTED_EDGE ( 'NONE', *, *, #38250, .F. ) ;
#13928=ADVANCED_FACE ( 'NONE', ( #44146 ), #5155, .T. ) ;
#13940=DIRECTION ( 'NONE',  ( -1.000000000000000000, -0.000000000000000000, -0.000000000000000000 ) ) ;
#13948=VECTOR ( 'NONE', #31052, 1000.000000000000000 ) ;
#13952=SHAPE_REPRESENTATION ( 'frame_Default<As Machined>', ( #45486 ), #41416 ) ;
#13957=ORIENTED_EDGE ( 'NONE', *, *, #17476, .T. ) ;
#13960=VERTEX_POINT ( 'NONE', #3067 ) ;
#13968=CARTESIAN_POINT ( 'NONE',  ( 339.9999999999998863, -164.9999999999999432, 355.9999999999997726 ) ) ;
#13969=DIRECTION ( 'NONE',  ( 1.000000000000000000, 0.000000000000000000, 0.000000000000000000 ) ) ;
#13975=FACE_OUTER_BOUND ( 'NONE', #44771, .T. ) ;
#13978=EDGE_CURVE ( 'NONE', #47711, #25776, #4910, .T. ) ;
#13979=DIRECTION ( 'NONE',  ( 0.000000000000000000, 2.537652627714642000E-15, 1.000000000000000000 ) ) ;
#13982=AXIS2_PLACEMENT_3D ( 'NONE', #2705, #30162, #11183 ) ;
#13990=DIRECTION ( 'NONE',  ( 0.000000000000000000, 5.664403186863042467E-17, 1.000000000000000000 ) ) ;
#13992=EDGE_CURVE ( 'NONE', #15814, #18475, #38525, .T. ) ;
#14001=ORIENTED_EDGE ( 'NONE', *, *, #8762, .F. ) ;
#14007=PLANE ( 'NONE',  #38219 ) ;
#14013=DIRECTION ( 'NONE',  ( 3.172065745548403743E-16, 1.000000000000000000, 0.000000000000000000 ) ) ;
#14016=LINE ( 'NONE', #21978, #4919 ) ;
#14019=LINE ( 'NONE', #18126, #46159 ) ;
#14021=AXIS2_PLACEMENT_3D ( 'NONE', #34738, #46222, #3399 ) ;
#14023=DIRECTION ( 'NONE',  ( 2.958228394578793832E-31, 0.000000000000000000, 1.000000000000000000 ) ) ;
#14028=DIRECTION ( 'NONE',  ( 6.203854594147707562E-25, -2.067951531382569187E-25, 1.000000000000000000 ) ) ;
#14037=CARTESIAN_POINT ( 'NONE',  ( -5.000000000000000000, 165.2000000000000171, -340.2000000000001592 ) ) ;
#14038=CARTESIAN_POINT ( 'NONE',  ( 4.999999999999999112, -175.0000000000000284, -346.2500000000002274 ) ) ;
#14049=AXIS2_PLACEMENT_3D ( 'NONE', #34753, #50321, #31143 ) ;
#14051=EDGE_CURVE ( 'NONE', #11765, #27818, #39257, .T. ) ;
#14053=CYLINDRICAL_SURFACE ( 'NONE', #29014, 4.000000000000003553 ) ;
#14057=FACE_OUTER_BOUND ( 'NONE', #20290, .T. ) ;
#14058=EDGE_CURVE ( 'NONE', #27139, #46544, #46648, .T. ) ;
#14059=ORIENTED_EDGE ( 'NONE', *, *, #5640, .T. ) ;
#14066=FACE_OUTER_BOUND ( 'NONE', #35807, .T. ) ;
#14067=EDGE_CURVE ( 'NONE', #10796, #3283, #34909, .T. ) ;
#14068=VECTOR ( 'NONE', #31757, 1000.000000000000000 ) ;
#14069=CARTESIAN_POINT ( 'NONE',  ( 342.8284271247460993, 167.0000000000000284, -342.0000000000001705 ) ) ;
#14072=DIRECTION ( 'NONE',  ( -1.368455531567204171E-48, 1.000000000000000000, 2.265761274745217480E-16 ) ) ;
#14075=DIRECTION ( 'NONE',  ( -1.612977847700450206E-50, 0.000000000000000000, -1.000000000000000000 ) ) ;
#14078=ORIENTED_EDGE ( 'NONE', *, *, #39809, .F. ) ;
#14084=LINE ( 'NONE', #28746, #34460 ) ;
#14087=ORIENTED_EDGE ( 'NONE', *, *, #47491, .F. ) ;
#14090=AXIS2_PLACEMENT_3D ( 'NONE', #4385, #20026, #28493 ) ;
#14098=LINE ( 'NONE', #41310, #26519 ) ;
#14109=DIRECTION ( 'NONE',  ( 0.000000000000000000, 0.000000000000000000, 1.000000000000000000 ) ) ;
#14124=AXIS2_PLACEMENT_3D ( 'NONE', #46177, #6711, #14414 ) ;
#14133=EDGE_LOOP ( 'NONE', ( #19381, #6002, #40223, #11287 ) ) ;
#14138=CARTESIAN_POINT ( 'NONE',  ( 181.0000000000000000, -97.49999999999998579, -350.0000000000001705 ) ) ;
#14144=FACE_OUTER_BOUND ( 'NONE', #38958, .T. ) ;
#14147=FACE_OUTER_BOUND ( 'NONE', #2386, .T. ) ;
#14152=CARTESIAN_POINT ( 'NONE',  ( 339.9999999999999432, 185.0000000000000284, -356.0000000000001705 ) ) ;
#14158=ORIENTED_EDGE ( 'NONE', *, *, #2018, .F. ) ;
#14160=VECTOR ( 'NONE', #38671, 1000.000000000000000 ) ;
#14162=CARTESIAN_POINT ( 'NONE',  ( 164.9999999999999716, -272.4999999999999432, -355.9999999999999432 ) ) ;
#14163=VECTOR ( 'NONE', #15580, 1000.000000000000000 ) ;
#14165=ORIENTED_EDGE ( 'NONE', *, *, #42796, .F. ) ;
#14167=ORIENTED_EDGE ( 'NONE', *, *, #23969, .T. ) ;
#14170=( BOUNDED_CURVE ( )  B_SPLINE_CURVE ( 3, ( #30089, #9810, #34198, #22369 ),
 .UNSPECIFIED., .F., .F. ) 
 B_SPLINE_CURVE_WITH_KNOTS ( ( 4, 4 ),
 ( 1.570796326794883013, 3.141592653589793560 ),
 .UNSPECIFIED. ) 
 CURVE ( )  GEOMETRIC_REPRESENTATION_ITEM ( )  RATIONAL_B_SPLINE_CURVE ( ( 1.000000000000000000, 0.8047378541243617178, 0.8047378541243617178, 1.000000000000000000 ) ) 
 REPRESENTATION_ITEM ( '' )  );
#14176=DIRECTION ( 'NONE',  ( 0.000000000000000000, -0.000000000000000000, 1.000000000000000000 ) ) ;
#14177=DIRECTION ( 'NONE',  ( -0.000000000000000000, -1.000000000000000000, -0.000000000000000000 ) ) ;
#14183=EDGE_CURVE ( 'NONE', #14529, #46434, #42823, .T. ) ;
#14190=VECTOR ( 'NONE', #23423, 1000.000000000000000 ) ;
#14191=FACE_OUTER_BOUND ( 'NONE', #24833, .T. ) ;
#14194=AXIS2_PLACEMENT_3D ( 'NONE', #32735, #16833, #5781 ) ;
#14195=VERTEX_POINT ( 'NONE', #38507 ) ;
#14196=EDGE_CURVE ( 'NONE', #4014, #17305, #28951, .T. ) ;
#14198=CIRCLE ( 'NONE', #46141, 2.000000000000001776 ) ;
#14202=VECTOR ( 'NONE', #28827, 1000.000000000000000 ) ;
#14207=DIRECTION ( 'NONE',  ( 6.203854594147707562E-25, -2.067951531382569187E-25, 1.000000000000000000 ) ) ;
#14211=CARTESIAN_POINT ( 'NONE',  ( 355.9999999999999432, 185.0000000000002274, -360.0000000000003411 ) ) ;
#14213=VERTEX_POINT ( 'NONE', #24611 ) ;
#14214=CARTESIAN_POINT ( 'NONE',  ( 168.9999999999999716, -97.49999999999997158, -115.0000000000001563 ) ) ;
#14224=ADVANCED_FACE ( 'NONE', ( #9450 ), #32572, .F. ) ;
#14225=CARTESIAN_POINT ( 'NONE',  ( 350.0000000000000000, 165.0000000000000000, -344.0000000000001705 ) ) ;
#14232=VECTOR ( 'NONE', #40999, 1000.000000000000000 ) ;
#14234=EDGE_CURVE ( 'NONE', #35315, #33292, #513, .T. ) ;
#14236=VECTOR ( 'NONE', #5337, 1000.000000000000000 ) ;
#14238=( NAMED_UNIT ( * ) PLANE_ANGLE_UNIT ( ) SI_UNIT ( $, .RADIAN. ) );
#14243=CARTESIAN_POINT ( 'NONE',  ( 340.0000000000000568, 165.0000000000000000, 349.9999999999998295 ) ) ;
#14245=EDGE_CURVE ( 'NONE', #19216, #37443, #47651, .T. ) ;
#14250=ADVANCED_FACE ( 'NONE', ( #20495 ), #28207, .F. ) ;
#14251=DIRECTION ( 'NONE',  ( -0.000000000000000000, -1.000000000000000000, 2.537652627714643577E-15 ) ) ;
#14252=AXIS2_PLACEMENT_3D ( 'NONE', #22746, #25845, #10440 ) ;
#14253=VERTEX_POINT ( 'NONE', #40014 ) ;
#14259=ORIENTED_EDGE ( 'NONE', *, *, #2988, .T. ) ;
#14268=AXIS2_PLACEMENT_3D ( 'NONE', #21964, #6819, #34278 ) ;
#14273=DIRECTION ( 'NONE',  ( 1.000000000000000000, 0.000000000000000000, 0.000000000000000000 ) ) ;
#14277=CARTESIAN_POINT ( 'NONE',  ( 355.9999999999999432, 174.9999999999996589, -356.0000000000003411 ) ) ;
#14278=EDGE_CURVE ( 'NONE', #20660, #21333, #16915, .T. ) ;
#14284=EDGE_CURVE ( 'NONE', #31660, #6290, #41756, .T. ) ;
#14288=CARTESIAN_POINT ( 'NONE',  ( 185.0000000000000000, -272.5000000000000000, -104.9999999999999289 ) ) ;
#14297=PLANE ( 'NONE',  #36152 ) ;
#14300=EDGE_CURVE ( 'NONE', #20217, #43954, #34083, .T. ) ;
#14307=DIRECTION ( 'NONE',  ( 0.000000000000000000, -1.000000000000000000, 3.469446951953611033E-15 ) ) ;
#14308=ORIENTED_EDGE ( 'NONE', *, *, #3320, .F. ) ;
#14312=VECTOR ( 'NONE', #24345, 1000.000000000000000 ) ;
#14317=DIRECTION ( 'NONE',  ( 0.000000000000000000, 0.000000000000000000, 1.000000000000000000 ) ) ;
#14318=FACE_OUTER_BOUND ( 'NONE', #50168, .T. ) ;
#14330=LINE ( 'NONE', #26134, #41511 ) ;
#14333=VECTOR ( 'NONE', #28263, 1000.000000000000000 ) ;
#14335=ORIENTED_EDGE ( 'NONE', *, *, #2018, .T. ) ;
#14345=EDGE_CURVE ( 'NONE', #6960, #6508, #10462, .T. ) ;
#14350=EDGE_CURVE ( 'NONE', #28031, #47828, #22932, .T. ) ;
#14353=AXIS2_PLACEMENT_3D ( 'NONE', #46748, #38610, #2911 ) ;
#14362=VERTEX_POINT ( 'NONE', #14553 ) ;
#14363=CARTESIAN_POINT ( 'NONE',  ( 350.0000000000000000, 169.0000000000000000, -342.0000000000001705 ) ) ;
#14367=CARTESIAN_POINT ( 'NONE',  ( 183.0000000000000000, -272.5000000000000000, -98.99999999999944578 ) ) ;
#14373=VERTEX_POINT ( 'NONE', #2750 ) ;
#14375=AXIS2_PLACEMENT_3D ( 'NONE', #9696, #26364, #2999 ) ;
#14377=CARTESIAN_POINT ( 'NONE',  ( 339.9999999999999432, -166.9999999999999432, -344.0000000000001705 ) ) ;
#14394=DIRECTION ( 'NONE',  ( 0.000000000000000000, 0.000000000000000000, 1.000000000000000000 ) ) ;
#14397=ORIENTED_EDGE ( 'NONE', *, *, #3439, .T. ) ;
#14399=FACE_OUTER_BOUND ( 'NONE', #22289, .T. ) ;
#14405=CARTESIAN_POINT ( 'NONE',  ( 0.000000000000000000, 175.0000000000000284, -353.7500000000001705 ) ) ;
#14406=CARTESIAN_POINT ( 'NONE',  ( 343.9999999999998863, -165.0000000000001137, -92.00000000000019895 ) ) ;
#14411=AXIS2_PLACEMENT_3D ( 'NONE', #32024, #44044, #8910 ) ;
#14413=VECTOR ( 'NONE', #38875, 1000.000000000000000 ) ;
#14414=DIRECTION ( 'NONE',  ( 1.860490536778032451E-50, 0.000000000000000000, -1.000000000000000000 ) ) ;
#14415=ORIENTED_EDGE ( 'NONE', *, *, #17340, .F. ) ;
#14416=VERTEX_POINT ( 'NONE', #10211 ) ;
#14419=ADVANCED_FACE ( 'NONE', ( #38436 ), #3251, .F. ) ;
#14427=STYLED_ITEM('',(#50747),#21652);
#14434=VECTOR ( 'NONE', #33280, 1000.000000000000000 ) ;
#14445=LINE ( 'NONE', #37817, #30338 ) ;
#14448=AXIS2_PLACEMENT_3D ( 'NONE', #47997, #47743, #27550 ) ;
#14449=LINE ( 'NONE', #30359, #804 ) ;
#14456=ORIENTED_EDGE ( 'NONE', *, *, #19340, .F. ) ;
#14457=VERTEX_POINT ( 'NONE', #18650 ) ;
#14460=DIRECTION ( 'NONE',  ( 0.000000000000000000, 0.000000000000000000, 1.000000000000000000 ) ) ;
#14462=ORIENTED_EDGE ( 'NONE', *, *, #37131, .T. ) ;
#14473=ORIENTED_EDGE ( 'NONE', *, *, #37076, .F. ) ;
#14483=AXIS2_PLACEMENT_3D ( 'NONE', #45103, #9224, #9474 ) ;
#14485=ORIENTED_EDGE ( 'NONE', *, *, #304, .F. ) ;
#14488=DIRECTION ( 'NONE',  ( -1.860490536778032451E-50, 0.000000000000000000, 1.000000000000000000 ) ) ;
#14495=DIRECTION ( 'NONE',  ( 1.000000000000000000, -4.758098676964956461E-16, -8.975803739141899931E-48 ) ) ;
#14498=ORIENTED_EDGE ( 'NONE', *, *, #33491, .T. ) ;
#14502=LINE ( 'NONE', #14243, #42038 ) ;
#14503=DIRECTION ( 'NONE',  ( -1.586032892321652236E-16, -1.000000000000000000, -2.288264760618012091E-48 ) ) ;
#14504=ORIENTED_EDGE ( 'NONE', *, *, #26298, .T. ) ;
#14505=EDGE_CURVE ( 'NONE', #14722, #13231, #21961, .T. ) ;
#14510=AXIS2_PLACEMENT_3D ( 'NONE', #36518, #27346, #46545 ) ;
#14513=CARTESIAN_POINT ( 'NONE',  ( 169.0000000000000000, -174.9999999999999716, -97.00000000000014211 ) ) ;
#14517=VERTEX_POINT ( 'NONE', #26619 ) ;
#14518=CARTESIAN_POINT ( 'NONE',  ( 181.0000000000000000, -164.9999999999999432, 341.9999999999998863 ) ) ;
#14523=CARTESIAN_POINT ( 'NONE',  ( 350.0000000000000000, -180.9999999999999716, -344.0000000000001705 ) ) ;
#14524=ORIENTED_EDGE ( 'NONE', *, *, #12940, .T. ) ;
#14527=FACE_OUTER_BOUND ( 'NONE', #41843, .T. ) ;
#14529=VERTEX_POINT ( 'NONE', #22764 ) ;
#14532=ADVANCED_FACE ( 'NONE', ( #34578 ), #42507, .F. ) ;
#14535=EDGE_CURVE ( 'NONE', #8324, #19838, #35229, .T. ) ;
#14537=ORIENTED_EDGE ( 'NONE', *, *, #23878, .F. ) ;
#14538=CARTESIAN_POINT ( 'NONE',  ( 181.0000000000000568, 175.0000000000000284, 357.9999999999998863 ) ) ;
#14543=EDGE_CURVE ( 'NONE', #42571, #6887, #46580, .T. ) ;
#14545=VECTOR ( 'NONE', #35272, 1000.000000000000114 ) ;
#14553=CARTESIAN_POINT ( 'NONE',  ( -5.000000000000000000, 184.8000000000000114, -340.2000000000001592 ) ) ;
#14564=ADVANCED_FACE ( 'NONE', ( #195 ), #43274, .T. ) ;
#14567=DIRECTION ( 'NONE',  ( -1.000000000000000000, 0.000000000000000000, -7.793956916774525800E-48 ) ) ;
#14573=DIRECTION ( 'NONE',  ( 1.000000000000000000, 0.000000000000000000, -0.000000000000000000 ) ) ;
#14577=LINE ( 'NONE', #9719, #2202 ) ;
#14582=ORIENTED_EDGE ( 'NONE', *, *, #34251, .T. ) ;
#14588=VERTEX_POINT ( 'NONE', #28895 ) ;
#14589=DIRECTION ( 'NONE',  ( 1.942330104924128867E-32, 0.000000000000000000, 1.000000000000000000 ) ) ;
#14596=EDGE_CURVE ( 'NONE', #4014, #47178, #24592, .T. ) ;
#14600=ORIENTED_EDGE ( 'NONE', *, *, #49816, .F. ) ;
#14605=DIRECTION ( 'NONE',  ( 0.000000000000000000, -1.000000000000000000, 0.000000000000000000 ) ) ;
#14610=VERTEX_POINT ( 'NONE', #27896 ) ;
#14613=PLANE ( 'NONE',  #46601 ) ;
#14620=VECTOR ( 'NONE', #8077, 1000.000000000000000 ) ;
#14630=CLOSED_SHELL ( 'NONE', ( #38241, #27473, #38886, #29545, #29901, #9337, #47517, #2706, #31985, #35118, #39107, #49681, #25914, #43581, #18053, #30845, #26924, #31222 ) ) ;
#14633=DIRECTION ( 'NONE',  ( -3.172065784643302499E-16, -1.000000000000000000, 2.537652627714642000E-15 ) ) ;
#14636=CARTESIAN_POINT ( 'NONE',  ( 181.0000000000000568, 175.0000000000000284, 359.9999999999998863 ) ) ;
#14648=CARTESIAN_POINT ( 'NONE',  ( 181.0000000000000000, -184.9999999999999716, -358.0000000000001705 ) ) ;
#14655=VECTOR ( 'NONE', #19346, 1000.000000000000000 ) ;
#14658=DIRECTION ( 'NONE',  ( 4.758098676964954489E-16, 1.000000000000000000, 1.751623080406021339E-46 ) ) ;
#14662=VECTOR ( 'NONE', #32611, 1000.000000000000000 ) ;
#14663=AXIS2_PLACEMENT_3D ( 'NONE', #23562, #50710, #46861 ) ;
#14670=CARTESIAN_POINT ( 'NONE',  ( 350.0000000000000000, -168.9999999999999432, -342.0000000000001705 ) ) ;
#14678=LINE ( 'NONE', #3122, #49035 ) ;
#14683=DIRECTION ( 'NONE',  ( 1.333906992743555050E-23, -1.000000000000000000, 0.000000000000000000 ) ) ;
#14691=AXIS2_PLACEMENT_3D ( 'NONE', #20116, #21125, #20365 ) ;
#14697=STYLED_ITEM('',(#50747),#4445);
#14702=EDGE_LOOP ( 'NONE', ( #6933, #30460, #12375, #35757 ) ) ;
#14710=FACE_OUTER_BOUND ( 'NONE', #30676, .T. ) ;
#14718=DIRECTION ( 'NONE',  ( 1.612977847700450206E-50, 0.000000000000000000, 1.000000000000000000 ) ) ;
#14721=ORIENTED_EDGE ( 'NONE', *, *, #23750, .F. ) ;
#14722=VERTEX_POINT ( 'NONE', #45016 ) ;
#14723=CARTESIAN_POINT ( 'NONE',  ( 339.9999999999998863, -185.0000000000001421, 343.9999999999997726 ) ) ;
#14727=AXIS2_PLACEMENT_3D ( 'NONE', #45337, #42025, #14317 ) ;
#14736=LINE ( 'NONE', #18074, #45754 ) ;
#14752=ORIENTED_EDGE ( 'NONE', *, *, #27869, .F. ) ;
#14780=VERTEX_POINT ( 'NONE', #30412 ) ;
#14800=PLANE ( 'NONE',  #47333 ) ;
#14810=DIRECTION ( 'NONE',  ( -1.000000000000000000, -0.000000000000000000, -0.000000000000000000 ) ) ;
#14813=CARTESIAN_POINT ( 'NONE',  ( 350.0000000000001137, 169.0000000000000000, 355.9999999999997726 ) ) ;
#14815=CARTESIAN_POINT ( 'NONE',  ( 356.0000000000000000, -165.0000000000001137, -349.9999999999998863 ) ) ;
#14822=VERTEX_POINT ( 'NONE', #35049 ) ;
#14824=FACE_OUTER_BOUND ( 'NONE', #35374, .T. ) ;
#14831=LINE ( 'NONE', #27401, #44770 ) ;
#14832=ORIENTED_EDGE ( 'NONE', *, *, #32308, .T. ) ;
#14835=AXIS2_PLACEMENT_3D ( 'NONE', #20849, #43677, #44677 ) ;
#14841=CARTESIAN_POINT ( 'NONE',  ( 358.0000000000000568, -167.8284271247463550, -342.8284271247465540 ) ) ;
#14842=FACE_OUTER_BOUND ( 'NONE', #2163, .T. ) ;
#14845=ORIENTED_EDGE ( 'NONE', *, *, #25993, .T. ) ;
#14846=CARTESIAN_POINT ( 'NONE',  ( 166.9999999999999716, -174.9999999999999716, -356.0000000000001705 ) ) ;
#14849=CARTESIAN_POINT ( 'NONE',  ( 343.9999999999999432, -183.0000000000001421, 358.0000000000001137 ) ) ;
#14853=CARTESIAN_POINT ( 'NONE',  ( 183.0000000000000284, -174.9999999999999716, -111.0000000000001563 ) ) ;
#14856=CARTESIAN_POINT ( 'NONE',  ( 342.0000000000000000, 169.0000000000000000, 343.9999999999998863 ) ) ;
#14857=CARTESIAN_POINT ( 'NONE',  ( 357.9999999999999432, 177.9999999999999432, -353.0000000000000568 ) ) ;
#14860=LINE ( 'NONE', #18446, #10872 ) ;
#14861=ADVANCED_FACE ( 'NONE', ( #22704, #7573 ), #38124, .T. ) ;
#14866=DIRECTION ( 'NONE',  ( 0.000000000000000000, -4.687818848539279227E-49, 1.000000000000000000 ) ) ;
#14867=ADVANCED_FACE ( 'NONE', ( #47290 ), #9090, .F. ) ;
#14871=VERTEX_POINT ( 'NONE', #48035 ) ;
#14872=EDGE_CURVE ( 'NONE', #19026, #18177, #28582, .T. ) ;
#14875=AXIS2_PLACEMENT_3D ( 'NONE', #14363, #21056, #21819 ) ;
#14902=EDGE_CURVE ( 'NONE', #21347, #14373, #18019, .T. ) ;
#14903=CARTESIAN_POINT ( 'NONE',  ( 5.551115123125782702E-14, -168.9999999999999432, 343.9999999999997726 ) ) ;
#14908=CARTESIAN_POINT ( 'NONE',  ( 340.0000000000000568, 165.0000000000000000, 343.9999999999997726 ) ) ;
#14912=ADVANCED_FACE ( 'NONE', ( #24492 ), #16537, .T. ) ;
#14916=CARTESIAN_POINT ( 'NONE',  ( 358.0000000000000000, -169.0000000000001137, -344.0000000000002842 ) ) ;
#14921=CYLINDRICAL_SURFACE ( 'NONE', #37384, 2.000000000000001776 ) ;
#14927=DIRECTION ( 'NONE',  ( -0.000000000000000000, -1.000000000000000000, 2.537652627714643577E-15 ) ) ;
#14929=ADVANCED_FACE ( 'NONE', ( #47786 ), #31948, .F. ) ;
#14946=CARTESIAN_POINT ( 'NONE',  ( 0.000000000000000000, 181.0000000000000284, -358.0000000000002274 ) ) ;
#14948=CARTESIAN_POINT ( 'NONE',  ( 341.6568542494921417, -185.0000000000001137, 360.0000000000002274 ) ) ;
#14949=CARTESIAN_POINT ( 'NONE',  ( -5.000000000000000000, 175.0000000000000284, -350.0000000000002274 ) ) ;
#14950=VERTEX_POINT ( 'NONE', #21380 ) ;
#14955=AXIS2_PLACEMENT_3D ( 'NONE', #14903, #25501, #18729 ) ;
#14964=LINE ( 'NONE', #45971, #32069 ) ;
#14968=CARTESIAN_POINT ( 'NONE',  ( 340.0000000000000000, -2.999999999999919176, 171.9999999999998295 ) ) ;
#14973=CYLINDRICAL_SURFACE ( 'NONE', #3372, 4.000000000000003553 ) ;
#14976=ORIENTED_EDGE ( 'NONE', *, *, #23465, .T. ) ;
#14980=CARTESIAN_POINT ( 'NONE',  ( 0.000000000000000000, 169.0000000000000000, -342.0000000000001705 ) ) ;
#14982=DIRECTION ( 'NONE',  ( 0.000000000000000000, 0.000000000000000000, -1.000000000000000000 ) ) ;
#14986=STYLED_ITEM('',(#50747),#39060);
#14988=EDGE_LOOP ( 'NONE', ( #6893, #42984, #39579, #35556 ) ) ;
#14992=CARTESIAN_POINT ( 'NONE',  ( 168.9999999999999716, -164.9999999999999432, -356.0000000000001705 ) ) ;
#14993=EDGE_CURVE ( 'NONE', #18727, #13237, #24998, .T. ) ;
#14996=LINE ( 'NONE', #45746, #13487 ) ;
#14997=ORIENTED_EDGE ( 'NONE', *, *, #29891, .F. ) ;
#15002=LINE ( 'NONE', #30660, #14620 ) ;
#15007=CARTESIAN_POINT ( 'NONE',  ( 350.0000000000001137, 165.0000000000000000, 355.9999999999997726 ) ) ;
#15011=VERTEX_POINT ( 'NONE', #7515 ) ;
#15014=CARTESIAN_POINT ( 'NONE',  ( 5.551115123125782702E-14, -184.9999999999999716, 343.9999999999997726 ) ) ;
#15016=AXIS2_PLACEMENT_3D ( 'NONE', #21940, #42184, #37607 ) ;
#15017=VERTEX_POINT ( 'NONE', #7777 ) ;
#15028=ORIENTED_EDGE ( 'NONE', *, *, #11274, .F. ) ;
#15033=DIRECTION ( 'NONE',  ( -1.000000000000000000, 0.000000000000000000, 0.000000000000000000 ) ) ;
#15034=ORIENTED_EDGE ( 'NONE', *, *, #45364, .F. ) ;
#15036=DIRECTION ( 'NONE',  ( 1.000000000000000000, 0.000000000000000000, 0.000000000000000000 ) ) ;
#15048=CARTESIAN_POINT ( 'NONE',  ( 166.9999999999999716, 6.000000000000060396, -340.0000000000001137 ) ) ;
#15060=DIRECTION ( 'NONE',  ( 0.000000000000000000, 0.000000000000000000, 1.000000000000000000 ) ) ;
#15064=DIRECTION ( 'NONE',  ( 1.000000000000000000, 0.000000000000000000, 1.612977847700450206E-50 ) ) ;
#15066=DIRECTION ( 'NONE',  ( 0.000000000000000000, 6.123233995736766036E-17, -1.000000000000000000 ) ) ;
#15067=( BOUNDED_CURVE ( )  B_SPLINE_CURVE ( 3, ( #38664, #49644, #6590, #3482 ),
 .UNSPECIFIED., .F., .F. ) 
 B_SPLINE_CURVE_WITH_KNOTS ( ( 4, 4 ),
 ( 1.570796326794890119, 3.141592653589794004 ),
 .UNSPECIFIED. ) 
 CURVE ( )  GEOMETRIC_REPRESENTATION_ITEM ( )  RATIONAL_B_SPLINE_CURVE ( ( 1.000000000000000000, 0.8047378541243632721, 0.8047378541243632721, 1.000000000000000000 ) ) 
 REPRESENTATION_ITEM ( '' )  );
#15071=CARTESIAN_POINT ( 'NONE',  ( 340.0000000000000568, 181.0000000000000853, 355.9999999999998295 ) ) ;
#15072=VERTEX_POINT ( 'NONE', #30356 ) ;
#15076=CARTESIAN_POINT ( 'NONE',  ( -5.000000000000000000, 165.2000000000000171, 359.7999999999997840 ) ) ;
#15079=LINE ( 'NONE', #27140, #20800 ) ;
#15080=ORIENTED_EDGE ( 'NONE', *, *, #23419, .T. ) ;
#15083=ORIENTED_EDGE ( 'NONE', *, *, #20969, .F. ) ;
#15086=VECTOR ( 'NONE', #47354, 1000.000000000000000 ) ;
#15090=CARTESIAN_POINT ( 'NONE',  ( 339.9999999999998863, -164.9999999999999432, 343.9999999999997726 ) ) ;
#15101=ORIENTED_EDGE ( 'NONE', *, *, #1454, .F. ) ;
#15103=CARTESIAN_POINT ( 'NONE',  ( 340.0000000000000568, 181.0000000000000284, 339.9999999999997726 ) ) ;
#15107=( NAMED_UNIT ( * ) SI_UNIT ( $, .STERADIAN. ) SOLID_ANGLE_UNIT ( ) );
#15117=ORIENTED_EDGE ( 'NONE', *, *, #3554, .T. ) ;
#15120=LINE ( 'NONE', #18701, #32249 ) ;
#15121=ORIENTED_EDGE ( 'NONE', *, *, #22998, .F. ) ;
#15123=EDGE_CURVE ( 'NONE', #10108, #43146, #42627, .T. ) ;
#15124=LINE ( 'NONE', #3829, #22903 ) ;
#15128=ORIENTED_EDGE ( 'NONE', *, *, #17355, .T. ) ;
#15133=CARTESIAN_POINT ( 'NONE',  ( 341.6568542494922553, -185.0000000000001705, -360.0000000000003411 ) ) ;
#15141=EDGE_CURVE ( 'NONE', #21498, #30616, #14445, .T. ) ;
#15142=VECTOR ( 'NONE', #39884, 1000.000000000000000 ) ;
#15158=EDGE_CURVE ( 'NONE', #14871, #19563, #4947, .T. ) ;
#15161=VECTOR ( 'NONE', #1643, 1000.000000000000000 ) ;
#15166=VERTEX_POINT ( 'NONE', #8278 ) ;
#15169=DIRECTION ( 'NONE',  ( -0.000000000000000000, -1.000000000000000000, -0.000000000000000000 ) ) ;
#15171=CARTESIAN_POINT ( 'NONE',  ( 5.551115123125782702E-14, -164.9999999999999432, 343.9999999999997726 ) ) ;
#15174=CARTESIAN_POINT ( 'NONE',  ( 5.551115123125782702E-14, -180.9999999999999716, 355.9999999999997726 ) ) ;
#15175=DIRECTION ( 'NONE',  ( 1.132880637372608740E-16, 4.718402560806925739E-50, 1.000000000000000000 ) ) ;
#15179=ORIENTED_EDGE ( 'NONE', *, *, #767, .F. ) ;
#15182=CARTESIAN_POINT ( 'NONE',  ( 340.0000000000000000, -166.6568542494923406, 341.6568542494921985 ) ) ;
#15185=ADVANCED_FACE ( 'NONE', ( #33084 ), #47230, .F. ) ;
#15186=CARTESIAN_POINT ( 'NONE',  ( 183.0000000000000000, -5.999999999999950262, -350.0000000000001705 ) ) ;
#15191=CARTESIAN_POINT ( 'NONE',  ( 168.9999999999999716, -81.49999999999997158, -350.0000000000001705 ) ) ;
#15202=AXIS2_PLACEMENT_3D ( 'NONE', #1544, #44111, #24644 ) ;
#15204=ORIENTED_EDGE ( 'NONE', *, *, #44013, .F. ) ;
#15207=DIRECTION ( 'NONE',  ( 0.000000000000000000, 0.000000000000000000, 1.000000000000000000 ) ) ;
#15208=CIRCLE ( 'NONE', #27481, 2.000000000000001776 ) ;
#15209=VERTEX_POINT ( 'NONE', #31381 ) ;
#15217=CYLINDRICAL_SURFACE ( 'NONE', #26684, 3.749999999999975575 ) ;
#15222=EDGE_CURVE ( 'NONE', #21391, #30988, #19806, .T. ) ;
#15224=EDGE_CURVE ( 'NONE', #20342, #41044, #8259, .T. ) ;
#15229=FACE_OUTER_BOUND ( 'NONE', #25610, .T. ) ;
#15236=VECTOR ( 'NONE', #18451, 1000.000000000000000 ) ;
#15237=CARTESIAN_POINT ( 'NONE',  ( 0.000000000000000000, 183.0000000000000284, 355.9999999999997726 ) ) ;
#15239=( BOUNDED_CURVE ( )  B_SPLINE_CURVE ( 3, ( #7017, #31133, #30624, #22659 ),
 .UNSPECIFIED., .F., .F. ) 
 B_SPLINE_CURVE_WITH_KNOTS ( ( 4, 4 ),
 ( 4.712388980384676351, 6.283185307179586232 ),
 .UNSPECIFIED. ) 
 CURVE ( )  GEOMETRIC_REPRESENTATION_ITEM ( )  RATIONAL_B_SPLINE_CURVE ( ( 1.000000000000000000, 0.8047378541243618288, 0.8047378541243618288, 1.000000000000000000 ) ) 
 REPRESENTATION_ITEM ( '' )  );
#15240=CARTESIAN_POINT ( 'NONE',  ( 339.9999999999999432, -180.9999999999999716, -340.0000000000001705 ) ) ;
#15250=EDGE_LOOP ( 'NONE', ( #27785, #49305, #6558, #29210 ) ) ;
#15255=CARTESIAN_POINT ( 'NONE',  ( 360.0000000000000000, 183.3431457505076310, -358.3431457505078015 ) ) ;
#15259=DIRECTION ( 'NONE',  ( 0.000000000000000000, -2.969158215481698263E-48, 1.000000000000000000 ) ) ;
#15267=VECTOR ( 'NONE', #19114, 1000.000000000000000 ) ;
#15270=DIRECTION ( 'NONE',  ( 0.000000000000000000, -2.969158215481698263E-48, 1.000000000000000000 ) ) ;
#15272=EDGE_CURVE ( 'NONE', #8483, #41468, #25260, .T. ) ;
#15285=VECTOR ( 'NONE', #23430, 1000.000000000000000 ) ;
#15288=EDGE_CURVE ( 'NONE', #21333, #42541, #2496, .T. ) ;
#15289=EDGE_LOOP ( 'NONE', ( #29180, #22535, #12868, #18541 ) ) ;
#15292=DIRECTION ( 'NONE',  ( 1.586032892321652482E-16, 0.000000000000000000, 1.000000000000000000 ) ) ;
#15295=ORIENTED_EDGE ( 'NONE', *, *, #19588, .T. ) ;
#15298=ADVANCED_FACE ( 'NONE', ( #5865 ), #25878, .F. ) ;
#15299=LINE ( 'NONE', #11193, #7018 ) ;
#15303=FACE_BOUND ( 'NONE', #38855, .T. ) ;
#15304=AXIS2_PLACEMENT_3D ( 'NONE', #21973, #29671, #22228 ) ;
#15306=CARTESIAN_POINT ( 'NONE',  ( 0.000000000000000000, -164.9999999999999432, -356.0000000000002274 ) ) ;
#15308=STYLED_ITEM('',(#50747),#21149);
#15310=DIRECTION ( 'NONE',  ( -1.586032892321652236E-16, -1.000000000000000000, -2.288264760618012091E-48 ) ) ;
#15312=EDGE_CURVE ( 'NONE', #8581, #5103, #37716, .T. ) ;
#15320=CARTESIAN_POINT ( 'NONE',  ( 183.0000000000000284, -9.999999999999953815, -111.0000000000001563 ) ) ;
#15331=LINE ( 'NONE', #30986, #9464 ) ;
#15337=EDGE_LOOP ( 'NONE', ( #8830, #6810, #28998, #7152 ) ) ;
#15342=EDGE_LOOP ( 'NONE', ( #7217, #33937, #31956, #32975 ) ) ;
#15343=DIRECTION ( 'NONE',  ( -1.000000000000000000, -0.000000000000000000, -0.000000000000000000 ) ) ;
#15345=VERTEX_POINT ( 'NONE', #37947 ) ;
#15347=ADVANCED_FACE ( 'NONE', ( #14057 ), #10224, .T. ) ;
#15353=ORIENTED_EDGE ( 'NONE', *, *, #6051, .T. ) ;
#15357=ADVANCED_FACE ( 'NONE', ( #21769, #14824 ), #13799, .F. ) ;
#15361=CARTESIAN_POINT ( 'NONE',  ( 166.9999999999999716, -256.4999999999999432, -339.9999999999998863 ) ) ;
#15367=DIRECTION ( 'NONE',  ( -1.000000000000000000, 0.000000000000000000, 0.000000000000000000 ) ) ;
#15379=ORIENTED_EDGE ( 'NONE', *, *, #40435, .F. ) ;
#15381=( BOUNDED_CURVE ( )  B_SPLINE_CURVE ( 3, ( #33591, #14069, #41528, #22022 ),
 .UNSPECIFIED., .F., .F. ) 
 B_SPLINE_CURVE_WITH_KNOTS ( ( 4, 4 ),
 ( 3.141592653589793560, 4.712388980384745629 ),
 .UNSPECIFIED. ) 
 CURVE ( )  GEOMETRIC_REPRESENTATION_ITEM ( )  RATIONAL_B_SPLINE_CURVE ( ( 1.000000000000000000, 0.8047378541243519479, 0.8047378541243519479, 1.000000000000000000 ) ) 
 REPRESENTATION_ITEM ( '' )  );
#15383=DIRECTION ( 'NONE',  ( 0.000000000000000000, -1.000000000000000000, -3.186989995019654210E-49 ) ) ;
#15384=LINE ( 'NONE', #27688, #10082 ) ;
#15385=ORIENTED_EDGE ( 'NONE', *, *, #7571, .T. ) ;
#15402=VECTOR ( 'NONE', #41497, 1000.000000000000000 ) ;
#15406=EDGE_LOOP ( 'NONE', ( #6135, #41283, #3959, #37596 ) ) ;
#15407=CARTESIAN_POINT ( 'NONE',  ( 168.9999999999999716, -174.9999999999999716, -340.0000000000001137 ) ) ;
#15408=LINE ( 'NONE', #31064, #40646 ) ;
#15410=ORIENTED_EDGE ( 'NONE', *, *, #1218, .T. ) ;
#15413=EDGE_LOOP ( 'NONE', ( #25067, #42925, #13394, #2651 ) ) ;
#15414=DIRECTION ( 'NONE',  ( 0.000000000000000000, 0.000000000000000000, 1.000000000000000000 ) ) ;
#15416=ORIENTED_EDGE ( 'NONE', *, *, #8060, .T. ) ;
#15417=DIRECTION ( 'NONE',  ( 1.000000000000000000, 0.000000000000000000, 0.000000000000000000 ) ) ;
#15419=CARTESIAN_POINT ( 'NONE',  ( 0.000000000000000000, 181.0000000000000284, -342.0000000000001705 ) ) ;
#15426=VERTEX_POINT ( 'NONE', #37689 ) ;
#15428=LINE ( 'NONE', #26973, #4583 ) ;
#15430=ORIENTED_EDGE ( 'NONE', *, *, #11496, .T. ) ;
#15447=ORIENTED_EDGE ( 'NONE', *, *, #34201, .T. ) ;
#15455=CARTESIAN_POINT ( 'NONE',  ( 341.9999999999999432, -180.9999999999999716, 355.9999999999998295 ) ) ;
#15457=DIRECTION ( 'NONE',  ( 1.000000000000000000, -4.105366553918459587E-48, -1.586032880504786307E-16 ) ) ;
#15464=VECTOR ( 'NONE', #42321, 1000.000000000000000 ) ;
#15473=ADVANCED_FACE ( 'NONE', ( #22521 ), #33840, .F. ) ;
#15476=CLOSED_SHELL ( 'NONE', ( #28589, #25174, #20477, #19016, #22186, #7367, #36643, #4697, #20824, #23737, #23148, #43681, #50178, #13592, #4561, #8844, #38261, #16211 ) ) ;
#15477=ADVANCED_FACE ( 'NONE', ( #11999 ), #7645, .T. ) ;
#15480=AXIS2_PLACEMENT_3D ( 'NONE', #2524, #5612, #13308 ) ;
#15481=LINE ( 'NONE', #41918, #13222 ) ;
#15482=ORIENTED_EDGE ( 'NONE', *, *, #2655, .T. ) ;
#15493=CARTESIAN_POINT ( 'NONE',  ( 165.0000000000000284, 165.0000000000000000, 355.9999999999998863 ) ) ;
#15497=ORIENTED_EDGE ( 'NONE', *, *, #43098, .T. ) ;
#15498=ORIENTED_EDGE ( 'NONE', *, *, #26868, .T. ) ;
#15508=DIRECTION ( 'NONE',  ( -3.172065784643302499E-16, -1.000000000000000000, 2.537652627714642000E-15 ) ) ;
#15509=VECTOR ( 'NONE', #8486, 1000.000000000000000 ) ;
#15511=ORIENTED_EDGE ( 'NONE', *, *, #27869, .T. ) ;
#15520=FACE_OUTER_BOUND ( 'NONE', #3996, .T. ) ;
#15526=ADVANCED_FACE ( 'NONE', ( #15845 ), #42516, .T. ) ;
#15528=( BOUNDED_CURVE ( )  B_SPLINE_CURVE ( 3, ( #27304, #47522, #15255, #31415 ),
 .UNSPECIFIED., .F., .F. ) 
 B_SPLINE_CURVE_WITH_KNOTS ( ( 4, 4 ),
 ( 4.710277376051313914E-16, 1.570796326794896780 ),
 .UNSPECIFIED. ) 
 CURVE ( )  GEOMETRIC_REPRESENTATION_ITEM ( )  RATIONAL_B_SPLINE_CURVE ( ( 1.000000000000000000, 0.8047378541243650485, 0.8047378541243650485, 1.000000000000000000 ) ) 
 REPRESENTATION_ITEM ( '' )  );
#15530=ORIENTED_EDGE ( 'NONE', *, *, #6120, .T. ) ;
#15537=ORIENTED_EDGE ( 'NONE', *, *, #26805, .F. ) ;
#15539=CIRCLE ( 'NONE', #828, 2.000000000000001776 ) ;
#15549=ORIENTED_EDGE ( 'NONE', *, *, #8900, .F. ) ;
#15566=DIRECTION ( 'NONE',  ( 0.000000000000000000, 0.000000000000000000, -1.000000000000000000 ) ) ;
#15567=LINE ( 'NONE', #4277, #32624 ) ;
#15569=EDGE_CURVE ( 'NONE', #46042, #31660, #25561, .T. ) ;
#15571=ORIENTED_EDGE ( 'NONE', *, *, #42860, .F. ) ;
#15577=EDGE_CURVE ( 'NONE', #49298, #27092, #47858, .T. ) ;
#15580=DIRECTION ( 'NONE',  ( 2.220446049250312588E-16, 0.7071067811865475727, -0.7071067811865474617 ) ) ;
#15585=DIRECTION ( 'NONE',  ( -4.758098676964956461E-16, 0.000000000000000000, -1.000000000000000000 ) ) ;
#15590=VERTEX_POINT ( 'NONE', #20436 ) ;
#15592=DIRECTION ( 'NONE',  ( -0.000000000000000000, -0.000000000000000000, 1.000000000000000000 ) ) ;
#15597=LINE ( 'NONE', #27655, #41789 ) ;
#15600=ORIENTED_EDGE ( 'NONE', *, *, #12661, .T. ) ;
#15603=( NAMED_UNIT ( * ) SI_UNIT ( $, .STERADIAN. ) SOLID_ANGLE_UNIT ( ) );
#15607=ORIENTED_EDGE ( 'NONE', *, *, #23316, .F. ) ;
#15608=VERTEX_POINT ( 'NONE', #43788 ) ;
#15609=ORIENTED_EDGE ( 'NONE', *, *, #27826, .F. ) ;
#15618=PLANE ( 'NONE',  #26569 ) ;
#15620=CARTESIAN_POINT ( 'NONE',  ( 181.0000000000000284, -174.9999999999999716, -115.0000000000001563 ) ) ;
#15621=VECTOR ( 'NONE', #19256, 1000.000000000000000 ) ;
#15629=CARTESIAN_POINT ( 'NONE',  ( 168.9999999999999716, 6.000000000000060396, -350.0000000000001705 ) ) ;
#15630=ORIENTED_EDGE ( 'NONE', *, *, #16810, .F. ) ;
#15631=DIRECTION ( 'NONE',  ( 1.000000000000000000, 0.000000000000000000, 0.000000000000000000 ) ) ;
#15643=LINE ( 'NONE', #39261, #13948 ) ;
#15649=VECTOR ( 'NONE', #23736, 1000.000000000000000 ) ;
#15650=CIRCLE ( 'NONE', #40131, 4.000000000000003553 ) ;
#15651=ORIENTED_EDGE ( 'NONE', *, *, #21458, .T. ) ;
#15664=ORIENTED_EDGE ( 'NONE', *, *, #26431, .F. ) ;
#15667=VERTEX_POINT ( 'NONE', #6813 ) ;
#15669=DIRECTION ( 'NONE',  ( 0.000000000000000000, -3.186989995019654210E-49, -1.000000000000000000 ) ) ;
#15670=CARTESIAN_POINT ( 'NONE',  ( 181.0000000000000284, 2.775557561562891351E-14, -99.00000000000014211 ) ) ;
#15673=PLANE ( 'NONE',  #35411 ) ;
#15679=EDGE_LOOP ( 'NONE', ( #850, #27293, #36659, #23019, #4968, #12330, #15430, #12892 ) ) ;
#15688=VERTEX_POINT ( 'NONE', #2214 ) ;
#15694=DIRECTION ( 'NONE',  ( 0.000000000000000000, -1.000000000000000000, 2.537652627714643577E-15 ) ) ;
#15695=ORIENTED_EDGE ( 'NONE', *, *, #25940, .T. ) ;
#15703=PLANE ( 'NONE',  #18369 ) ;
#15710=ORIENTED_EDGE ( 'NONE', *, *, #37506, .F. ) ;
#15716=ORIENTED_EDGE ( 'NONE', *, *, #5062, .T. ) ;
#15718=ORIENTED_EDGE ( 'NONE', *, *, #13798, .F. ) ;
#15721=AXIS2_PLACEMENT_3D ( 'NONE', #20359, #36294, #43456 ) ;
#15733=ORIENTED_EDGE ( 'NONE', *, *, #22240, .T. ) ;
#15734=ORIENTED_EDGE ( 'NONE', *, *, #34471, .F. ) ;
#15735=CARTESIAN_POINT ( 'NONE',  ( 341.9999999999999432, -169.0000000000001137, -344.0000000000002842 ) ) ;
#15737=PLANE ( 'NONE',  #25096 ) ;
#15740=DIRECTION ( 'NONE',  ( -1.586032892321652236E-16, -1.000000000000000000, -2.288264760618012091E-48 ) ) ;
#15744=SHAPE_REPRESENTATION_RELATIONSHIP ( 'NONE' , 'NONE' ,  #13952, #38746 ) ;
#15745=LINE ( 'NONE', #619, #49752 ) ;
#15756=MECHANICAL_DESIGN_GEOMETRIC_PRESENTATION_REPRESENTATION('',(#11662),#46070);
#15759=PLANE ( 'NONE',  #49864 ) ;
#15761=EDGE_CURVE ( 'NONE', #2864, #46936, #21445, .T. ) ;
#15763=DIRECTION ( 'NONE',  ( -1.586032892321652236E-16, -1.000000000000000000, -2.288264760618012091E-48 ) ) ;
#15765=DIRECTION ( 'NONE',  ( -1.000000000000000000, 0.000000000000000000, -0.000000000000000000 ) ) ;
#15770=EDGE_CURVE ( 'NONE', #24618, #4113, #18056, .T. ) ;
#15772=ORIENTED_EDGE ( 'NONE', *, *, #6467, .T. ) ;
#15779=LINE ( 'NONE', #23220, #23278 ) ;
#15785=VECTOR ( 'NONE', #14207, 1000.000000000000000 ) ;
#15788=EDGE_CURVE ( 'NONE', #27142, #47198, #6055, .T. ) ;
#15793=VERTEX_POINT ( 'NONE', #49612 ) ;
#15797=CARTESIAN_POINT ( 'NONE',  ( 358.0000000000001137, 169.0000000000000000, 343.9999999999998295 ) ) ;
#15803=ADVANCED_FACE ( 'NONE', ( #6318 ), #1960, .T. ) ;
#15805=UNCERTAINTY_MEASURE_WITH_UNIT (LENGTH_MEASURE( 1.000000000000000082E-05 ), #47360, 'distance_accuracy_value', 'NONE');
#15809=VERTEX_POINT ( 'NONE', #45533 ) ;
#15814=VERTEX_POINT ( 'NONE', #10413 ) ;
#15815=CARTESIAN_POINT ( 'NONE',  ( 181.0000000000000000, 175.0000000000000284, -344.0000000000001137 ) ) ;
#15820=EDGE_CURVE ( 'NONE', #33697, #43357, #36141, .T. ) ;
#15821=EDGE_CURVE ( 'NONE', #5037, #45423, #42664, .T. ) ;
#15825=EDGE_CURVE ( 'NONE', #26083, #16304, #8093, .T. ) ;
#15830=VERTEX_POINT ( 'NONE', #7845 ) ;
#15833=DIRECTION ( 'NONE',  ( 0.000000000000000000, -2.537652627714643577E-15, -1.000000000000000000 ) ) ;
#15840=DIRECTION ( 'NONE',  ( -2.958228394578794708E-31, 0.000000000000000000, 1.000000000000000000 ) ) ;
#15845=FACE_OUTER_BOUND ( 'NONE', #41627, .T. ) ;
#15852=LINE ( 'NONE', #11254, #42255 ) ;
#15856=EDGE_CURVE ( 'NONE', #750, #32832, #2529, .T. ) ;
#15857=CARTESIAN_POINT ( 'NONE',  ( 343.9999999999999432, -185.0000000000001421, -360.0000000000003411 ) ) ;
#15858=CARTESIAN_POINT ( 'NONE',  ( 183.0000000000000000, -268.4999999999999432, -339.9999999999998863 ) ) ;
#15859=CIRCLE ( 'NONE', #26514, 2.000000000000001776 ) ;
#15860=ORIENTED_EDGE ( 'NONE', *, *, #35999, .F. ) ;
#15862=VERTEX_POINT ( 'NONE', #50628 ) ;
#15863=LINE ( 'NONE', #46613, #43457 ) ;
#15874=CARTESIAN_POINT ( 'NONE',  ( 339.9999999999998863, -174.9999999999999432, 355.9999999999998295 ) ) ;
#15883=LINE ( 'NONE', #11277, #43091 ) ;
#15884=VECTOR ( 'NONE', #12151, 1000.000000000000000 ) ;
#15887=CARTESIAN_POINT ( 'NONE',  ( 339.9999999999998863, -185.0000000000001421, -344.0000000000001705 ) ) ;
#15895=ORIENTED_EDGE ( 'NONE', *, *, #33399, .F. ) ;
#15902=DIRECTION ( 'NONE',  ( -1.000000000000000000, 1.331116318405244905E-23, 4.759647537211363479E-16 ) ) ;
#15905=EDGE_CURVE ( 'NONE', #11040, #31210, #17044, .T. ) ;
#15907=DIRECTION ( 'NONE',  ( -1.000000000000000000, 0.000000000000000000, -7.793956916774525800E-48 ) ) ;
#15909=VECTOR ( 'NONE', #43848, 1000.000000000000000 ) ;
#15912=DIRECTION ( 'NONE',  ( -1.000000000000000000, 0.000000000000000000, 0.000000000000000000 ) ) ;
#15913=ORIENTED_EDGE ( 'NONE', *, *, #28619, .F. ) ;
#15915=DIRECTION ( 'NONE',  ( -1.000000000000000000, 0.000000000000000000, 0.000000000000000000 ) ) ;
#15921=CIRCLE ( 'NONE', #35609, 2.000000000000001776 ) ;
#15928=CARTESIAN_POINT ( 'NONE',  ( 181.0000000000000284, 2.775557561562891351E-14, -115.0000000000001563 ) ) ;
#15930=DIRECTION ( 'NONE',  ( 0.000000000000000000, 1.000000000000000000, -2.969158215481698263E-48 ) ) ;
#15934=DIRECTION ( 'NONE',  ( 0.000000000000000000, -1.000000000000000000, 0.000000000000000000 ) ) ;
#15954=CARTESIAN_POINT ( 'NONE',  ( 339.9999999999999432, -180.9999999999999432, 355.9999999999998295 ) ) ;
#15957=ORIENTED_EDGE ( 'NONE', *, *, #30989, .T. ) ;
#15959=FACE_OUTER_BOUND ( 'NONE', #33853, .T. ) ;
#15965=CARTESIAN_POINT ( 'NONE',  ( 343.9999999999999432, -183.0000000000001421, -358.0000000000003411 ) ) ;
#15966=CARTESIAN_POINT ( 'NONE',  ( 349.9999999999999432, -168.9999999999999432, 355.9999999999997726 ) ) ;
#15971=DIRECTION ( 'NONE',  ( 0.000000000000000000, 0.000000000000000000, -1.000000000000000000 ) ) ;
#15973=CARTESIAN_POINT ( 'NONE',  ( -5.000000000000000000, 184.8000000000000114, -340.2000000000001592 ) ) ;
#15983=ADVANCED_FACE ( 'NONE', ( #30111 ), #5740, .F. ) ;
#15993=EDGE_CURVE ( 'NONE', #19838, #38709, #13445, .T. ) ;
#16011=CARTESIAN_POINT ( 'NONE',  ( 340.0000000000000568, 169.0000000000000000, 349.9999999999998295 ) ) ;
#16016=DIRECTION ( 'NONE',  ( -1.000000000000000000, 0.000000000000000000, 0.000000000000000000 ) ) ;
#16017=CIRCLE ( 'NONE', #24223, 2.000000000000001776 ) ;
#16020=ORIENTED_EDGE ( 'NONE', *, *, #14872, .F. ) ;
#16029=DIRECTION ( 'NONE',  ( -1.000000000000000000, -6.344131455081961406E-16, 4.759647537211363479E-16 ) ) ;
#16036=DIRECTION ( 'NONE',  ( 0.000000000000000000, -3.186989995019654210E-49, -1.000000000000000000 ) ) ;
#16037=CARTESIAN_POINT ( 'NONE',  ( 356.0000000000000000, -164.9999999999999432, 339.9999999999998295 ) ) ;
#16038=AXIS2_PLACEMENT_3D ( 'NONE', #41117, #12651, #1124 ) ;
#16043=VECTOR ( 'NONE', #35383, 1000.000000000000000 ) ;
#16044=VERTEX_POINT ( 'NONE', #9598 ) ;
#16049=DIRECTION ( 'NONE',  ( -1.586032880504786307E-16, 1.654361225106055350E-24, -1.000000000000000000 ) ) ;
#16050=AXIS2_PLACEMENT_3D ( 'NONE', #27296, #38092, #23181 ) ;
#16055=VECTOR ( 'NONE', #41713, 1000.000000000000000 ) ;
#16064=CARTESIAN_POINT ( 'NONE',  ( 339.9999999999999432, -180.9999999999999716, -342.0000000000001705 ) ) ;
#16066=ORIENTED_EDGE ( 'NONE', *, *, #26219, .T. ) ;
#16068=ORIENTED_EDGE ( 'NONE', *, *, #25027, .F. ) ;
#16071=CARTESIAN_POINT ( 'NONE',  ( 166.9999999999999716, -93.49999999999997158, -115.0000000000001563 ) ) ;
#16076=DIRECTION ( 'NONE',  ( 4.759647537211363479E-16, -5.772796816983493182E-42, 1.000000000000000000 ) ) ;
#16077=LINE ( 'NONE', #22994, #49771 ) ;
#16079=CIRCLE ( 'NONE', #27552, 2.000000000000001776 ) ;
#16081=FACE_OUTER_BOUND ( 'NONE', #29186, .T. ) ;
#16090=LINE ( 'NONE', #43780, #14068 ) ;
#16092=DIRECTION ( 'NONE',  ( -1.000000000000000000, 0.000000000000000000, 1.860490536778032451E-50 ) ) ;
#16096=ORIENTED_EDGE ( 'NONE', *, *, #3239, .F. ) ;
#16107=ORIENTED_EDGE ( 'NONE', *, *, #24683, .F. ) ;
#16114=EDGE_CURVE ( 'NONE', #33352, #20660, #6499, .T. ) ;
#16116=CARTESIAN_POINT ( 'NONE',  ( 358.3431457505075741, -185.0000000000001137, 360.0000000000000000 ) ) ;
#16118=VERTEX_POINT ( 'NONE', #11625 ) ;
#16119=ORIENTED_EDGE ( 'NONE', *, *, #50555, .T. ) ;
#16124=EDGE_CURVE ( 'NONE', #44732, #37243, #37789, .T. ) ;
#16127=CARTESIAN_POINT ( 'NONE',  ( 168.9999999999999716, -272.5000000000000000, -98.99999999999990052 ) ) ;
#16129=EDGE_CURVE ( 'NONE', #18208, #14529, #96, .T. ) ;
#16137=LINE ( 'NONE', #43823, #43727 ) ;
#16138=DIRECTION ( 'NONE',  ( 0.000000000000000000, 2.969158215481698263E-48, -1.000000000000000000 ) ) ;
#16139=AXIS2_PLACEMENT_3D ( 'NONE', #34544, #49865, #46039 ) ;
#16141=LINE ( 'NONE', #47385, #10913 ) ;
#16142=VERTEX_POINT ( 'NONE', #18544 ) ;
#16148=EDGE_CURVE ( 'NONE', #29772, #8852, #14964, .T. ) ;
#16155=DIRECTION ( 'NONE',  ( 0.000000000000000000, 5.664403186863042467E-17, 1.000000000000000000 ) ) ;
#16160=DIRECTION ( 'NONE',  ( -0.000000000000000000, -1.000000000000000000, 2.537652627714643577E-15 ) ) ;
#16162=ORIENTED_EDGE ( 'NONE', *, *, #15820, .T. ) ;
#16165=CIRCLE ( 'NONE', #9597, 4.000000000000003553 ) ;
#16171=PLANE ( 'NONE',  #18031 ) ;
#16176=DIRECTION ( 'NONE',  ( 1.000000000000000000, 0.000000000000000000, -4.758098676964956461E-16 ) ) ;
#16177=EDGE_CURVE ( 'NONE', #10936, #13504, #9928, .T. ) ;
#16178=EDGE_LOOP ( 'NONE', ( #8104, #24748, #39333, #44182 ) ) ;
#16179=AXIS2_PLACEMENT_3D ( 'NONE', #31027, #11266, #4328 ) ;
#16182=CARTESIAN_POINT ( 'NONE',  ( 185.0000000000000000, -272.4999999999999432, -356.0000000000001705 ) ) ;
#16185=DIRECTION ( 'NONE',  ( -1.000000000000000000, 0.000000000000000000, 0.000000000000000000 ) ) ;
#16186=ORIENTED_EDGE ( 'NONE', *, *, #19252, .F. ) ;
#16188=CYLINDRICAL_SURFACE ( 'NONE', #42954, 4.000000000000003553 ) ;
#16201=EDGE_CURVE ( 'NONE', #4028, #921, #22907, .T. ) ;
#16208=EDGE_CURVE ( 'NONE', #14871, #1515, #43191, .T. ) ;
#16211=ADVANCED_FACE ( 'NONE', ( #46741, #27798 ), #47254, .T. ) ;
#16214=CARTESIAN_POINT ( 'NONE',  ( 183.0000000000000000, 6.000000000000060396, -350.0000000000001705 ) ) ;
#16215=ORIENTED_EDGE ( 'NONE', *, *, #44055, .T. ) ;
#16219=CARTESIAN_POINT ( 'NONE',  ( 341.6568542494923690, -165.0000000000001421, 339.9999999999999432 ) ) ;
#16226=CARTESIAN_POINT ( 'NONE',  ( 342.8284271247458150, -182.9999999999996589, 357.9999999999995453 ) ) ;
#16231=CIRCLE ( 'NONE', #12131, 4.000000000000003553 ) ;
#16234=ORIENTED_EDGE ( 'NONE', *, *, #21826, .T. ) ;
#16239=CARTESIAN_POINT ( 'NONE',  ( 5.551115123125782702E-14, -164.9999999999999432, 355.9999999999997726 ) ) ;
#16241=LINE ( 'NONE', #39349, #47248 ) ;
#16242=VERTEX_POINT ( 'NONE', #39360 ) ;
#16244=FACE_OUTER_BOUND ( 'NONE', #7088, .T. ) ;
#16263=CARTESIAN_POINT ( 'NONE',  ( 168.9999999999999716, -272.5000000000000000, -110.9999999999999005 ) ) ;
#16265=ORIENTED_EDGE ( 'NONE', *, *, #21826, .F. ) ;
#16276=EDGE_CURVE ( 'NONE', #17553, #43423, #31914, .T. ) ;
#16287=( BOUNDED_CURVE ( )  B_SPLINE_CURVE ( 3, ( #10773, #42070, #15133, #3322 ),
 .UNSPECIFIED., .F., .F. ) 
 B_SPLINE_CURVE_WITH_KNOTS ( ( 4, 4 ),
 ( 4.712388980384693227, 6.283185307179586232 ),
 .UNSPECIFIED. ) 
 CURVE ( )  GEOMETRIC_REPRESENTATION_ITEM ( )  RATIONAL_B_SPLINE_CURVE ( ( 1.000000000000000000, 0.8047378541243658256, 0.8047378541243658256, 1.000000000000000000 ) ) 
 REPRESENTATION_ITEM ( '' )  );
#16299=FACE_OUTER_BOUND ( 'NONE', #8317, .T. ) ;
#16301=VERTEX_POINT ( 'NONE', #31670 ) ;
#16304=VERTEX_POINT ( 'NONE', #15735 ) ;
#16305=CARTESIAN_POINT ( 'NONE',  ( 169.0000000000000000, -9.999999999999953815, -95.00000000000014211 ) ) ;
#16306=VERTEX_POINT ( 'NONE', #31406 ) ;
#16308=DIRECTION ( 'NONE',  ( 0.000000000000000000, 2.969158215481698263E-48, -1.000000000000000000 ) ) ;
#16317=AXIS2_PLACEMENT_3D ( 'NONE', #18379, #30450, #33804 ) ;
#16320=DIRECTION ( 'NONE',  ( 0.000000000000000000, -1.000000000000000000, 0.000000000000000000 ) ) ;
#16335=CARTESIAN_POINT ( 'NONE',  ( 169.0000000000000000, 2.775557561562891351E-14, -95.00000000000014211 ) ) ;
#16340=LINE ( 'NONE', #31759, #29103 ) ;
#16341=ORIENTED_EDGE ( 'NONE', *, *, #46136, .T. ) ;
#16347=VECTOR ( 'NONE', #39945, 1000.000000000000000 ) ;
#16348=ORIENTED_EDGE ( 'NONE', *, *, #21401, .T. ) ;
#16356=ORIENTED_EDGE ( 'NONE', *, *, #25406, .F. ) ;
#16358=CARTESIAN_POINT ( 'NONE',  ( 343.9999999999999432, -185.0000000000001421, 360.0000000000001137 ) ) ;
#16361=ORIENTED_EDGE ( 'NONE', *, *, #4829, .F. ) ;
#16370=CARTESIAN_POINT ( 'NONE',  ( 181.0000000000000000, -7.999999999999952038, 339.9999999999998295 ) ) ;
#16386=VECTOR ( 'NONE', #4932, 1000.000000000000000 ) ;
#16387=DIRECTION ( 'NONE',  ( -1.000000000000000000, 0.000000000000000000, -1.612977847700450206E-50 ) ) ;
#16404=EDGE_CURVE ( 'NONE', #42389, #39773, #24208, .T. ) ;
#16407=DIRECTION ( 'NONE',  ( 0.000000000000000000, -1.000000000000000000, 0.000000000000000000 ) ) ;
#16409=ORIENTED_EDGE ( 'NONE', *, *, #3526, .T. ) ;
#16411=DIRECTION ( 'NONE',  ( 0.000000000000000000, 0.000000000000000000, 1.000000000000000000 ) ) ;
#16421=VECTOR ( 'NONE', #2081, 1000.000000000000000 ) ;
#16422=ORIENTED_EDGE ( 'NONE', *, *, #20259, .T. ) ;
#16428=STYLED_ITEM('',(#50747),#5102);
#16431=EDGE_CURVE ( 'NONE', #42864, #38152, #37002, .T. ) ;
#16433=EDGE_CURVE ( 'NONE', #2629, #28405, #37039, .T. ) ;
#16438=LINE ( 'NONE', #47439, #7559 ) ;
#16443=ADVANCED_FACE ( 'NONE', ( #36781 ), #1615, .T. ) ;
#16451=CARTESIAN_POINT ( 'NONE',  ( 355.9999999999999432, -174.9999999999999432, 357.9999999999998295 ) ) ;
#16458=LINE ( 'NONE', #32110, #18747 ) ;
#16462=AXIS2_PLACEMENT_3D ( 'NONE', #24436, #20318, #12610 ) ;
#16465=EDGE_CURVE ( 'NONE', #29723, #3587, #34417, .T. ) ;
#16467=EDGE_LOOP ( 'NONE', ( #859, #6754, #8654, #50640 ) ) ;
#16470=ORIENTED_EDGE ( 'NONE', *, *, #35031, .F. ) ;
#16487=ORIENTED_EDGE ( 'NONE', *, *, #7473, .T. ) ;
#16497=FACE_OUTER_BOUND ( 'NONE', #44490, .T. ) ;
#16503=VERTEX_POINT ( 'NONE', #50465 ) ;
#16504=ORIENTED_EDGE ( 'NONE', *, *, #47028, .T. ) ;
#16509=DIRECTION ( 'NONE',  ( -0.000000000000000000, -0.000000000000000000, 1.000000000000000000 ) ) ;
#16514=EDGE_LOOP ( 'NONE', ( #9172, #47643, #11001, #11258 ) ) ;
#16518=DIRECTION ( 'NONE',  ( -1.000000000000000000, 0.000000000000000000, -7.793956916774525800E-48 ) ) ;
#16522=DIRECTION ( 'NONE',  ( -1.000000000000000000, 0.000000000000000000, 0.000000000000000000 ) ) ;
#16528=EDGE_CURVE ( 'NONE', #19349, #36804, #42049, .T. ) ;
#16530=CARTESIAN_POINT ( 'NONE',  ( 164.9999999999999716, -164.9999999999999432, 355.9999999999998863 ) ) ;
#16533=VECTOR ( 'NONE', #20085, 1000.000000000000000 ) ;
#16536=VECTOR ( 'NONE', #24420, 1000.000000000000000 ) ;
#16537=PLANE ( 'NONE',  #11471 ) ;
#16548=ORIENTED_EDGE ( 'NONE', *, *, #22415, .F. ) ;
#16553=VERTEX_POINT ( 'NONE', #20228 ) ;
#16562=CARTESIAN_POINT ( 'NONE',  ( 185.0000000000000000, 6.000000000000060396, -340.0000000000001137 ) ) ;
#16564=DIRECTION ( 'NONE',  ( 0.000000000000000000, -1.000000000000000000, 0.000000000000000000 ) ) ;
#16568=( GEOMETRIC_REPRESENTATION_CONTEXT ( 3 ) GLOBAL_UNCERTAINTY_ASSIGNED_CONTEXT ( ( #31214 ) ) GLOBAL_UNIT_ASSIGNED_CONTEXT ( ( #46703, #35218, #11342 ) ) REPRESENTATION_CONTEXT ( 'NONE', 'WORKASPACE' ) );
#16569=EDGE_CURVE ( 'NONE', #4709, #19922, #31287, .T. ) ;
#16572=VERTEX_POINT ( 'NONE', #19966 ) ;
#16584=CYLINDRICAL_SURFACE ( 'NONE', #39286, 2.000000000000001776 ) ;
#16586=AXIS2_PLACEMENT_3D ( 'NONE', #40277, #5107, #20763 ) ;
#16589=ORIENTED_EDGE ( 'NONE', *, *, #30071, .T. ) ;
#16593=ORIENTED_EDGE ( 'NONE', *, *, #16177, .F. ) ;
#16595=CARTESIAN_POINT ( 'NONE',  ( 341.9999999999999432, 182.1715728752539860, -357.1715728752541281 ) ) ;
#16602=ADVANCED_FACE ( 'NONE', ( #12271 ), #24091, .T. ) ;
#16603=CARTESIAN_POINT ( 'NONE',  ( 358.0000000000001137, 182.1715728752538439, 357.1715728752535597 ) ) ;
#16606=CARTESIAN_POINT ( 'NONE',  ( -5.000000000000000000, -165.1999999999999602, -340.2000000000001592 ) ) ;
#16610=LINE ( 'NONE', #35631, #31553 ) ;
#16619=VECTOR ( 'NONE', #41849, 1000.000000000000000 ) ;
#16620=CARTESIAN_POINT ( 'NONE',  ( 343.9999999999999432, -183.0000000000002558, -358.0000000000003411 ) ) ;
#16627=CARTESIAN_POINT ( 'NONE',  ( 168.9999999999999716, -77.49999999999995737, -115.0000000000001563 ) ) ;
#16632=CARTESIAN_POINT ( 'NONE',  ( 181.0000000000000284, -174.9999999999999716, -99.00000000000014211 ) ) ;
#16641=LINE ( 'NONE', #28700, #40612 ) ;
#16646=ORIENTED_EDGE ( 'NONE', *, *, #13491, .F. ) ;
#16651=LINE ( 'NONE', #4844, #15909 ) ;
#16652=VERTEX_POINT ( 'NONE', #24349 ) ;
#16656=CARTESIAN_POINT ( 'NONE',  ( 181.0000000000000000, -272.4999999999999432, -343.9999999999999432 ) ) ;
#16657=CARTESIAN_POINT ( 'NONE',  ( 344.0000000000000000, -165.0000000000001137, -340.0000000000002842 ) ) ;
#16662=VECTOR ( 'NONE', #45808, 1000.000000000000000 ) ;
#16663=LINE ( 'NONE', #24875, #22441 ) ;
#16665=ORIENTED_EDGE ( 'NONE', *, *, #13922, .T. ) ;
#16668=( GEOMETRIC_REPRESENTATION_CONTEXT ( 3 ) GLOBAL_UNCERTAINTY_ASSIGNED_CONTEXT ( ( #38918 ) ) GLOBAL_UNIT_ASSIGNED_CONTEXT ( ( #13172, #35536, #47775 ) ) REPRESENTATION_CONTEXT ( 'NONE', 'WORKASPACE' ) );
#16686=EDGE_LOOP ( 'NONE', ( #35789, #20077, #45977, #39642 ) ) ;
#16692=CARTESIAN_POINT ( 'NONE',  ( 356.0000000000000568, 183.0000000000000853, 357.9999999999998295 ) ) ;
#16699=CARTESIAN_POINT ( 'NONE',  ( 339.9999999999999432, -169.0000000000001137, -349.9999999999998863 ) ) ;
#16701=DIRECTION ( 'NONE',  ( 0.000000000000000000, 0.000000000000000000, 1.000000000000000000 ) ) ;
#16703=CIRCLE ( 'NONE', #45349, 4.000000000000003553 ) ;
#16707=CYLINDRICAL_SURFACE ( 'NONE', #18780, 4.000000000000003553 ) ;
#16710=CARTESIAN_POINT ( 'NONE',  ( 168.9999999999999716, -95.49999999999998579, -340.0000000000001137 ) ) ;
#16712=DIRECTION ( 'NONE',  ( 0.000000000000000000, 0.000000000000000000, 1.000000000000000000 ) ) ;
#16715=VERTEX_POINT ( 'NONE', #9683 ) ;
#16719=VECTOR ( 'NONE', #36409, 1000.000000000000000 ) ;
#16722=CARTESIAN_POINT ( 'NONE',  ( 164.9999999999999716, -93.50000000000005684, -340.0000000000001137 ) ) ;
#16727=ORIENTED_EDGE ( 'NONE', *, *, #50642, .F. ) ;
#16729=PLANE ( 'NONE',  #49653 ) ;
#16749=EDGE_CURVE ( 'NONE', #40480, #36547, #13020, .T. ) ;
#16754=ADVANCED_FACE ( 'NONE', ( #28931, #36408 ), #9932, .T. ) ;
#16763=DIRECTION ( 'NONE',  ( 1.000000000000000000, -4.758098676964956461E-16, -8.975803739141899931E-48 ) ) ;
#16770=LINE ( 'NONE', #43699, #44378 ) ;
#16777=PLANE ( 'NONE',  #13040 ) ;
#16778=ORIENTED_EDGE ( 'NONE', *, *, #31586, .T. ) ;
#16782=ADVANCED_FACE ( 'NONE', ( #13269, #20989 ), #1740, .T. ) ;
#16791=DIRECTION ( 'NONE',  ( -0.000000000000000000, 1.000000000000000000, 0.000000000000000000 ) ) ;
#16794=ORIENTED_EDGE ( 'NONE', *, *, #15761, .T. ) ;
#16798=VERTEX_POINT ( 'NONE', #15320 ) ;
#16800=CARTESIAN_POINT ( 'NONE',  ( 339.9999999999998863, 181.0000000000000284, -360.0000000000003411 ) ) ;
#16802=LINE ( 'NONE', #31959, #21004 ) ;
#16803=LINE ( 'NONE', #23999, #22325 ) ;
#16804=ORIENTED_EDGE ( 'NONE', *, *, #514, .F. ) ;
#16805=CIRCLE ( 'NONE', #43007, 4.000000000000003553 ) ;
#16810=EDGE_CURVE ( 'NONE', #23987, #750, #11213, .T. ) ;
#16812=DIRECTION ( 'NONE',  ( 1.000000000000000000, -4.996003610813203446E-16, 1.033975765691284226E-24 ) ) ;
#16813=AXIS2_PLACEMENT_3D ( 'NONE', #6327, #2468, #2714 ) ;
#16819=ORIENTED_EDGE ( 'NONE', *, *, #42456, .F. ) ;
#16821=VECTOR ( 'NONE', #39120, 1000.000000000000000 ) ;
#16830=VERTEX_POINT ( 'NONE', #10439 ) ;
#16833=DIRECTION ( 'NONE',  ( 0.000000000000000000, -2.537652627714643577E-15, -1.000000000000000000 ) ) ;
#16836=EDGE_CURVE ( 'NONE', #11587, #22898, #34829, .T. ) ;
#16844=FACE_BOUND ( 'NONE', #12581, .T. ) ;
#16845=CIRCLE ( 'NONE', #3723, 4.000000000000003553 ) ;
#16849=AXIS2_PLACEMENT_3D ( 'NONE', #22187, #37854, #42424 ) ;
#16854=EDGE_CURVE ( 'NONE', #48255, #15017, #49832, .T. ) ;
#16856=FACE_OUTER_BOUND ( 'NONE', #48166, .T. ) ;
#16857=ORIENTED_EDGE ( 'NONE', *, *, #9079, .F. ) ;
#16861=EDGE_CURVE ( 'NONE', #8725, #22263, #15067, .T. ) ;
#16871=CARTESIAN_POINT ( 'NONE',  ( 344.0000000000000000, 175.0000000000000284, -94.00000000000019895 ) ) ;
#16872=CARTESIAN_POINT ( 'NONE',  ( 349.9999999999999432, -180.9999999999999716, 341.9999999999997726 ) ) ;
#16880=VERTEX_POINT ( 'NONE', #38168 ) ;
#16884=DIRECTION ( 'NONE',  ( 1.000000000000000000, 0.000000000000000000, 2.958228394578794270E-31 ) ) ;
#16890=CARTESIAN_POINT ( 'NONE',  ( 185.0000000000000000, -5.999999999999950262, 339.9999999999998295 ) ) ;
#16891=CARTESIAN_POINT ( 'NONE',  ( 350.0000000000000000, -184.9999999999999716, -344.0000000000001705 ) ) ;
#16895=DIRECTION ( 'NONE',  ( 1.000000000000000000, 0.000000000000000000, 0.000000000000000000 ) ) ;
#16904=ORIENTED_EDGE ( 'NONE', *, *, #2313, .F. ) ;
#16906=DIRECTION ( 'NONE',  ( -1.000000000000000000, 0.000000000000000000, 0.000000000000000000 ) ) ;
#16909=VERTEX_POINT ( 'NONE', #27113 ) ;
#16911=PLANE ( 'NONE',  #33863 ) ;
#16914=VECTOR ( 'NONE', #25641, 1000.000000000000000 ) ;
#16915=LINE ( 'NONE', #48155, #25394 ) ;
#16925=EDGE_CURVE ( 'NONE', #26133, #11313, #38929, .T. ) ;
#16926=ADVANCED_FACE ( 'NONE', ( #23244 ), #8628, .F. ) ;
#16932=DIRECTION ( 'NONE',  ( -1.000000000000000000, 4.996003610813203446E-16, -1.033975765691284226E-24 ) ) ;
#16933=CARTESIAN_POINT ( 'NONE',  ( 185.0000000000000000, -272.4999999999999432, -343.9999999999987494 ) ) ;
#16942=CARTESIAN_POINT ( 'NONE',  ( 350.0000000000000000, -166.9999999999999432, -344.0000000000001705 ) ) ;
#16943=VERTEX_POINT ( 'NONE', #20161 ) ;
#16955=CARTESIAN_POINT ( 'NONE',  ( -5.000000000000000000, 184.8000000000000114, -359.8000000000002387 ) ) ;
#16970=ORIENTED_EDGE ( 'NONE', *, *, #9327, .T. ) ;
#16972=ORIENTED_EDGE ( 'NONE', *, *, #25879, .F. ) ;
#16974=CARTESIAN_POINT ( 'NONE',  ( 185.0000000000000284, -174.9999999999999716, -111.0000000000001563 ) ) ;
#16981=DIRECTION ( 'NONE',  ( 1.000000000000000000, 0.000000000000000000, -0.000000000000000000 ) ) ;
#16983=DIRECTION ( 'NONE',  ( 0.000000000000000000, 0.000000000000000000, 1.000000000000000000 ) ) ;
#16992=DIRECTION ( 'NONE',  ( 0.000000000000000000, 1.000000000000000000, 3.186989995019654210E-49 ) ) ;
#16995=PLANE ( 'NONE',  #7065 ) ;
#17004=DIRECTION ( 'NONE',  ( 0.000000000000000000, -1.000000000000000000, 2.537652627714643577E-15 ) ) ;
#17005=DIRECTION ( 'NONE',  ( -1.000000000000000000, 0.000000000000000000, 0.000000000000000000 ) ) ;
#17006=DIRECTION ( 'NONE',  ( 1.000000000000000000, 0.000000000000000000, 0.000000000000000000 ) ) ;
#17009=ORIENTED_EDGE ( 'NONE', *, *, #17476, .F. ) ;
#17044=LINE ( 'NONE', #36316, #32882 ) ;
#17045=EDGE_CURVE ( 'NONE', #3886, #31711, #424, .T. ) ;
#17046=ORIENTED_EDGE ( 'NONE', *, *, #37886, .T. ) ;
#17050=DIRECTION ( 'NONE',  ( 0.000000000000000000, -1.000000000000000000, 0.000000000000000000 ) ) ;
#17052=ORIENTED_EDGE ( 'NONE', *, *, #19924, .F. ) ;
#17053=VERTEX_POINT ( 'NONE', #16071 ) ;
#17056=DIRECTION ( 'NONE',  ( -0.000000000000000000, 1.000000000000000000, 0.000000000000000000 ) ) ;
#17057=CARTESIAN_POINT ( 'NONE',  ( 341.9999999999999432, -169.0000000000001137, -349.9999999999998863 ) ) ;
#17064=ADVANCED_FACE ( 'NONE', ( #46815 ), #12461, .F. ) ;
#17072=CARTESIAN_POINT ( 'NONE',  ( 0.000000000000000000, 181.0000000000000284, 341.9999999999997726 ) ) ;
#17073=EDGE_CURVE ( 'NONE', #27540, #26544, #13217, .T. ) ;
#17074=DIRECTION ( 'NONE',  ( 1.000000000000000000, 0.000000000000000000, 0.000000000000000000 ) ) ;
#17087=ADVANCED_FACE ( 'NONE', ( #36858 ), #2187, .T. ) ;
#17092=EDGE_CURVE ( 'NONE', #921, #11040, #8911, .T. ) ;
#17098=CARTESIAN_POINT ( 'NONE',  ( 181.0000000000000284, -174.9999999999999716, -111.0000000000001563 ) ) ;
#17100=ORIENTED_EDGE ( 'NONE', *, *, #41675, .T. ) ;
#17102=EDGE_CURVE ( 'NONE', #49685, #16572, #40928, .T. ) ;
#17104=VERTEX_POINT ( 'NONE', #44253 ) ;
#17108=ORIENTED_EDGE ( 'NONE', *, *, #5599, .T. ) ;
#17114=VECTOR ( 'NONE', #8379, 1000.000000000000000 ) ;
#17121=EDGE_CURVE ( 'NONE', #14780, #7447, #49082, .T. ) ;
#17135=DIRECTION ( 'NONE',  ( 0.000000000000000000, 1.000000000000000000, 0.000000000000000000 ) ) ;
#17143=EDGE_CURVE ( 'NONE', #29017, #25893, #28378, .T. ) ;
#17150=CARTESIAN_POINT ( 'NONE',  ( 181.0000000000000000, -182.9999999999999716, -115.0000000000001279 ) ) ;
#17151=AXIS2_PLACEMENT_3D ( 'NONE', #13734, #13979, #33506 ) ;
#17152=ORIENTED_EDGE ( 'NONE', *, *, #17977, .T. ) ;
#17153=AXIS2_PLACEMENT_3D ( 'NONE', #39629, #8831, #12665 ) ;
#17155=ADVANCED_FACE ( 'NONE', ( #36346, #40179 ), #5014, .T. ) ;
#17158=DIRECTION ( 'NONE',  ( -3.363195139050033768E-16, -0.7071067811865474617, -0.7071067811865475727 ) ) ;
#17159=DIRECTION ( 'NONE',  ( 0.000000000000000000, 0.000000000000000000, -1.000000000000000000 ) ) ;
#17160=VECTOR ( 'NONE', #16387, 1000.000000000000000 ) ;
#17161=FACE_OUTER_BOUND ( 'NONE', #44945, .T. ) ;
#17162=ORIENTED_EDGE ( 'NONE', *, *, #6265, .F. ) ;
#17171=FACE_OUTER_BOUND ( 'NONE', #27795, .T. ) ;
#17173=FACE_OUTER_BOUND ( 'NONE', #6621, .T. ) ;
#17179=ORIENTED_EDGE ( 'NONE', *, *, #17960, .F. ) ;
#17196=EDGE_CURVE ( 'NONE', #26544, #19216, #6449, .T. ) ;
#17203=ORIENTED_EDGE ( 'NONE', *, *, #28126, .F. ) ;
#17211=CARTESIAN_POINT ( 'NONE',  ( -5.000000000000000000, 184.8000000000000114, -359.8000000000002387 ) ) ;
#17218=DIRECTION ( 'NONE',  ( 1.000000000000000000, 0.000000000000000000, 0.000000000000000000 ) ) ;
#17219=ORIENTED_EDGE ( 'NONE', *, *, #14183, .F. ) ;
#17228=AXIS2_PLACEMENT_3D ( 'NONE', #22639, #45196, #3128 ) ;
#17230=ORIENTED_EDGE ( 'NONE', *, *, #41579, .F. ) ;
#17236=DIRECTION ( 'NONE',  ( -1.000000000000000000, 0.000000000000000000, 0.000000000000000000 ) ) ;
#17239=VECTOR ( 'NONE', #37974, 1000.000000000000000 ) ;
#17242=CARTESIAN_POINT ( 'NONE',  ( 168.9999999999999716, -252.4999999999999432, -349.9999999999999432 ) ) ;
#17243=EDGE_CURVE ( 'NONE', #50656, #3572, #6785, .T. ) ;
#17253=DIRECTION ( 'NONE',  ( 1.000000000000000000, 0.000000000000000000, 7.793956916774525800E-48 ) ) ;
#17254=LINE ( 'NONE', #21868, #24775 ) ;
#17255=ORIENTED_EDGE ( 'NONE', *, *, #27826, .T. ) ;
#17257=ORIENTED_EDGE ( 'NONE', *, *, #14535, .T. ) ;
#17258=DIRECTION ( 'NONE',  ( -1.000000000000000000, 0.000000000000000000, 0.000000000000000000 ) ) ;
#17281=PLANE ( 'NONE',  #23217 ) ;
#17284=VERTEX_POINT ( 'NONE', #13968 ) ;
#17295=CARTESIAN_POINT ( 'NONE',  ( 344.0000000000000568, 165.0000000000000000, 349.9999999999998295 ) ) ;
#17299=ORIENTED_EDGE ( 'NONE', *, *, #50304, .F. ) ;
#17305=VERTEX_POINT ( 'NONE', #29628 ) ;
#17306=ORIENTED_EDGE ( 'NONE', *, *, #46650, .T. ) ;
#17314=ORIENTED_EDGE ( 'NONE', *, *, #25466, .T. ) ;
#17319=LINE ( 'NONE', #48324, #48733 ) ;
#17322=CYLINDRICAL_SURFACE ( 'NONE', #8820, 2.000000000000001776 ) ;
#17325=ORIENTED_EDGE ( 'NONE', *, *, #2361, .T. ) ;
#17329=VECTOR ( 'NONE', #43933, 1000.000000000000000 ) ;
#17332=CARTESIAN_POINT ( 'NONE',  ( 339.9999999999999432, 169.0000000000000000, -340.0000000000001705 ) ) ;
#17333=VECTOR ( 'NONE', #8436, 1000.000000000000000 ) ;
#17336=EDGE_CURVE ( 'NONE', #15017, #49245, #14736, .T. ) ;
#17339=AXIS2_PLACEMENT_3D ( 'NONE', #9021, #41253, #43907 ) ;
#17340=EDGE_CURVE ( 'NONE', #12862, #34493, #26292, .T. ) ;
#17355=EDGE_CURVE ( 'NONE', #16242, #34818, #28059, .T. ) ;
#17358=CARTESIAN_POINT ( 'NONE',  ( 0.000000000000000000, 165.2000000000000171, 340.1999999999997044 ) ) ;
#17362=EDGE_CURVE ( 'NONE', #17487, #3809, #7023, .T. ) ;
#17363=DIRECTION ( 'NONE',  ( 1.000000000000000000, 0.000000000000000000, 0.000000000000000000 ) ) ;
#17369=CARTESIAN_POINT ( 'NONE',  ( 339.9999999999999432, -168.9999999999999432, -356.0000000000002274 ) ) ;
#17381=CARTESIAN_POINT ( 'NONE',  ( 181.0000000000000000, -9.999999999999953815, -350.0000000000001705 ) ) ;
#17385=ADVANCED_FACE ( 'NONE', ( #47524 ), #116, .T. ) ;
#17387=AXIS2_PLACEMENT_3D ( 'NONE', #43233, #27605, #19632 ) ;
#17396=AXIS2_PLACEMENT_3D ( 'NONE', #7283, #35265, #22676 ) ;
#17397=LINE ( 'NONE', #24851, #24556 ) ;
#17398=FACE_OUTER_BOUND ( 'NONE', #8887, .T. ) ;
#17399=DIRECTION ( 'NONE',  ( 0.000000000000000000, -0.000000000000000000, 1.000000000000000000 ) ) ;
#17406=ORIENTED_EDGE ( 'NONE', *, *, #37116, .T. ) ;
#17409=CARTESIAN_POINT ( 'NONE',  ( 169.0000000000000000, -168.9999999999999432, -115.0000000000001847 ) ) ;
#17410=EDGE_LOOP ( 'NONE', ( #2221, #12143, #39517, #48413, #607, #16804, #28416, #32829 ) ) ;
#17411=FACE_OUTER_BOUND ( 'NONE', #42020, .T. ) ;
#17413=ORIENTED_EDGE ( 'NONE', *, *, #28513, .F. ) ;
#17422=DIRECTION ( 'NONE',  ( 1.000000000000000000, -4.758098676964956461E-16, -8.975803739141899931E-48 ) ) ;
#17423=ADVANCED_FACE ( 'NONE', ( #42936, #8568 ), #7816, .T. ) ;
#17425=VECTOR ( 'NONE', #38019, 1000.000000000000000 ) ;
#17427=ORIENTED_EDGE ( 'NONE', *, *, #8974, .F. ) ;
#17428=EDGE_CURVE ( 'NONE', #1861, #26957, #47119, .T. ) ;
#17429=DIRECTION ( 'NONE',  ( 0.000000000000000000, 0.000000000000000000, 1.000000000000000000 ) ) ;
#17446=AXIS2_PLACEMENT_3D ( 'NONE', #45441, #21363, #9574 ) ;
#17448=DIRECTION ( 'NONE',  ( 3.172065745548403743E-16, 1.000000000000000000, 0.000000000000000000 ) ) ;
#17454=DIRECTION ( 'NONE',  ( 7.793956916774525800E-48, 0.000000000000000000, -1.000000000000000000 ) ) ;
#17457=ORIENTED_EDGE ( 'NONE', *, *, #5098, .T. ) ;
#17463=FACE_OUTER_BOUND ( 'NONE', #6567, .T. ) ;
#17465=CARTESIAN_POINT ( 'NONE',  ( 359.9999999999998863, -183.3431457505076310, 358.3431457505074036 ) ) ;
#17472=EDGE_LOOP ( 'NONE', ( #39390, #20154, #42873, #19111, #9138, #50434, #3408, #48512 ) ) ;
#17476=EDGE_CURVE ( 'NONE', #21871, #32124, #12730, .T. ) ;
#17487=VERTEX_POINT ( 'NONE', #24725 ) ;
#17488=DIRECTION ( 'NONE',  ( 0.000000000000000000, 1.000000000000000000, 0.000000000000000000 ) ) ;
#17489=ADVANCED_FACE ( 'NONE', ( #47764 ), #36288, .T. ) ;
#17507=CARTESIAN_POINT ( 'NONE',  ( 343.9999999999999432, -174.9999999999999716, 355.9999999999998295 ) ) ;
#17510=DIRECTION ( 'NONE',  ( 1.000000000000000000, 0.000000000000000000, 7.793956916774525800E-48 ) ) ;
#17515=AXIS2_PLACEMENT_3D ( 'NONE', #31801, #32302, #1255 ) ;
#17519=CARTESIAN_POINT ( 'NONE',  ( 350.0000000000000000, -168.9999999999999432, -356.0000000000002274 ) ) ;
#17523=CARTESIAN_POINT ( 'NONE',  ( 181.0000000000000284, -9.999999999999953815, -115.0000000000001563 ) ) ;
#17527=ADVANCED_FACE ( 'NONE', ( #9569, #24473 ), #28313, .T. ) ;
#17528=VECTOR ( 'NONE', #39171, 1000.000000000000000 ) ;
#17530=ORIENTED_EDGE ( 'NONE', *, *, #11070, .F. ) ;
#17534=CARTESIAN_POINT ( 'NONE',  ( 181.0000000000000284, 2.775557561562891351E-14, -95.00000000000014211 ) ) ;
#17537=ORIENTED_EDGE ( 'NONE', *, *, #3272, .T. ) ;
#17543=AXIS2_PLACEMENT_3D ( 'NONE', #26380, #49680, #29725 ) ;
#17544=CARTESIAN_POINT ( 'NONE',  ( 340.0000000000000568, 181.0000000000000284, 355.9999999999997726 ) ) ;
#17547=ORIENTED_EDGE ( 'NONE', *, *, #41546, .F. ) ;
#17553=VERTEX_POINT ( 'NONE', #28562 ) ;
#17556=CARTESIAN_POINT ( 'NONE',  ( 181.0000000000000000, -81.49999999999997158, -350.0000000000001705 ) ) ;
#17560=ADVANCED_FACE ( 'NONE', ( #44194, #9068 ), #40372, .T. ) ;
#17561=ORIENTED_EDGE ( 'NONE', *, *, #37371, .F. ) ;
#17566=CARTESIAN_POINT ( 'NONE',  ( 0.000000000000000000, 165.2000000000000171, -340.2000000000001592 ) ) ;
#17567=DIRECTION ( 'NONE',  ( 0.000000000000000000, 1.000000000000000000, 6.123233995736766036E-17 ) ) ;
#17570=CARTESIAN_POINT ( 'NONE',  ( -5.000000000000000000, -165.1999999999999602, -340.2000000000001592 ) ) ;
#17572=EDGE_LOOP ( 'NONE', ( #10599, #8197, #24951, #32710 ) ) ;
#17584=LINE ( 'NONE', #48840, #29989 ) ;
#17592=EDGE_LOOP ( 'NONE', ( #43898, #33419, #45551, #28779 ) ) ;
#17601=DIRECTION ( 'NONE',  ( 0.000000000000000000, 1.000000000000000000, 0.000000000000000000 ) ) ;
#17606=EDGE_LOOP ( 'NONE', ( #46281, #33202, #24703, #7043 ) ) ;
#17612=EDGE_CURVE ( 'NONE', #39424, #30540, #23397, .T. ) ;
#17614=DIRECTION ( 'NONE',  ( 1.586032892321651989E-16, -3.736034562988530447E-32, 1.000000000000000000 ) ) ;
#17617=VERTEX_POINT ( 'NONE', #34197 ) ;
#17626=DIRECTION ( 'NONE',  ( 1.000000000000000000, 0.000000000000000000, 0.000000000000000000 ) ) ;
#17632=DIRECTION ( 'NONE',  ( 0.000000000000000000, 0.000000000000000000, -1.000000000000000000 ) ) ;
#17640=( BOUNDED_CURVE ( )  B_SPLINE_CURVE ( 3, ( #50722, #39000, #39250, #19473 ),
 .UNSPECIFIED., .F., .F. ) 
 B_SPLINE_CURVE_WITH_KNOTS ( ( 4, 4 ),
 ( 3.141592653589849515, 4.712388980384676351 ),
 .UNSPECIFIED. ) 
 CURVE ( )  GEOMETRIC_REPRESENTATION_ITEM ( )  RATIONAL_B_SPLINE_CURVE ( ( 1.000000000000000000, 0.8047378541243814798, 0.8047378541243814798, 1.000000000000000000 ) ) 
 REPRESENTATION_ITEM ( '' )  );
#17641=CARTESIAN_POINT ( 'NONE',  ( 344.0000000000000000, -165.0000000000001137, -349.9999999999999432 ) ) ;
#17647=LINE ( 'NONE', #26097, #47448 ) ;
#17650=VECTOR ( 'NONE', #31677, 1000.000000000000000 ) ;
#17654=DIRECTION ( 'NONE',  ( -0.000000000000000000, -1.000000000000000000, -0.000000000000000000 ) ) ;
#17665=AXIS2_PLACEMENT_3D ( 'NONE', #35756, #8790, #32131 ) ;
#17667=VERTEX_POINT ( 'NONE', #49272 ) ;
#17672=CARTESIAN_POINT ( 'NONE',  ( 357.9999999999998863, 182.1715728752540429, -357.1715728752541850 ) ) ;
#17678=EDGE_CURVE ( 'NONE', #43135, #13514, #6976, .T. ) ;
#17686=( GEOMETRIC_REPRESENTATION_CONTEXT ( 3 ) GLOBAL_UNCERTAINTY_ASSIGNED_CONTEXT ( ( #48143 ) ) GLOBAL_UNIT_ASSIGNED_CONTEXT ( ( #34954, #10557, #38791 ) ) REPRESENTATION_CONTEXT ( 'NONE', 'WORKASPACE' ) );
#17688=ORIENTED_EDGE ( 'NONE', *, *, #48355, .T. ) ;
#17689=CARTESIAN_POINT ( 'NONE',  ( 339.9999999999998863, -182.9999999999999716, 343.9999999999997726 ) ) ;
#17691=ORIENTED_EDGE ( 'NONE', *, *, #50399, .F. ) ;
#17703=ORIENTED_EDGE ( 'NONE', *, *, #15288, .F. ) ;
#17708=CIRCLE ( 'NONE', #12801, 2.000000000000001776 ) ;
#17711=CARTESIAN_POINT ( 'NONE',  ( 342.8284271247462129, 183.0000000000000853, 357.9999999999998295 ) ) ;
#17712=ORIENTED_EDGE ( 'NONE', *, *, #27489, .F. ) ;
#17713=EDGE_CURVE ( 'NONE', #3850, #28373, #29953, .T. ) ;
#17718=FACE_OUTER_BOUND ( 'NONE', #6709, .T. ) ;
#17723=ORIENTED_EDGE ( 'NONE', *, *, #27586, .F. ) ;
#17724=DIRECTION ( 'NONE',  ( -0.000000000000000000, 1.000000000000000000, 0.000000000000000000 ) ) ;
#17735=ADVANCED_FACE ( 'NONE', ( #38798 ), #23895, .T. ) ;
#17736=VERTEX_POINT ( 'NONE', #7232 ) ;
#17738=CARTESIAN_POINT ( 'NONE',  ( 181.0000000000000000, -9.999999999999953815, 339.9999999999998295 ) ) ;
#17739=LINE ( 'NONE', #33405, #40 ) ;
#17746=AXIS2_PLACEMENT_3D ( 'NONE', #42293, #38468, #6384 ) ;
#17749=CIRCLE ( 'NONE', #33322, 2.000000000000001776 ) ;
#17769=LINE ( 'NONE', #2368, #753 ) ;
#17772=EDGE_CURVE ( 'NONE', #47173, #31887, #49489, .T. ) ;
#17779=DIRECTION ( 'NONE',  ( -1.000000000000000000, 0.000000000000000000, 0.000000000000000000 ) ) ;
#17780=DIRECTION ( 'NONE',  ( 0.000000000000000000, -1.000000000000000000, -3.186989995019654210E-49 ) ) ;
#17781=ADVANCED_FACE ( 'NONE', ( #42618 ), #35209, .T. ) ;
#17783=DIRECTION ( 'NONE',  ( -2.775557561562891844E-16, 0.7071067811865473507, -0.7071067811865477948 ) ) ;
#17797=ORIENTED_EDGE ( 'NONE', *, *, #6467, .F. ) ;
#17808=EDGE_LOOP ( 'NONE', ( #46218, #13579, #664, #50489 ) ) ;
#17810=CARTESIAN_POINT ( 'NONE',  ( 356.0000000000001137, 183.0000000000000284, 349.9999999999998295 ) ) ;
#17815=ORIENTED_EDGE ( 'NONE', *, *, #281, .F. ) ;
#17816=VERTEX_POINT ( 'NONE', #3626 ) ;
#17820=DIRECTION ( 'NONE',  ( 0.000000000000000000, -1.000000000000000000, 1.544785076050074834E-48 ) ) ;
#17821=CARTESIAN_POINT ( 'NONE',  ( 0.000000000000000000, 181.0000000000000284, 339.9999999999997726 ) ) ;
#17840=EDGE_CURVE ( 'NONE', #34478, #8464, #32359, .T. ) ;
#17841=DIRECTION ( 'NONE',  ( 1.000000000000000000, 0.000000000000000000, 0.000000000000000000 ) ) ;
#17854=CARTESIAN_POINT ( 'NONE',  ( 341.9999999999999432, 181.0000000000000568, -356.0000000000002274 ) ) ;
#17857=ORIENTED_EDGE ( 'NONE', *, *, #27143, .T. ) ;
#17863=ORIENTED_EDGE ( 'NONE', *, *, #14051, .F. ) ;
#17864=DIRECTION ( 'NONE',  ( 1.132880637372608740E-16, 4.718402560806925739E-50, 1.000000000000000000 ) ) ;
#17868=LINE ( 'NONE', #49637, #43926 ) ;
#17870=VERTEX_POINT ( 'NONE', #13600 ) ;
#17883=ORIENTED_EDGE ( 'NONE', *, *, #38628, .F. ) ;
#17893=CARTESIAN_POINT ( 'NONE',  ( 183.0000000000000000, -5.999999999999950262, -340.0000000000001137 ) ) ;
#17904=DIRECTION ( 'NONE',  ( -1.000000000000000000, 0.000000000000000000, 0.000000000000000000 ) ) ;
#17910=CARTESIAN_POINT ( 'NONE',  ( 169.0000000000000284, 165.0000000000000000, 343.9999999999998863 ) ) ;
#17911=VERTEX_POINT ( 'NONE', #4886 ) ;
#17912=DIRECTION ( 'NONE',  ( 0.000000000000000000, 0.000000000000000000, -1.000000000000000000 ) ) ;
#17916=ORIENTED_EDGE ( 'NONE', *, *, #5845, .T. ) ;
#17918=DIRECTION ( 'NONE',  ( -0.000000000000000000, 1.000000000000000000, 6.123233995736766036E-17 ) ) ;
#17928=CARTESIAN_POINT ( 'NONE',  ( 168.9999999999999716, -184.9999999999999716, -350.0000000000001705 ) ) ;
#17935=AXIS2_PLACEMENT_3D ( 'NONE', #1944, #37618, #48589 ) ;
#17936=DIRECTION ( 'NONE',  ( -1.000000000000000000, 0.000000000000000000, -1.612977847700450206E-50 ) ) ;
#17940=ORIENTED_EDGE ( 'NONE', *, *, #25212, .T. ) ;
#17942=AXIS2_PLACEMENT_3D ( 'NONE', #41281, #28736, #33105 ) ;
#17944=ADVANCED_FACE ( 'NONE', ( #40555 ), #20294, .T. ) ;
#17951=EDGE_CURVE ( 'NONE', #46080, #45423, #33125, .T. ) ;
#17953=VERTEX_POINT ( 'NONE', #47698 ) ;
#17960=EDGE_CURVE ( 'NONE', #38152, #42864, #38176, .T. ) ;
#17964=EDGE_CURVE ( 'NONE', #49667, #8311, #4573, .T. ) ;
#17977=EDGE_CURVE ( 'NONE', #22263, #46472, #6653, .T. ) ;
#17978=EDGE_CURVE ( 'NONE', #9166, #34629, #50414, .T. ) ;
#17981=LINE ( 'NONE', #13134, #29212 ) ;
#17982=CARTESIAN_POINT ( 'NONE',  ( 355.9999999999999432, -183.0000000000001137, -358.0000000000003411 ) ) ;
#17983=ORIENTED_EDGE ( 'NONE', *, *, #37210, .F. ) ;
#17985=VECTOR ( 'NONE', #50004, 1000.000000000000000 ) ;
#17987=DIRECTION ( 'NONE',  ( -1.000000000000000000, 0.000000000000000000, 0.000000000000000000 ) ) ;
#17989=DIRECTION ( 'NONE',  ( -0.000000000000000000, -1.000000000000000000, 2.537652627714643577E-15 ) ) ;
#17990=CARTESIAN_POINT ( 'NONE',  ( 183.0000000000000000, -256.4999999999998295, -339.9999999999998863 ) ) ;
#17995=ORIENTED_EDGE ( 'NONE', *, *, #8948, .F. ) ;
#17998=CARTESIAN_POINT ( 'NONE',  ( 5.551115123125782702E-14, -180.9999999999999716, 339.9999999999997726 ) ) ;
#18000=EDGE_LOOP ( 'NONE', ( #19050, #24490, #6931, #49498 ) ) ;
#18003=EDGE_LOOP ( 'NONE', ( #36499, #15609, #34989, #29187, #16162, #41360, #13652, #39623 ) ) ;
#18014=EDGE_CURVE ( 'NONE', #2864, #47198, #29255, .T. ) ;
#18016=CARTESIAN_POINT ( 'NONE',  ( 0.000000000000000000, -175.0000000000000284, -346.2500000000002274 ) ) ;
#18019=CIRCLE ( 'NONE', #20520, 4.000000000000003553 ) ;
#18022=ORIENTED_EDGE ( 'NONE', *, *, #6826, .T. ) ;
#18023=FACE_OUTER_BOUND ( 'NONE', #25358, .T. ) ;
#18029=EDGE_CURVE ( 'NONE', #36234, #33463, #2553, .T. ) ;
#18030=ORIENTED_EDGE ( 'NONE', *, *, #20042, .F. ) ;
#18031=AXIS2_PLACEMENT_3D ( 'NONE', #47665, #16932, #4621 ) ;
#18038=VERTEX_POINT ( 'NONE', #44872 ) ;
#18053=ADVANCED_FACE ( 'NONE', ( #39244 ), #38734, .F. ) ;
#18056=CIRCLE ( 'NONE', #43476, 4.000000000000003553 ) ;
#18059=ORIENTED_EDGE ( 'NONE', *, *, #22742, .T. ) ;
#18061=VECTOR ( 'NONE', #36076, 1000.000000000000000 ) ;
#18063=VECTOR ( 'NONE', #3994, 1000.000000000000000 ) ;
#18064=CARTESIAN_POINT ( 'NONE',  ( 339.9999999999999432, 169.0000000000000000, -340.0000000000001705 ) ) ;
#18066=CARTESIAN_POINT ( 'NONE',  ( 168.9999999999999716, -174.9999999999999716, -360.0000000000001705 ) ) ;
#18071=CARTESIAN_POINT ( 'NONE',  ( 181.0000000000000000, -180.9999999999999716, -340.0000000000001137 ) ) ;
#18074=CARTESIAN_POINT ( 'NONE',  ( 350.0000000000001137, 165.0000000000000000, 355.9999999999997726 ) ) ;
#18089=VECTOR ( 'NONE', #24811, 1000.000000000000000 ) ;
#18095=CARTESIAN_POINT ( 'NONE',  ( 169.0000000000000000, -9.999999999999953815, -97.00000000000014211 ) ) ;
#18097=PLANE ( 'NONE',  #22534 ) ;
#18103=EDGE_CURVE ( 'NONE', #47413, #20395, #35664, .T. ) ;
#18111=EDGE_CURVE ( 'NONE', #13008, #42500, #15883, .T. ) ;
#18115=EDGE_CURVE ( 'NONE', #10975, #49733, #47138, .T. ) ;
#18117=ORIENTED_EDGE ( 'NONE', *, *, #43450, .T. ) ;
#18120=DIRECTION ( 'NONE',  ( 0.000000000000000000, 0.000000000000000000, -1.000000000000000000 ) ) ;
#18123=CYLINDRICAL_SURFACE ( 'NONE', #13122, 2.000000000000001776 ) ;
#18126=CARTESIAN_POINT ( 'NONE',  ( 168.9999999999999716, -77.49999999999997158, -340.0000000000001137 ) ) ;
#18127=EDGE_LOOP ( 'NONE', ( #49945, #12261, #32407, #15101 ) ) ;
#18128=VECTOR ( 'NONE', #39112, 1000.000000000000000 ) ;
#18149=( BOUNDED_CURVE ( )  B_SPLINE_CURVE ( 3, ( #26118, #18418, #50173, #37951 ),
 .UNSPECIFIED., .F., .F. ) 
 B_SPLINE_CURVE_WITH_KNOTS ( ( 4, 4 ),
 ( 1.570796326794889897, 3.141592653589793116 ),
 .UNSPECIFIED. ) 
 CURVE ( )  GEOMETRIC_REPRESENTATION_ITEM ( )  RATIONAL_B_SPLINE_CURVE ( ( 1.000000000000000000, 0.8047378541243634942, 0.8047378541243634942, 1.000000000000000000 ) ) 
 REPRESENTATION_ITEM ( '' )  );
#18154=CARTESIAN_POINT ( 'NONE',  ( 356.0000000000003411, -165.0000000000001137, -92.00000000000019895 ) ) ;
#18155=CIRCLE ( 'NONE', #11621, 2.000000000000001776 ) ;
#18163=CYLINDRICAL_SURFACE ( 'NONE', #24591, 4.000000000000003553 ) ;
#18167=CARTESIAN_POINT ( 'NONE',  ( 344.0000000000000568, 185.0000000000000284, 359.9999999999998295 ) ) ;
#18171=EDGE_CURVE ( 'NONE', #23604, #37534, #3823, .T. ) ;
#18176=DIRECTION ( 'NONE',  ( -1.000000000000000000, 7.930164457481157120E-16, -1.587271980518778491E-16 ) ) ;
#18177=VERTEX_POINT ( 'NONE', #39500 ) ;
#18187=DIRECTION ( 'NONE',  ( 0.000000000000000000, 0.000000000000000000, 1.000000000000000000 ) ) ;
#18197=DIRECTION ( 'NONE',  ( 1.000000000000000000, -4.758098676964957447E-16, 2.958228394578795584E-31 ) ) ;
#18208=VERTEX_POINT ( 'NONE', #17332 ) ;
#18214=VECTOR ( 'NONE', #88, 1000.000000000000000 ) ;
#18216=ORIENTED_EDGE ( 'NONE', *, *, #27908, .F. ) ;
#18223=CARTESIAN_POINT ( 'NONE',  ( 165.0000000000000284, 175.0000000000000284, 343.9999999999998863 ) ) ;
#18224=VECTOR ( 'NONE', #3875, 1000.000000000000000 ) ;
#18227=ORIENTED_EDGE ( 'NONE', *, *, #5417, .F. ) ;
#18229=VECTOR ( 'NONE', #24924, 1000.000000000000000 ) ;
#18231=AXIS2_PLACEMENT_3D ( 'NONE', #27816, #43205, #36033 ) ;
#18232=LINE ( 'NONE', #14648, #30833 ) ;
#18233=DIRECTION ( 'NONE',  ( 0.000000000000000000, 0.000000000000000000, -1.000000000000000000 ) ) ;
#18234=ORIENTED_EDGE ( 'NONE', *, *, #13012, .F. ) ;
#18247=ADVANCED_FACE ( 'NONE', ( #2194 ), #36617, .T. ) ;
#18249=EDGE_CURVE ( 'NONE', #4473, #31718, #10738, .T. ) ;
#18250=ORIENTED_EDGE ( 'NONE', *, *, #16749, .T. ) ;
#18254=DIRECTION ( 'NONE',  ( -1.612977847700450206E-50, 0.000000000000000000, -1.000000000000000000 ) ) ;
#18263=ADVANCED_FACE ( 'NONE', ( #40440 ), #25793, .F. ) ;
#18268=AXIS2_PLACEMENT_3D ( 'NONE', #15629, #31555, #35408 ) ;
#18272=CARTESIAN_POINT ( 'NONE',  ( 339.9999999999999432, -181.0000000000001421, 356.0000000000000000 ) ) ;
#18281=ADVANCED_FACE ( 'NONE', ( #13975 ), #33503, .T. ) ;
#18282=PLANE ( 'NONE',  #48012 ) ;
#18285=VERTEX_POINT ( 'NONE', #48335 ) ;
#18289=CARTESIAN_POINT ( 'NONE',  ( 168.9999999999999716, -268.5000000000000000, -114.9999999999999147 ) ) ;
#18291=CARTESIAN_POINT ( 'NONE',  ( 0.000000000000000000, 175.0000000000000284, -350.0000000000002274 ) ) ;
#18297=AXIS2_PLACEMENT_3D ( 'NONE', #15966, #24932, #16712 ) ;
#18315=DIRECTION ( 'NONE',  ( -1.000000000000000000, 0.000000000000000000, -1.612977847700450206E-50 ) ) ;
#18318=DIRECTION ( 'NONE',  ( 1.000000000000000000, 0.000000000000000000, 0.000000000000000000 ) ) ;
#18320=CARTESIAN_POINT ( 'NONE',  ( 0.000000000000000000, 165.2000000000000171, 359.7999999999997840 ) ) ;
#18322=EDGE_CURVE ( 'NONE', #40029, #38870, #17584, .T. ) ;
#18333=AXIS2_PLACEMENT_3D ( 'NONE', #19466, #35151, #42313 ) ;
#18343=ADVANCED_FACE ( 'NONE', ( #46009 ), #10895, .T. ) ;
#18347=VECTOR ( 'NONE', #29197, 1000.000000000000000 ) ;
#18353=LINE ( 'NONE', #28724, #47150 ) ;
#18363=FACE_OUTER_BOUND ( 'NONE', #22260, .T. ) ;
#18365=AXIS2_PLACEMENT_3D ( 'NONE', #20962, #32766, #37141 ) ;
#18367=VERTEX_POINT ( 'NONE', #34005 ) ;
#18368=CARTESIAN_POINT ( 'NONE',  ( 169.0000000000000000, -174.9999999999999716, -99.00000000000014211 ) ) ;
#18369=AXIS2_PLACEMENT_3D ( 'NONE', #68, #20061, #825 ) ;
#18375=AXIS2_PLACEMENT_3D ( 'NONE', #40606, #4935, #48755 ) ;
#18379=CARTESIAN_POINT ( 'NONE',  ( 340.0000000000000568, 169.0000000000000000, 355.9999999999997726 ) ) ;
#18389=VECTOR ( 'NONE', #2610, 1000.000000000000000 ) ;
#18399=EDGE_CURVE ( 'NONE', #45613, #49664, #45752, .T. ) ;
#18400=EDGE_LOOP ( 'NONE', ( #35592, #11030, #9767, #22688 ) ) ;
#18404=ORIENTED_EDGE ( 'NONE', *, *, #9852, .F. ) ;
#18418=CARTESIAN_POINT ( 'NONE',  ( 359.9999999999998863, -183.3431457505077447, -358.3431457505079152 ) ) ;
#18423=DIRECTION ( 'NONE',  ( -0.000000000000000000, -1.000000000000000000, -0.000000000000000000 ) ) ;
#18428=CARTESIAN_POINT ( 'NONE',  ( 165.0000000000000284, 165.0000000000000000, 343.9999999999998863 ) ) ;
#18429=EDGE_LOOP ( 'NONE', ( #2341, #36627, #46675, #39223 ) ) ;
#18430=CIRCLE ( 'NONE', #48683, 2.000000000000001776 ) ;
#18432=ORIENTED_EDGE ( 'NONE', *, *, #11462, .F. ) ;
#18440=( GEOMETRIC_REPRESENTATION_CONTEXT ( 3 ) GLOBAL_UNCERTAINTY_ASSIGNED_CONTEXT ( ( #28691 ) ) GLOBAL_UNIT_ASSIGNED_CONTEXT ( ( #22748, #2491, #49397 ) ) REPRESENTATION_CONTEXT ( 'NONE', 'WORKASPACE' ) );
#18443=ORIENTED_EDGE ( 'NONE', *, *, #11250, .T. ) ;
#18444=AXIS2_PLACEMENT_3D ( 'NONE', #43292, #8164, #24069 ) ;
#18445=CARTESIAN_POINT ( 'NONE',  ( 168.9999999999999716, -9.999999999999953815, 339.9999999999998295 ) ) ;
#18446=CARTESIAN_POINT ( 'NONE',  ( 344.0000000000001705, 165.0000000000000000, -340.0000000000001137 ) ) ;
#18448=AXIS2_PLACEMENT_3D ( 'NONE', #28191, #20472, #16895 ) ;
#18451=DIRECTION ( 'NONE',  ( -1.586032880504786307E-16, 1.654361225106055350E-24, -1.000000000000000000 ) ) ;
#18465=ORIENTED_EDGE ( 'NONE', *, *, #17951, .F. ) ;
#18470=AXIS2_PLACEMENT_3D ( 'NONE', #3496, #15064, #31491 ) ;
#18475=VERTEX_POINT ( 'NONE', #20362 ) ;
#18483=DIRECTION ( 'NONE',  ( 0.000000000000000000, 0.000000000000000000, 1.000000000000000000 ) ) ;
#18488=ORIENTED_EDGE ( 'NONE', *, *, #47983, .T. ) ;
#18491=CIRCLE ( 'NONE', #20144, 2.000000000000001776 ) ;
#18502=CARTESIAN_POINT ( 'NONE',  ( 185.0000000000000000, -180.9999999999999716, -340.0000000000000000 ) ) ;
#18523=DIRECTION ( 'NONE',  ( 3.172065784643302499E-16, 1.000000000000000000, 0.000000000000000000 ) ) ;
#18527=ORIENTED_EDGE ( 'NONE', *, *, #8043, .F. ) ;
#18530=CARTESIAN_POINT ( 'NONE',  ( 0.000000000000000000, 181.0000000000000284, -356.0000000000002274 ) ) ;
#18540=ORIENTED_EDGE ( 'NONE', *, *, #43072, .T. ) ;
#18541=ORIENTED_EDGE ( 'NONE', *, *, #4808, .F. ) ;
#18544=CARTESIAN_POINT ( 'NONE',  ( 185.0000000000000284, -180.9999999999999716, -115.0000000000001563 ) ) ;
#18545=AXIS2_PLACEMENT_3D ( 'NONE', #35, #34944, #4865 ) ;
#18555=VECTOR ( 'NONE', #22782, 1000.000000000000000 ) ;
#18561=DIRECTION ( 'NONE',  ( -7.793956916774525800E-48, 0.000000000000000000, -1.000000000000000000 ) ) ;
#18563=VERTEX_POINT ( 'NONE', #40130 ) ;
#18567=( NAMED_UNIT ( * ) PLANE_ANGLE_UNIT ( ) SI_UNIT ( $, .RADIAN. ) );
#18568=EDGE_LOOP ( 'NONE', ( #771, #716, #47779, #5659 ) ) ;
#18573=AXIS2_PLACEMENT_3D ( 'NONE', #29236, #9723, #14075 ) ;
#18583=EDGE_CURVE ( 'NONE', #39773, #8719, #9815, .T. ) ;
#18587=CIRCLE ( 'NONE', #31745, 2.000000000000001776 ) ;
#18589=ADVANCED_FACE ( 'NONE', ( #48274 ), #13674, .F. ) ;
#18598=EDGE_CURVE ( 'NONE', #34262, #41902, #43819, .T. ) ;
#18608=EDGE_CURVE ( 'NONE', #41044, #49858, #13907, .T. ) ;
#18609=CARTESIAN_POINT ( 'NONE',  ( 181.0000000000000000, 175.0000000000000284, -358.0000000000001705 ) ) ;
#18610=CARTESIAN_POINT ( 'NONE',  ( 358.0000000000001137, 181.0000000000000284, 349.9999999999998295 ) ) ;
#18611=CARTESIAN_POINT ( 'NONE',  ( 339.9999999999999432, 181.0000000000000284, -340.0000000000001705 ) ) ;
#18613=ORIENTED_EDGE ( 'NONE', *, *, #18678, .F. ) ;
#18621=EDGE_CURVE ( 'NONE', #3854, #37848, #44201, .T. ) ;
#18623=EDGE_CURVE ( 'NONE', #13304, #8209, #27462, .T. ) ;
#18627=LINE ( 'NONE', #22985, #28863 ) ;
#18628=CARTESIAN_POINT ( 'NONE',  ( 339.9999999999998863, -174.9999999999999432, 359.9999999999998295 ) ) ;
#18630=LINE ( 'NONE', #37917, #43743 ) ;
#18631=ORIENTED_EDGE ( 'NONE', *, *, #39994, .F. ) ;
#18632=DIRECTION ( 'NONE',  ( 1.000000000000000000, 0.000000000000000000, -4.758098676964956461E-16 ) ) ;
#18633=LINE ( 'NONE', #30454, #13586 ) ;
#18634=CARTESIAN_POINT ( 'NONE',  ( -5.000000000000000000, -184.7999999999999545, -340.2000000000001592 ) ) ;
#18635=CARTESIAN_POINT ( 'NONE',  ( 356.0000000000001137, 165.0000000000000000, 339.9999999999998295 ) ) ;
#18636=EDGE_CURVE ( 'NONE', #2097, #23500, #48526, .T. ) ;
#18641=DIRECTION ( 'NONE',  ( -3.172065784643302499E-16, -1.000000000000000000, 2.537652627714642000E-15 ) ) ;
#18642=ORIENTED_EDGE ( 'NONE', *, *, #35450, .T. ) ;
#18650=CARTESIAN_POINT ( 'NONE',  ( 356.0000000000000000, -167.0000000000001137, -342.0000000000003411 ) ) ;
#18651=VERTEX_POINT ( 'NONE', #34450 ) ;
#18652=CARTESIAN_POINT ( 'NONE',  ( 166.9999999999999716, 6.000000000000060396, 339.9999999999998295 ) ) ;
#18657=CIRCLE ( 'NONE', #34253, 2.000000000000001776 ) ;
#18661=ORIENTED_EDGE ( 'NONE', *, *, #48203, .T. ) ;
#18664=ORIENTED_EDGE ( 'NONE', *, *, #21142, .T. ) ;
#18667=LINE ( 'NONE', #26637, #20419 ) ;
#18671=ORIENTED_EDGE ( 'NONE', *, *, #12661, .F. ) ;
#18675=LINE ( 'NONE', #41534, #2898 ) ;
#18676=EDGE_CURVE ( 'NONE', #46047, #27092, #18430, .T. ) ;
#18678=EDGE_CURVE ( 'NONE', #45390, #44283, #6728, .T. ) ;
#18680=CARTESIAN_POINT ( 'NONE',  ( 357.1715728752537871, -167.0000000000001137, -342.0000000000003411 ) ) ;
#18681=DIRECTION ( 'NONE',  ( -1.000000000000000000, -0.000000000000000000, -0.000000000000000000 ) ) ;
#18686=EDGE_CURVE ( 'NONE', #21143, #48323, #38049, .T. ) ;
#18697=FACE_OUTER_BOUND ( 'NONE', #30629, .T. ) ;
#18698=DIRECTION ( 'NONE',  ( 0.000000000000000000, -2.265761274745217480E-16, 1.000000000000000000 ) ) ;
#18701=CARTESIAN_POINT ( 'NONE',  ( 343.9999999999999432, -174.9999999999999432, 357.9999999999998295 ) ) ;
#18703=CARTESIAN_POINT ( 'NONE',  ( 343.9999999999999432, -174.9999999999999716, 355.9999999999998295 ) ) ;
#18710=DIRECTION ( 'NONE',  ( 1.000000000000000000, 0.000000000000000000, -1.860490536778032451E-50 ) ) ;
#18711=VERTEX_POINT ( 'NONE', #6238 ) ;
#18716=ORIENTED_EDGE ( 'NONE', *, *, #9412, .F. ) ;
#18727=VERTEX_POINT ( 'NONE', #45446 ) ;
#18729=DIRECTION ( 'NONE',  ( 0.000000000000000000, 0.000000000000000000, -1.000000000000000000 ) ) ;
#18735=VERTEX_POINT ( 'NONE', #14162 ) ;
#18739=VERTEX_POINT ( 'NONE', #18016 ) ;
#18741=ADVANCED_FACE ( 'NONE', ( #22131 ), #37805, .T. ) ;
#18747=VECTOR ( 'NONE', #8772, 1000.000000000000000 ) ;
#18749=( BOUNDED_CURVE ( )  B_SPLINE_CURVE ( 3, ( #12153, #43438, #44188, #28052 ),
 .UNSPECIFIED., .F., .F. ) 
 B_SPLINE_CURVE_WITH_KNOTS ( ( 4, 4 ),
 ( 1.586958686267291678E-16, 1.570796326794889675 ),
 .UNSPECIFIED. ) 
 CURVE ( )  GEOMETRIC_REPRESENTATION_ITEM ( )  RATIONAL_B_SPLINE_CURVE ( ( 1.000000000000000000, 0.8047378541243667138, 0.8047378541243667138, 1.000000000000000000 ) ) 
 REPRESENTATION_ITEM ( '' )  );
#18761=CARTESIAN_POINT ( 'NONE',  ( 168.9999999999997158, -164.9999999999999432, 359.9999999999997726 ) ) ;
#18763=LINE ( 'NONE', #34444, #37381 ) ;
#18772=ORIENTED_EDGE ( 'NONE', *, *, #32419, .F. ) ;
#18774=ORIENTED_EDGE ( 'NONE', *, *, #12370, .F. ) ;
#18780=AXIS2_PLACEMENT_3D ( 'NONE', #28521, #8522, #44636 ) ;
#18783=EDGE_LOOP ( 'NONE', ( #32107, #7019, #3751, #23623, #35278, #36588, #37252, #33726 ) ) ;
#18786=MECHANICAL_DESIGN_GEOMETRIC_PRESENTATION_REPRESENTATION('',(#12248),#4048);
#18793=VERTEX_POINT ( 'NONE', #23399 ) ;
#18795=CARTESIAN_POINT ( 'NONE',  ( 165.0000000000000000, -174.9999999999999716, -99.00000000000014211 ) ) ;
#18799=CARTESIAN_POINT ( 'NONE',  ( 185.0000000000000000, -268.4999999999999432, -349.9999999999999432 ) ) ;
#18812=CARTESIAN_POINT ( 'NONE',  ( 168.9999999999999716, -81.49999999999995737, -115.0000000000001563 ) ) ;
#18814=EDGE_LOOP ( 'NONE', ( #12432, #29874, #47875, #15530 ) ) ;
#18818=ORIENTED_EDGE ( 'NONE', *, *, #46631, .F. ) ;
#18833=DIRECTION ( 'NONE',  ( 1.000000000000000000, 0.000000000000000000, 0.000000000000000000 ) ) ;
#18835=CARTESIAN_POINT ( 'NONE',  ( 355.9999999999999432, -185.0000000000001421, -349.9999999999998863 ) ) ;
#18842=ORIENTED_EDGE ( 'NONE', *, *, #18115, .T. ) ;
#18850=LINE ( 'NONE', #399, #3441 ) ;
#18854=ORIENTED_EDGE ( 'NONE', *, *, #8255, .T. ) ;
#18858=PLANE ( 'NONE',  #33203 ) ;
#18859=DIRECTION ( 'NONE',  ( -1.586032880504786307E-16, 1.654361225106055350E-24, -1.000000000000000000 ) ) ;
#18862=PLANE ( 'NONE',  #16139 ) ;
#18865=ORIENTED_EDGE ( 'NONE', *, *, #32958, .F. ) ;
#18866=ORIENTED_EDGE ( 'NONE', *, *, #12308, .F. ) ;
#18867=DIRECTION ( 'NONE',  ( -0.000000000000000000, 0.000000000000000000, 1.000000000000000000 ) ) ;
#18871=CARTESIAN_POINT ( 'NONE',  ( 355.9999999999999432, -183.0000000000000000, 357.9999999999998295 ) ) ;
#18873=ORIENTED_EDGE ( 'NONE', *, *, #42429, .F. ) ;
#18875=DIRECTION ( 'NONE',  ( -1.000000000000000000, 0.000000000000000000, 1.860490536778032451E-50 ) ) ;
#18878=CARTESIAN_POINT ( 'NONE',  ( 339.9999999999999432, -181.0000000000001421, 356.0000000000000000 ) ) ;
#18879=EDGE_LOOP ( 'NONE', ( #34853, #6116, #5968, #33037 ) ) ;
#18882=LINE ( 'NONE', #46818, #48787 ) ;
#18891=CARTESIAN_POINT ( 'NONE',  ( 341.9999999999999432, -167.8284271247463266, 342.8284271247462129 ) ) ;
#18893=CARTESIAN_POINT ( 'NONE',  ( 169.0000000000000000, -9.999999999999953815, -115.0000000000001563 ) ) ;
#18895=CIRCLE ( 'NONE', #6644, 4.000000000000003553 ) ;
#18898=DIRECTION ( 'NONE',  ( 1.000000000000000000, 0.000000000000000000, 0.000000000000000000 ) ) ;
#18899=EDGE_CURVE ( 'NONE', #19563, #34472, #35216, .T. ) ;
#18900=ORIENTED_EDGE ( 'NONE', *, *, #28320, .T. ) ;
#18901=DIRECTION ( 'NONE',  ( 0.000000000000000000, 0.000000000000000000, 1.000000000000000000 ) ) ;
#18905=CARTESIAN_POINT ( 'NONE',  ( 181.0000000000000284, -174.9999999999999716, -95.00000000000014211 ) ) ;
#18909=ADVANCED_FACE ( 'NONE', ( #27752 ), #318, .F. ) ;
#18910=ORIENTED_EDGE ( 'NONE', *, *, #2270, .T. ) ;
#18912=ORIENTED_EDGE ( 'NONE', *, *, #46773, .F. ) ;
#18925=EDGE_CURVE ( 'NONE', #15814, #22226, #5148, .T. ) ;
#18935=VECTOR ( 'NONE', #22665, 1000.000000000000000 ) ;
#18944=DIRECTION ( 'NONE',  ( 0.000000000000000000, 0.000000000000000000, -1.000000000000000000 ) ) ;
#18956=DIRECTION ( 'NONE',  ( -0.000000000000000000, -0.000000000000000000, 1.000000000000000000 ) ) ;
#18969=AXIS2_PLACEMENT_3D ( 'NONE', #23131, #19278, #22881 ) ;
#18974=CARTESIAN_POINT ( 'NONE',  ( 360.0000000000001137, 181.0000000000000568, 355.9999999999998863 ) ) ;
#18979=ORIENTED_EDGE ( 'NONE', *, *, #11462, .T. ) ;
#18986=EDGE_LOOP ( 'NONE', ( #46496, #2379, #40893, #34735 ) ) ;
#18991=EDGE_CURVE ( 'NONE', #22723, #2845, #16805, .T. ) ;
#18996=AXIS2_PLACEMENT_3D ( 'NONE', #3612, #7991, #8240 ) ;
#19005=DIRECTION ( 'NONE',  ( -1.000000000000000000, 3.172065799423185948E-16, -1.587271980518778491E-16 ) ) ;
#19006=DIRECTION ( 'NONE',  ( 0.000000000000000000, 0.000000000000000000, -1.000000000000000000 ) ) ;
#19016=ADVANCED_FACE ( 'NONE', ( #25166 ), #1063, .F. ) ;
#19026=VERTEX_POINT ( 'NONE', #25676 ) ;
#19034=CARTESIAN_POINT ( 'NONE',  ( 183.0000000000000000, 165.0000000000000000, -356.0000000000001705 ) ) ;
#19035=EDGE_CURVE ( 'NONE', #2059, #1045, #22063, .T. ) ;
#19041=CYLINDRICAL_SURFACE ( 'NONE', #40109, 2.000000000000001776 ) ;
#19043=DIRECTION ( 'NONE',  ( 0.000000000000000000, 0.000000000000000000, -1.000000000000000000 ) ) ;
#19046=CARTESIAN_POINT ( 'NONE',  ( 168.9999999999999716, 175.0000000000000284, -340.0000000000001137 ) ) ;
#19050=ORIENTED_EDGE ( 'NONE', *, *, #23298, .F. ) ;
#19051=LINE ( 'NONE', #34737, #15285 ) ;
#19054=ORIENTED_EDGE ( 'NONE', *, *, #30867, .F. ) ;
#19058=VERTEX_POINT ( 'NONE', #14367 ) ;
#19064=CARTESIAN_POINT ( 'NONE',  ( 183.0000000000000568, 165.0000000000000000, 343.9999999999998863 ) ) ;
#19065=ORIENTED_EDGE ( 'NONE', *, *, #44400, .F. ) ;
#19066=ORIENTED_EDGE ( 'NONE', *, *, #27908, .T. ) ;
#19069=LINE ( 'NONE', #42926, #34111 ) ;
#19076=FACE_OUTER_BOUND ( 'NONE', #30529, .T. ) ;
#19078=CARTESIAN_POINT ( 'NONE',  ( 344.0000000000000000, 175.0000000000000284, -90.00000000000018474 ) ) ;
#19079=CARTESIAN_POINT ( 'NONE',  ( 340.0000000000000000, -178.0000000000000284, 2.999999999999891642 ) ) ;
#19081=DIRECTION ( 'NONE',  ( 1.000000000000000000, 0.000000000000000000, -1.132880637372608740E-16 ) ) ;
#19084=DIRECTION ( 'NONE',  ( 0.000000000000000000, 1.000000000000000000, 1.544785076050074834E-48 ) ) ;
#19088=ADVANCED_FACE ( 'NONE', ( #17718 ), #3063, .F. ) ;
#19094=CYLINDRICAL_SURFACE ( 'NONE', #29575, 4.000000000000003553 ) ;
#19103=AXIS2_PLACEMENT_3D ( 'NONE', #20415, #16076, #8635 ) ;
#19104=ORIENTED_EDGE ( 'NONE', *, *, #33616, .F. ) ;
#19111=ORIENTED_EDGE ( 'NONE', *, *, #18676, .F. ) ;
#19112=PLANE ( 'NONE',  #4115 ) ;
#19114=DIRECTION ( 'NONE',  ( -1.000000000000000000, -0.000000000000000000, -0.000000000000000000 ) ) ;
#19122=VERTEX_POINT ( 'NONE', #50483 ) ;
#19126=DIRECTION ( 'NONE',  ( -1.586032892321652236E-16, -1.000000000000000000, -2.288264760618012091E-48 ) ) ;
#19133=ORIENTED_EDGE ( 'NONE', *, *, #42278, .T. ) ;
#19141=ORIENTED_EDGE ( 'NONE', *, *, #33491, .F. ) ;
#19161=FACE_BOUND ( 'NONE', #21587, .T. ) ;
#19163=VERTEX_POINT ( 'NONE', #43325 ) ;
#19173=UNCERTAINTY_MEASURE_WITH_UNIT (LENGTH_MEASURE( 1.000000000000000082E-05 ), #49131, 'distance_accuracy_value', 'NONE');
#19182=ORIENTED_EDGE ( 'NONE', *, *, #28383, .T. ) ;
#19185=VERTEX_POINT ( 'NONE', #30791 ) ;
#19186=ORIENTED_EDGE ( 'NONE', *, *, #43464, .T. ) ;
#19190=ORIENTED_EDGE ( 'NONE', *, *, #4534, .T. ) ;
#19206=AXIS2_PLACEMENT_3D ( 'NONE', #23929, #42909, #50571 ) ;
#19207=CARTESIAN_POINT ( 'NONE',  ( 166.9999999999999716, 175.0000000000000284, -344.0000000000001137 ) ) ;
#19216=VERTEX_POINT ( 'NONE', #8202 ) ;
#19218=ORIENTED_EDGE ( 'NONE', *, *, #43560, .F. ) ;
#19222=DIRECTION ( 'NONE',  ( -1.000000000000000000, 0.000000000000000000, -1.612977847700450206E-50 ) ) ;
#19225=ORIENTED_EDGE ( 'NONE', *, *, #44011, .F. ) ;
#19226=CARTESIAN_POINT ( 'NONE',  ( 168.9999999999999716, -93.49999999999998579, -340.0000000000001137 ) ) ;
#19231=EDGE_LOOP ( 'NONE', ( #7719, #38778, #7927, #16794 ) ) ;
#19239=ORIENTED_EDGE ( 'NONE', *, *, #8080, .F. ) ;
#19242=DIRECTION ( 'NONE',  ( 0.000000000000000000, -0.000000000000000000, -1.000000000000000000 ) ) ;
#19248=CARTESIAN_POINT ( 'NONE',  ( 185.0000000000000284, -9.999999999999953815, -99.00000000000014211 ) ) ;
#19251=VERTEX_POINT ( 'NONE', #34643 ) ;
#19252=EDGE_CURVE ( 'NONE', #26847, #27608, #17640, .T. ) ;
#19256=DIRECTION ( 'NONE',  ( -1.000000000000000000, 0.000000000000000000, -1.612977847700450206E-50 ) ) ;
#19262=DIRECTION ( 'NONE',  ( 0.000000000000000000, 0.000000000000000000, -1.000000000000000000 ) ) ;
#19278=DIRECTION ( 'NONE',  ( -0.000000000000000000, -0.000000000000000000, 1.000000000000000000 ) ) ;
#19287=ORIENTED_EDGE ( 'NONE', *, *, #32868, .T. ) ;
#19289=DIRECTION ( 'NONE',  ( 0.000000000000000000, 3.186989995019654210E-49, 1.000000000000000000 ) ) ;
#19291=DIRECTION ( 'NONE',  ( 0.000000000000000000, -1.000000000000000000, 0.000000000000000000 ) ) ;
#19292=EDGE_LOOP ( 'NONE', ( #626, #43737, #1800, #1833 ) ) ;
#19299=LINE ( 'NONE', #19805, #33551 ) ;
#19301=VERTEX_POINT ( 'NONE', #40756 ) ;
#19302=CARTESIAN_POINT ( 'NONE',  ( 344.0000000000000000, -167.0000000000001137, -342.0000000000002842 ) ) ;
#19306=ADVANCED_FACE ( 'NONE', ( #17398 ), #32817, .F. ) ;
#19307=ORIENTED_EDGE ( 'NONE', *, *, #5775, .T. ) ;
#19308=ORIENTED_EDGE ( 'NONE', *, *, #23170, .T. ) ;
#19310=DIRECTION ( 'NONE',  ( 1.000000000000000000, 0.000000000000000000, -4.758098676964956461E-16 ) ) ;
#19314=PLANE ( 'NONE',  #30699 ) ;
#19315=DIRECTION ( 'NONE',  ( 0.000000000000000000, 1.000000000000000000, 0.000000000000000000 ) ) ;
#19316=CARTESIAN_POINT ( 'NONE',  ( 0.000000000000000000, -180.9999999999999716, -360.0000000000002274 ) ) ;
#19323=LINE ( 'NONE', #27286, #9937 ) ;
#19326=VECTOR ( 'NONE', #48926, 1000.000000000000000 ) ;
#19336=ORIENTED_EDGE ( 'NONE', *, *, #5136, .T. ) ;
#19337=FACE_OUTER_BOUND ( 'NONE', #21688, .T. ) ;
#19338=ORIENTED_EDGE ( 'NONE', *, *, #3312, .T. ) ;
#19340=EDGE_CURVE ( 'NONE', #11545, #16553, #16641, .T. ) ;
#19346=DIRECTION ( 'NONE',  ( -1.000000000000000000, 0.000000000000000000, 0.000000000000000000 ) ) ;
#19349=VERTEX_POINT ( 'NONE', #28947 ) ;
#19355=VECTOR ( 'NONE', #1908, 1000.000000000000000 ) ;
#19356=DIRECTION ( 'NONE',  ( 0.000000000000000000, 0.000000000000000000, 1.000000000000000000 ) ) ;
#19357=VECTOR ( 'NONE', #43924, 1000.000000000000000 ) ;
#19361=ORIENTED_EDGE ( 'NONE', *, *, #24269, .T. ) ;
#19371=ORIENTED_EDGE ( 'NONE', *, *, #50234, .T. ) ;
#19372=CARTESIAN_POINT ( 'NONE',  ( 183.0000000000000284, 2.775557561562891351E-14, -111.0000000000001563 ) ) ;
#19375=ORIENTED_EDGE ( 'NONE', *, *, #18014, .T. ) ;
#19381=ORIENTED_EDGE ( 'NONE', *, *, #44019, .T. ) ;
#19393=ORIENTED_EDGE ( 'NONE', *, *, #49158, .T. ) ;
#19394=CARTESIAN_POINT ( 'NONE',  ( -5.000000000000000000, 184.8000000000000114, 359.7999999999997840 ) ) ;
#19399=ORIENTED_EDGE ( 'NONE', *, *, #35137, .T. ) ;
#19414=EDGE_CURVE ( 'NONE', #50507, #10238, #41004, .T. ) ;
#19417=VECTOR ( 'NONE', #9157, 1000.000000000000000 ) ;
#19418=CARTESIAN_POINT ( 'NONE',  ( 5.551115123125782702E-14, -166.9999999999999432, 343.9999999999997726 ) ) ;
#19423=ORIENTED_EDGE ( 'NONE', *, *, #25632, .T. ) ;
#19432=ORIENTED_EDGE ( 'NONE', *, *, #45121, .T. ) ;
#19438=ORIENTED_EDGE ( 'NONE', *, *, #31542, .T. ) ;
#19439=LINE ( 'NONE', #22778, #40160 ) ;
#19449=ORIENTED_EDGE ( 'NONE', *, *, #48139, .T. ) ;
#19455=( NAMED_UNIT ( * ) PLANE_ANGLE_UNIT ( ) SI_UNIT ( $, .RADIAN. ) );
#19462=ADVANCED_FACE ( 'NONE', ( #49411 ), #48899, .T. ) ;
#19465=ORIENTED_EDGE ( 'NONE', *, *, #17951, .T. ) ;
#19466=CARTESIAN_POINT ( 'NONE',  ( 349.9999999999999432, -180.9999999999999716, 355.9999999999997726 ) ) ;
#19467=DIRECTION ( 'NONE',  ( 0.000000000000000000, 5.664403186863042467E-17, 1.000000000000000000 ) ) ;
#19469=CARTESIAN_POINT ( 'NONE',  ( -5.000000000000000000, -184.7999999999999545, -359.8000000000002387 ) ) ;
#19470=ORIENTED_EDGE ( 'NONE', *, *, #40387, .T. ) ;
#19471=CARTESIAN_POINT ( 'NONE',  ( 358.0000000000000000, 165.0000000000000000, -106.0000000000001990 ) ) ;
#19473=CARTESIAN_POINT ( 'NONE',  ( 342.0000000000000568, 181.0000000000000284, 355.9999999999998863 ) ) ;
#19479=VERTEX_POINT ( 'NONE', #6861 ) ;
#19480=DIRECTION ( 'NONE',  ( 0.000000000000000000, 0.000000000000000000, 1.000000000000000000 ) ) ;
#19487=ORIENTED_EDGE ( 'NONE', *, *, #29564, .F. ) ;
#19488=DIRECTION ( 'NONE',  ( -0.000000000000000000, -1.000000000000000000, 2.537652627714643577E-15 ) ) ;
#19492=DIRECTION ( 'NONE',  ( 1.000000000000000000, -4.996003610813203446E-16, -1.586032878436834529E-16 ) ) ;
#19495=CARTESIAN_POINT ( 'NONE',  ( 339.9999999999999432, -180.9999999999999716, -360.0000000000002274 ) ) ;
#19496=DIRECTION ( 'NONE',  ( 0.000000000000000000, 0.000000000000000000, -1.000000000000000000 ) ) ;
#19502=DIRECTION ( 'NONE',  ( -1.586032892321652236E-16, -1.000000000000000000, -6.853681917100419162E-49 ) ) ;
#19506=CYLINDRICAL_SURFACE ( 'NONE', #3792, 4.000000000000003553 ) ;
#19512=CARTESIAN_POINT ( 'NONE',  ( 168.9999999999999716, -254.4999999999999432, -349.9999999999999432 ) ) ;
#19521=AXIS2_PLACEMENT_3D ( 'NONE', #40937, #44763, #9636 ) ;
#19523=CARTESIAN_POINT ( 'NONE',  ( 181.0000000000000284, -174.9999999999999716, -111.0000000000001563 ) ) ;
#19525=ORIENTED_EDGE ( 'NONE', *, *, #7368, .T. ) ;
#19529=CARTESIAN_POINT ( 'NONE',  ( 360.0000000000000568, -3.000000000000196732, -178.0000000000003695 ) ) ;
#19532=EDGE_CURVE ( 'NONE', #1115, #2541, #22503, .T. ) ;
#19540=EDGE_CURVE ( 'NONE', #39358, #9482, #21749, .T. ) ;
#19549=DIRECTION ( 'NONE',  ( 1.000000000000000000, 0.000000000000000000, 0.000000000000000000 ) ) ;
#19552=LINE ( 'NONE', #8536, #46314 ) ;
#19553=EDGE_CURVE ( 'NONE', #27291, #29017, #34062, .T. ) ;
#19554=EDGE_LOOP ( 'NONE', ( #46167, #29308, #6269, #16020, #4679, #27110, #13302, #42985 ) ) ;
#19555=EDGE_LOOP ( 'NONE', ( #44805, #10520, #38653, #34956 ) ) ;
#19558=CIRCLE ( 'NONE', #2388, 2.000000000000001776 ) ;
#19563=VERTEX_POINT ( 'NONE', #46830 ) ;
#19564=DIRECTION ( 'NONE',  ( 1.000000000000000000, 0.000000000000000000, -4.758098676964956461E-16 ) ) ;
#19566=VECTOR ( 'NONE', #21031, 1000.000000000000000 ) ;
#19588=EDGE_CURVE ( 'NONE', #28405, #20395, #15331, .T. ) ;
#19591=( LENGTH_UNIT ( ) NAMED_UNIT ( * ) SI_UNIT ( .MILLI., .METRE. ) );
#19592=CARTESIAN_POINT ( 'NONE',  ( 0.000000000000000000, -166.9999999999999432, -356.0000000000002274 ) ) ;
#19594=DIRECTION ( 'NONE',  ( 0.000000000000000000, -1.000000000000000000, -1.544785076050074834E-48 ) ) ;
#19603=AXIS2_PLACEMENT_3D ( 'NONE', #21371, #25228, #5723 ) ;
#19608=ORIENTED_EDGE ( 'NONE', *, *, #5796, .T. ) ;
#19624=DIRECTION ( 'NONE',  ( -0.000000000000000000, -1.000000000000000000, -0.000000000000000000 ) ) ;
#19627=ORIENTED_EDGE ( 'NONE', *, *, #17143, .F. ) ;
#19628=ORIENTED_EDGE ( 'NONE', *, *, #15825, .T. ) ;
#19631=LINE ( 'NONE', #34804, #24282 ) ;
#19632=DIRECTION ( 'NONE',  ( 1.000000000000000000, 0.000000000000000000, 0.000000000000000000 ) ) ;
#19638=VECTOR ( 'NONE', #3319, 1000.000000000000000 ) ;
#19644=CARTESIAN_POINT ( 'NONE',  ( 357.1715728752542418, 167.0000000000003695, 342.0000000000001137 ) ) ;
#19648=DIRECTION ( 'NONE',  ( -1.000000000000000000, 1.586032892321652236E-16, 9.711650524620651178E-33 ) ) ;
#19662=ORIENTED_EDGE ( 'NONE', *, *, #48614, .T. ) ;
#19663=EDGE_CURVE ( 'NONE', #38030, #24255, #24042, .T. ) ;
#19671=VECTOR ( 'NONE', #964, 1000.000000000000000 ) ;
#19675=CARTESIAN_POINT ( 'NONE',  ( 168.9999999999999716, -164.9999999999999432, -350.0000000000001705 ) ) ;
#19686=ADVANCED_FACE ( 'NONE', ( #27889 ), #44017, .T. ) ;
#19696=ORIENTED_EDGE ( 'NONE', *, *, #18623, .F. ) ;
#19697=DIRECTION ( 'NONE',  ( -0.000000000000000000, 1.544785076050074834E-48, 1.000000000000000000 ) ) ;
#19701=EDGE_LOOP ( 'NONE', ( #22416, #32916, #17857, #14158 ) ) ;
#19702=DIRECTION ( 'NONE',  ( 0.000000000000000000, 0.000000000000000000, -1.000000000000000000 ) ) ;
#19704=CARTESIAN_POINT ( 'NONE',  ( 181.0000000000000000, -9.999999999999953815, -350.0000000000001705 ) ) ;
#19710=VERTEX_POINT ( 'NONE', #44288 ) ;
#19713=EDGE_LOOP ( 'NONE', ( #47794, #9448, #39168, #33139, #21977, #8847, #19824, #41835 ) ) ;
#19714=AXIS2_PLACEMENT_3D ( 'NONE', #31256, #11743, #38448 ) ;
#19723=( LENGTH_UNIT ( ) NAMED_UNIT ( * ) SI_UNIT ( .MILLI., .METRE. ) );
#19729=CYLINDRICAL_SURFACE ( 'NONE', #18333, 2.000000000000001776 ) ;
#19735=( BOUNDED_CURVE ( )  B_SPLINE_CURVE ( 3, ( #1210, #5293, #16595, #20950 ),
 .UNSPECIFIED., .F., .F. ) 
 B_SPLINE_CURVE_WITH_KNOTS ( ( 4, 4 ),
 ( 3.141592653589793116, 4.712388980384710990 ),
 .UNSPECIFIED. ) 
 CURVE ( )  GEOMETRIC_REPRESENTATION_ITEM ( )  RATIONAL_B_SPLINE_CURVE ( ( 1.000000000000000000, 0.8047378541243599415, 0.8047378541243599415, 1.000000000000000000 ) ) 
 REPRESENTATION_ITEM ( '' )  );
#19739=EDGE_LOOP ( 'NONE', ( #27029, #34649 ) ) ;
#19748=FACE_OUTER_BOUND ( 'NONE', #2889, .T. ) ;
#19750=AXIS2_PLACEMENT_3D ( 'NONE', #7075, #43227, #27599 ) ;
#19751=EDGE_CURVE ( 'NONE', #4003, #41575, #24566, .T. ) ;
#19759=LINE ( 'NONE', #36710, #38029 ) ;
#19760=VERTEX_POINT ( 'NONE', #43799 ) ;
#19761=VECTOR ( 'NONE', #15763, 1000.000000000000000 ) ;
#19762=LINE ( 'NONE', #50505, #27563 ) ;
#19763=CARTESIAN_POINT ( 'NONE',  ( 164.9999999999999716, 175.0000000000000284, -344.0000000000001137 ) ) ;
#19765=DIRECTION ( 'NONE',  ( -1.586032892321652236E-16, -1.000000000000000000, -6.853681917100419162E-49 ) ) ;
#19773=LINE ( 'NONE', #4641, #32814 ) ;
#19795=EDGE_LOOP ( 'NONE', ( #21878, #26011, #12447, #330 ) ) ;
#19799=ORIENTED_EDGE ( 'NONE', *, *, #7305, .F. ) ;
#19801=DIRECTION ( 'NONE',  ( 4.758098676964956461E-16, 1.000000000000000000, 0.000000000000000000 ) ) ;
#19805=CARTESIAN_POINT ( 'NONE',  ( 181.0000000000000000, -79.49999999999997158, -350.0000000000001705 ) ) ;
#19806=LINE ( 'NONE', #35751, #46701 ) ;
#19814=ORIENTED_EDGE ( 'NONE', *, *, #42831, .T. ) ;
#19818=VECTOR ( 'NONE', #13410, 1000.000000000000000 ) ;
#19820=FACE_OUTER_BOUND ( 'NONE', #42707, .T. ) ;
#19824=ORIENTED_EDGE ( 'NONE', *, *, #47426, .F. ) ;
#19825=DIRECTION ( 'NONE',  ( 6.203854594147707562E-25, -2.067951531382569187E-25, 1.000000000000000000 ) ) ;
#19830=ORIENTED_EDGE ( 'NONE', *, *, #32109, .T. ) ;
#19831=VERTEX_POINT ( 'NONE', #20970 ) ;
#19835=VERTEX_POINT ( 'NONE', #36654 ) ;
#19836=CARTESIAN_POINT ( 'NONE',  ( 183.0000000000000000, -184.9999999999999716, -356.0000000000014211 ) ) ;
#19838=VERTEX_POINT ( 'NONE', #4313 ) ;
#19841=LINE ( 'NONE', #3687, #50377 ) ;
#19843=CARTESIAN_POINT ( 'NONE',  ( 168.9999999999999716, 6.000000000000060396, 339.9999999999998295 ) ) ;
#19844=LINE ( 'NONE', #20607, #44849 ) ;
#19846=PLANE ( 'NONE',  #20054 ) ;
#19847=CARTESIAN_POINT ( 'NONE',  ( 0.000000000000000000, -175.0000000000000284, 353.7500000000001705 ) ) ;
#19851=AXIS2_PLACEMENT_3D ( 'NONE', #10619, #26033, #5326 ) ;
#19854=AXIS2_PLACEMENT_3D ( 'NONE', #25539, #41179, #6029 ) ;
#19856=CIRCLE ( 'NONE', #48492, 2.000000000000001776 ) ;
#19864=EDGE_CURVE ( 'NONE', #38973, #26951, #28421, .T. ) ;
#19866=CARTESIAN_POINT ( 'NONE',  ( 164.9999999999999716, -164.9999999999999432, -344.0000000000001137 ) ) ;
#19867=LINE ( 'NONE', #28584, #9460 ) ;
#19870=AXIS2_PLACEMENT_3D ( 'NONE', #46475, #3148, #22915 ) ;
#19871=VERTEX_POINT ( 'NONE', #16358 ) ;
#19873=DIRECTION ( 'NONE',  ( -0.000000000000000000, -1.000000000000000000, -0.000000000000000000 ) ) ;
#19874=EDGE_CURVE ( 'NONE', #43828, #25523, #1316, .T. ) ;
#19882=( GEOMETRIC_REPRESENTATION_CONTEXT ( 3 ) GLOBAL_UNCERTAINTY_ASSIGNED_CONTEXT ( ( #20482 ) ) GLOBAL_UNIT_ASSIGNED_CONTEXT ( ( #6522, #18567, #45993 ) ) REPRESENTATION_CONTEXT ( 'NONE', 'WORKASPACE' ) );
#19893=ORIENTED_EDGE ( 'NONE', *, *, #11144, .T. ) ;
#19896=VERTEX_POINT ( 'NONE', #48870 ) ;
#19897=ADVANCED_FACE ( 'NONE', ( #1722 ), #2469, .F. ) ;
#19904=DIRECTION ( 'NONE',  ( -1.000000000000000000, 0.000000000000000000, 0.000000000000000000 ) ) ;
#19908=ORIENTED_EDGE ( 'NONE', *, *, #36838, .T. ) ;
#19910=DIRECTION ( 'NONE',  ( 0.000000000000000000, -1.000000000000000000, -3.186989995019654210E-49 ) ) ;
#19917=AXIS2_PLACEMENT_3D ( 'NONE', #11399, #47957, #23197 ) ;
#19922=VERTEX_POINT ( 'NONE', #9664 ) ;
#19924=EDGE_CURVE ( 'NONE', #16572, #13422, #5816, .T. ) ;
#19937=DIRECTION ( 'NONE',  ( 0.000000000000000000, 0.000000000000000000, 1.000000000000000000 ) ) ;
#19942=LINE ( 'NONE', #45221, #29233 ) ;
#19947=VERTEX_POINT ( 'NONE', #34810 ) ;
#19952=EDGE_CURVE ( 'NONE', #2948, #49297, #23226, .T. ) ;
#19953=ORIENTED_EDGE ( 'NONE', *, *, #20891, .T. ) ;
#19956=VECTOR ( 'NONE', #18641, 1000.000000000000000 ) ;
#19958=EDGE_LOOP ( 'NONE', ( #41749, #21724, #33703, #48790 ) ) ;
#19959=CIRCLE ( 'NONE', #33098, 4.000000000000003553 ) ;
#19965=DIRECTION ( 'NONE',  ( 3.172065745548403743E-16, 1.000000000000000000, 0.000000000000000000 ) ) ;
#19966=CARTESIAN_POINT ( 'NONE',  ( 185.0000000000000000, 165.0000000000000000, -356.0000000000001705 ) ) ;
#19972=ADVANCED_FACE ( 'NONE', ( #38397 ), #46542, .F. ) ;
#19975=EDGE_CURVE ( 'NONE', #49105, #10936, #23502, .T. ) ;
#19983=DIRECTION ( 'NONE',  ( 0.000000000000000000, -1.000000000000000000, 0.000000000000000000 ) ) ;
#19990=ORIENTED_EDGE ( 'NONE', *, *, #15158, .T. ) ;
#20009=CYLINDRICAL_SURFACE ( 'NONE', #34782, 4.000000000000003553 ) ;
#20011=EDGE_CURVE ( 'NONE', #20258, #2953, #42714, .T. ) ;
#20016=DIRECTION ( 'NONE',  ( 1.000000000000000000, 0.000000000000000000, 0.000000000000000000 ) ) ;
#20023=CARTESIAN_POINT ( 'NONE',  ( 183.0000000000000000, 165.0000000000000000, -356.0000000000001705 ) ) ;
#20024=DIRECTION ( 'NONE',  ( 0.000000000000000000, 0.000000000000000000, -1.000000000000000000 ) ) ;
#20026=DIRECTION ( 'NONE',  ( -1.000000000000000000, 0.000000000000000000, 1.860490536778032451E-50 ) ) ;
#20029=VERTEX_POINT ( 'NONE', #49860 ) ;
#20031=CARTESIAN_POINT ( 'NONE',  ( 0.000000000000000000, 183.0000000000000284, -344.0000000000001705 ) ) ;
#20033=CIRCLE ( 'NONE', #46176, 4.000000000000003553 ) ;
#20042=EDGE_CURVE ( 'NONE', #15072, #49733, #15299, .T. ) ;
#20053=ORIENTED_EDGE ( 'NONE', *, *, #44960, .T. ) ;
#20054=AXIS2_PLACEMENT_3D ( 'NONE', #7817, #19081, #11913 ) ;
#20056=ORIENTED_EDGE ( 'NONE', *, *, #10149, .T. ) ;
#20061=DIRECTION ( 'NONE',  ( -1.000000000000000000, 0.000000000000000000, 0.000000000000000000 ) ) ;
#20068=AXIS2_PLACEMENT_3D ( 'NONE', #2960, #33786, #38149 ) ;
#20077=ORIENTED_EDGE ( 'NONE', *, *, #19663, .F. ) ;
#20083=ORIENTED_EDGE ( 'NONE', *, *, #24045, .T. ) ;
#20085=DIRECTION ( 'NONE',  ( 1.132880637372608740E-16, 4.718402560806925739E-50, 1.000000000000000000 ) ) ;
#20086=AXIS2_PLACEMENT_3D ( 'NONE', #9400, #40955, #44776 ) ;
#20089=EDGE_LOOP ( 'NONE', ( #36106, #47571, #3995, #27071 ) ) ;
#20094=PRODUCT_DEFINITION_CONTEXT ( 'detailed design', #30246, 'design' ) ;
#20095=ORIENTED_EDGE ( 'NONE', *, *, #44628, .T. ) ;
#20097=ORIENTED_EDGE ( 'NONE', *, *, #31784, .T. ) ;
#20100=AXIS2_PLACEMENT_3D ( 'NONE', #17519, #29827, #33191 ) ;
#20101=DIRECTION ( 'NONE',  ( 1.000000000000000000, 0.000000000000000000, -1.612977847700450206E-50 ) ) ;
#20106=AXIS2_PLACEMENT_3D ( 'NONE', #46375, #49700, #2787 ) ;
#20109=EDGE_CURVE ( 'NONE', #26847, #44300, #5252, .T. ) ;
#20115=( BOUNDED_CURVE ( )  B_SPLINE_CURVE ( 3, ( #17854, #33521, #22219, #26574 ),
 .UNSPECIFIED., .F., .F. ) 
 B_SPLINE_CURVE_WITH_KNOTS ( ( 4, 4 ),
 ( 4.712388980384710990, 6.283185307179309120 ),
 .UNSPECIFIED. ) 
 CURVE ( )  GEOMETRIC_REPRESENTATION_ITEM ( )  RATIONAL_B_SPLINE_CURVE ( ( 1.000000000000000000, 0.8047378541243699335, 0.8047378541243699335, 1.000000000000000000 ) ) 
 REPRESENTATION_ITEM ( '' )  );
#20116=CARTESIAN_POINT ( 'NONE',  ( 356.0000000000000000, 174.9999999999996589, -344.0000000000002842 ) ) ;
#20120=ORIENTED_EDGE ( 'NONE', *, *, #50609, .F. ) ;
#20123=VECTOR ( 'NONE', #8420, 1000.000000000000000 ) ;
#20125=CARTESIAN_POINT ( 'NONE',  ( 0.000000000000000000, 181.0000000000000284, 359.9999999999997726 ) ) ;
#20131=AXIS2_PLACEMENT_3D ( 'NONE', #7146, #10990, #23287 ) ;
#20133=ORIENTED_EDGE ( 'NONE', *, *, #45592, .T. ) ;
#20144=AXIS2_PLACEMENT_3D ( 'NONE', #47796, #32457, #43973 ) ;
#20150=FACE_OUTER_BOUND ( 'NONE', #38593, .T. ) ;
#20152=DIRECTION ( 'NONE',  ( -4.758098676964956461E-16, -1.000000000000000000, 0.000000000000000000 ) ) ;
#20154=ORIENTED_EDGE ( 'NONE', *, *, #6024, .F. ) ;
#20159=CARTESIAN_POINT ( 'NONE',  ( 339.9999999999998863, -180.9999999999999716, 355.9999999999997726 ) ) ;
#20160=CARTESIAN_POINT ( 'NONE',  ( -5.000000000000000000, 175.0000000000000284, 353.7500000000001705 ) ) ;
#20161=CARTESIAN_POINT ( 'NONE',  ( 185.0000000000000284, -174.9999999999999716, -111.0000000000001563 ) ) ;
#20164=ORIENTED_EDGE ( 'NONE', *, *, #34914, .F. ) ;
#20173=STYLED_ITEM('',(#50747),#22072);
#20183=LINE ( 'NONE', #24306, #14163 ) ;
#20195=PLANE ( 'NONE',  #36591 ) ;
#20197=EDGE_CURVE ( 'NONE', #24185, #31089, #20978, .T. ) ;
#20199=AXIS2_PLACEMENT_3D ( 'NONE', #31132, #38079, #50572 ) ;
#20203=VECTOR ( 'NONE', #33239, 1000.000000000000000 ) ;
#20216=ORIENTED_EDGE ( 'NONE', *, *, #48614, .F. ) ;
#20217=VERTEX_POINT ( 'NONE', #21402 ) ;
#20218=LINE ( 'NONE', #25085, #24598 ) ;
#20219=CARTESIAN_POINT ( 'NONE',  ( 5.551115123125782702E-14, -168.9999999999999432, 355.9999999999997726 ) ) ;
#20222=CIRCLE ( 'NONE', #9564, 2.000000000000001776 ) ;
#20223=DIRECTION ( 'NONE',  ( 1.000000000000000000, -4.758098676964956461E-16, -8.975803739141899931E-48 ) ) ;
#20224=CARTESIAN_POINT ( 'NONE',  ( 183.0000000000000000, 175.0000000000000284, -356.0000000000001705 ) ) ;
#20228=CARTESIAN_POINT ( 'NONE',  ( 167.0000000000000000, -180.9999999999999716, -115.0000000000001563 ) ) ;
#20238=VECTOR ( 'NONE', #25078, 1000.000000000000000 ) ;
#20241=CARTESIAN_POINT ( 'NONE',  ( 350.0000000000001137, 169.0000000000000000, 341.9999999999997726 ) ) ;
#20258=VERTEX_POINT ( 'NONE', #1917 ) ;
#20259=EDGE_CURVE ( 'NONE', #1207, #20650, #40650, .T. ) ;
#20261=ORIENTED_EDGE ( 'NONE', *, *, #11230, .T. ) ;
#20268=CARTESIAN_POINT ( 'NONE',  ( 181.0000000000000000, 10.00000000000006395, -340.0000000000001137 ) ) ;
#20273=FACE_OUTER_BOUND ( 'NONE', #18879, .T. ) ;
#20276=LINE ( 'NONE', #40784, #16914 ) ;
#20288=FACE_OUTER_BOUND ( 'NONE', #39606, .T. ) ;
#20290=EDGE_LOOP ( 'NONE', ( #22304, #340, #12655, #17815 ) ) ;
#20293=DIRECTION ( 'NONE',  ( -1.586032892321651989E-16, -1.194346094642793337E-32, -1.000000000000000000 ) ) ;
#20294=PLANE ( 'NONE',  #33265 ) ;
#20296=CARTESIAN_POINT ( 'NONE',  ( -5.000000000000000000, 165.2000000000000171, -340.2000000000001592 ) ) ;
#20300=ADVANCED_FACE ( 'NONE', ( #40913 ), #5752, .T. ) ;
#20308=ORIENTED_EDGE ( 'NONE', *, *, #12660, .F. ) ;
#20311=CARTESIAN_POINT ( 'NONE',  ( 183.0000000000000000, -272.5000000000000000, -111.0000000000001563 ) ) ;
#20315=EDGE_CURVE ( 'NONE', #4748, #19163, #11374, .T. ) ;
#20318=DIRECTION ( 'NONE',  ( 1.000000000000000000, 0.000000000000000000, -1.860490536778032451E-50 ) ) ;
#20323=DIRECTION ( 'NONE',  ( 0.000000000000000000, 0.000000000000000000, 1.000000000000000000 ) ) ;
#20325=ORIENTED_EDGE ( 'NONE', *, *, #4090, .F. ) ;
#20326=EDGE_CURVE ( 'NONE', #7888, #2228, #30120, .T. ) ;
#20328=DIRECTION ( 'NONE',  ( 0.000000000000000000, 0.000000000000000000, -1.000000000000000000 ) ) ;
#20333=CARTESIAN_POINT ( 'NONE',  ( 168.9999999999999716, 174.9999999999999716, -340.0000000000001137 ) ) ;
#20334=CARTESIAN_POINT ( 'NONE',  ( 358.0000000000001137, -172.0000000000000000, -3.000000000000058176 ) ) ;
#20335=ORIENTED_EDGE ( 'NONE', *, *, #26868, .F. ) ;
#20342=VERTEX_POINT ( 'NONE', #7274 ) ;
#20346=LINE ( 'NONE', #43680, #38016 ) ;
#20348=CARTESIAN_POINT ( 'NONE',  ( 341.9999999999999432, 169.0000000000001990, -344.0000000000002842 ) ) ;
#20350=CARTESIAN_POINT ( 'NONE',  ( 349.9999999999999432, -168.9999999999999432, 341.9999999999997726 ) ) ;
#20351=ORIENTED_EDGE ( 'NONE', *, *, #22554, .F. ) ;
#20357=CYLINDRICAL_SURFACE ( 'NONE', #18231, 2.000000000000001776 ) ;
#20359=CARTESIAN_POINT ( 'NONE',  ( 169.0000000000000000, -9.999999999999953815, -111.0000000000001563 ) ) ;
#20362=CARTESIAN_POINT ( 'NONE',  ( 181.0000000000000000, -184.9999999999999716, -360.0000000000002274 ) ) ;
#20365=DIRECTION ( 'NONE',  ( 0.000000000000000000, 0.000000000000000000, -1.000000000000000000 ) ) ;
#20373=FACE_OUTER_BOUND ( 'NONE', #37560, .T. ) ;
#20375=CARTESIAN_POINT ( 'NONE',  ( 349.9999999999999432, -166.9999999999999432, 355.9999999999997726 ) ) ;
#20376=EDGE_LOOP ( 'NONE', ( #4922, #16972, #42634, #48101 ) ) ;
#20377=CLOSED_SHELL ( 'NONE', ( #17944, #35882, #32436, #35967, #44810, #22464, #50412, #26867, #21523, #29678, #34710, #39208, #43489, #33847, #15347, #14532, #39011, #17527 ) ) ;
#20394=ORIENTED_EDGE ( 'NONE', *, *, #7473, .F. ) ;
#20395=VERTEX_POINT ( 'NONE', #50579 ) ;
#20396=CYLINDRICAL_SURFACE ( 'NONE', #40198, 2.000000000000001776 ) ;
#20402=CARTESIAN_POINT ( 'NONE',  ( 339.9999999999998863, -168.9999999999999432, 339.9999999999997726 ) ) ;
#20410=CARTESIAN_POINT ( 'NONE',  ( 169.0000000000000000, -9.999999999999953815, -95.00000000000014211 ) ) ;
#20413=VECTOR ( 'NONE', #18176, 1000.000000000000000 ) ;
#20415=CARTESIAN_POINT ( 'NONE',  ( 355.9999999999999432, 174.9999999999996305, -360.0000000000003411 ) ) ;
#20419=VECTOR ( 'NONE', #3519, 1000.000000000000000 ) ;
#20425=DIRECTION ( 'NONE',  ( 0.000000000000000000, 0.000000000000000000, -1.000000000000000000 ) ) ;
#20431=LINE ( 'NONE', #43022, #24919 ) ;
#20432=EDGE_LOOP ( 'NONE', ( #46910, #21450, #23095, #18022 ) ) ;
#20434=ORIENTED_EDGE ( 'NONE', *, *, #13798, .T. ) ;
#20435=CARTESIAN_POINT ( 'NONE',  ( -5.000000000000000000, -184.7999999999999545, -340.2000000000001592 ) ) ;
#20436=CARTESIAN_POINT ( 'NONE',  ( 183.0000000000000284, -9.999999999999953815, -99.00000000000014211 ) ) ;
#20437=CIRCLE ( 'NONE', #27000, 2.000000000000001776 ) ;
#20438=VECTOR ( 'NONE', #14683, 1000.000000000000000 ) ;
#20441=DIRECTION ( 'NONE',  ( 0.000000000000000000, -2.265761274745217480E-16, 1.000000000000000000 ) ) ;
#20455=ORIENTED_EDGE ( 'NONE', *, *, #304, .T. ) ;
#20460=CARTESIAN_POINT ( 'NONE',  ( 356.0000000000000568, 183.0000000000000853, 357.9999999999998295 ) ) ;
#20461=ORIENTED_EDGE ( 'NONE', *, *, #32308, .F. ) ;
#20468=DIRECTION ( 'NONE',  ( 3.364279341222521245E-16, 0.7071067811865474617, -0.7071067811865475727 ) ) ;
#20470=CARTESIAN_POINT ( 'NONE',  ( 181.0000000000000000, -166.9999999999999432, -340.0000000000001137 ) ) ;
#20472=DIRECTION ( 'NONE',  ( 0.000000000000000000, 1.000000000000000000, 6.123233995736766036E-17 ) ) ;
#20477=ADVANCED_FACE ( 'NONE', ( #605 ), #47501, .T. ) ;
#20482=UNCERTAINTY_MEASURE_WITH_UNIT (LENGTH_MEASURE( 1.000000000000000082E-05 ), #6522, 'distance_accuracy_value', 'NONE');
#20491=DIRECTION ( 'NONE',  ( 1.000000000000000000, 0.000000000000000000, -0.000000000000000000 ) ) ;
#20492=VECTOR ( 'NONE', #6191, 1000.000000000000000 ) ;
#20493=ORIENTED_EDGE ( 'NONE', *, *, #39821, .T. ) ;
#20494=DIRECTION ( 'NONE',  ( 1.000000000000000000, 0.000000000000000000, 0.000000000000000000 ) ) ;
#20495=FACE_OUTER_BOUND ( 'NONE', #24272, .T. ) ;
#20499=CARTESIAN_POINT ( 'NONE',  ( 343.9999999999999432, 174.9999999999996589, -356.0000000000003411 ) ) ;
#20509=LINE ( 'NONE', #36704, #31109 ) ;
#20513=CARTESIAN_POINT ( 'NONE',  ( 342.8284271247462129, 167.0000000000000000, 341.9999999999998295 ) ) ;
#20515=CARTESIAN_POINT ( 'NONE',  ( 183.0000000000000000, -180.9999999999999432, -340.0000000000001137 ) ) ;
#20518=ADVANCED_FACE ( 'NONE', ( #16497 ), #36014, .T. ) ;
#20520=AXIS2_PLACEMENT_3D ( 'NONE', #5232, #20882, #8086 ) ;
#20521=VECTOR ( 'NONE', #50490, 1000.000000000000000 ) ;
#20527=CIRCLE ( 'NONE', #29429, 4.000000000000003553 ) ;
#20531=ORIENTED_EDGE ( 'NONE', *, *, #18991, .T. ) ;
#20535=FACE_OUTER_BOUND ( 'NONE', #33654, .T. ) ;
#20547=EDGE_CURVE ( 'NONE', #4003, #44732, #39353, .T. ) ;
#20569=ORIENTED_EDGE ( 'NONE', *, *, #14902, .T. ) ;
#20579=FACE_OUTER_BOUND ( 'NONE', #41599, .T. ) ;
#20585=CARTESIAN_POINT ( 'NONE',  ( 166.9999999999999716, -5.999999999999950262, -340.0000000000001137 ) ) ;
#20589=VECTOR ( 'NONE', #42670, 1000.000000000000000 ) ;
#20590=DIRECTION ( 'NONE',  ( 0.000000000000000000, 0.000000000000000000, 1.000000000000000000 ) ) ;
#20600=CARTESIAN_POINT ( 'NONE',  ( 350.0000000000000000, 181.0000000000000284, -344.0000000000001705 ) ) ;
#20607=CARTESIAN_POINT ( 'NONE',  ( 350.0000000000000000, 181.0000000000000284, -360.0000000000002274 ) ) ;
#20618=CARTESIAN_POINT ( 'NONE',  ( 166.9999999999999716, -164.9999999999999432, 355.9999999999998863 ) ) ;
#20624=CARTESIAN_POINT ( 'NONE',  ( 360.0000000000000000, 169.0000000000001990, -344.0000000000002842 ) ) ;
#20626=DIRECTION ( 'NONE',  ( 3.364279341222521245E-16, 0.7071067811865474617, -0.7071067811865476838 ) ) ;
#20629=CIRCLE ( 'NONE', #49249, 4.000000000000003553 ) ;
#20630=ADVANCED_FACE ( 'NONE', ( #48754 ), #40605, .F. ) ;
#20631=CARTESIAN_POINT ( 'NONE',  ( 0.000000000000000000, -168.9999999999999432, -360.0000000000002274 ) ) ;
#20632=VERTEX_POINT ( 'NONE', #17990 ) ;
#20635=CARTESIAN_POINT ( 'NONE',  ( 358.3431457505075741, -165.0000000000001137, -340.0000000000002274 ) ) ;
#20647=CARTESIAN_POINT ( 'NONE',  ( 181.0000000000000000, -272.5000000000000000, -110.9999999999999005 ) ) ;
#20649=ORIENTED_EDGE ( 'NONE', *, *, #36630, .F. ) ;
#20650=VERTEX_POINT ( 'NONE', #44911 ) ;
#20660=VERTEX_POINT ( 'NONE', #3609 ) ;
#20667=CARTESIAN_POINT ( 'NONE',  ( 350.0000000000000000, -164.9999999999999432, -356.0000000000002274 ) ) ;
#20670=CIRCLE ( 'NONE', #36256, 2.000000000000001776 ) ;
#20673=VERTEX_POINT ( 'NONE', #42095 ) ;
#20689=VECTOR ( 'NONE', #48575, 1000.000000000000000 ) ;
#20695=CARTESIAN_POINT ( 'NONE',  ( 183.0000000000000000, -180.9999999999999716, -340.0000000000001137 ) ) ;
#20702=VECTOR ( 'NONE', #9072, 1000.000000000000000 ) ;
#20707=DIRECTION ( 'NONE',  ( 6.203854594147707562E-25, -2.067951531382569187E-25, 1.000000000000000000 ) ) ;
#20714=LINE ( 'NONE', #36391, #20238 ) ;
#20720=AXIS2_PLACEMENT_3D ( 'NONE', #849, #16992, #46985 ) ;
#20722=ORIENTED_EDGE ( 'NONE', *, *, #10976, .F. ) ;
#20726=LINE ( 'NONE', #16890, #5508 ) ;
#20730=CARTESIAN_POINT ( 'NONE',  ( 181.0000000000000284, 2.775557561562891351E-14, -111.0000000000001563 ) ) ;
#20734=VECTOR ( 'NONE', #24048, 1000.000000000000000 ) ;
#20739=ADVANCED_FACE ( 'NONE', ( #30570 ), #2590, .T. ) ;
#20740=CARTESIAN_POINT ( 'NONE',  ( 344.0000000000000000, 185.0000000000000000, 359.9999999999998295 ) ) ;
#20741=PLANE ( 'NONE',  #4043 ) ;
#20746=CARTESIAN_POINT ( 'NONE',  ( 181.0000000000000000, -164.9999999999999432, -358.0000000000001705 ) ) ;
#20749=FACE_OUTER_BOUND ( 'NONE', #18814, .T. ) ;
#20752=( NAMED_UNIT ( * ) SI_UNIT ( $, .STERADIAN. ) SOLID_ANGLE_UNIT ( ) );
#20755=ORIENTED_EDGE ( 'NONE', *, *, #8346, .T. ) ;
#20756=CARTESIAN_POINT ( 'NONE',  ( 343.9999999999999432, 185.0000000000002558, -360.0000000000003411 ) ) ;
#20759=ORIENTED_EDGE ( 'NONE', *, *, #24297, .F. ) ;
#20762=CIRCLE ( 'NONE', #13361, 4.000000000000003553 ) ;
#20763=DIRECTION ( 'NONE',  ( 1.612977847700450206E-50, 0.000000000000000000, 1.000000000000000000 ) ) ;
#20766=CARTESIAN_POINT ( 'NONE',  ( -5.000000000000000000, -165.1999999999999602, 359.7999999999997840 ) ) ;
#20768=AXIS2_PLACEMENT_3D ( 'NONE', #37559, #2378, #30095 ) ;
#20770=LINE ( 'NONE', #16942, #8131 ) ;
#20771=VERTEX_POINT ( 'NONE', #10311 ) ;
#20773=LINE ( 'NONE', #32598, #29503 ) ;
#20774=( BOUNDED_CURVE ( )  B_SPLINE_CURVE ( 3, ( #43568, #28187, #36669, #8435 ),
 .UNSPECIFIED., .F., .F. ) 
 B_SPLINE_CURVE_WITH_KNOTS ( ( 4, 4 ),
 ( 1.570796326794882791, 3.141592653589793116 ),
 .UNSPECIFIED. ) 
 CURVE ( )  GEOMETRIC_REPRESENTATION_ITEM ( )  RATIONAL_B_SPLINE_CURVE ( ( 1.000000000000000000, 0.8047378541243617178, 0.8047378541243617178, 1.000000000000000000 ) ) 
 REPRESENTATION_ITEM ( '' )  );
#20780=CARTESIAN_POINT ( 'NONE',  ( 181.0000000000000000, -256.4999999999999432, -339.9999999999998863 ) ) ;
#20790=DIRECTION ( 'NONE',  ( 0.000000000000000000, 0.000000000000000000, 1.000000000000000000 ) ) ;
#20792=VECTOR ( 'NONE', #15912, 1000.000000000000000 ) ;
#20794=LINE ( 'NONE', #36475, #47765 ) ;
#20796=CARTESIAN_POINT ( 'NONE',  ( 181.0000000000000000, 10.00000000000006395, -350.0000000000001705 ) ) ;
#20800=VECTOR ( 'NONE', #15343, 1000.000000000000000 ) ;
#20803=EDGE_CURVE ( 'NONE', #17104, #7818, #22616, .T. ) ;
#20814=EDGE_LOOP ( 'NONE', ( #7974, #14165, #4608, #16589 ) ) ;
#20821=FACE_OUTER_BOUND ( 'NONE', #11623, .T. ) ;
#20823=EDGE_LOOP ( 'NONE', ( #21714, #1808, #32843, #41081 ) ) ;
#20824=ADVANCED_FACE ( 'NONE', ( #39285 ), #11576, .T. ) ;
#20826=DIRECTION ( 'NONE',  ( 0.000000000000000000, -1.000000000000000000, 0.000000000000000000 ) ) ;
#20838=AXIS2_PLACEMENT_3D ( 'NONE', #35921, #34913, #39262 ) ;
#20840=CARTESIAN_POINT ( 'NONE',  ( 341.6568542494924259, 164.9999999999999716, 339.9999999999998295 ) ) ;
#20844=CYLINDRICAL_SURFACE ( 'NONE', #33172, 2.000000000000001776 ) ;
#20847=ORIENTED_EDGE ( 'NONE', *, *, #46939, .F. ) ;
#20849=CARTESIAN_POINT ( 'NONE',  ( -5.000000000000000000, -175.0000000000000284, 350.0000000000002274 ) ) ;
#20852=ORIENTED_EDGE ( 'NONE', *, *, #46631, .T. ) ;
#20859=CIRCLE ( 'NONE', #5327, 4.000000000000003553 ) ;
#20860=ADVANCED_FACE ( 'NONE', ( #24147 ), #19506, .T. ) ;
#20861=EDGE_CURVE ( 'NONE', #14457, #49709, #39797, .T. ) ;
#20872=CARTESIAN_POINT ( 'NONE',  ( -5.000000000000000000, -165.1999999999999602, 359.7999999999997840 ) ) ;
#20875=DIRECTION ( 'NONE',  ( -0.000000000000000000, 1.000000000000000000, 0.000000000000000000 ) ) ;
#20882=DIRECTION ( 'NONE',  ( 0.000000000000000000, 2.537652627714642000E-15, 1.000000000000000000 ) ) ;
#20891=EDGE_CURVE ( 'NONE', #22581, #46920, #40047, .T. ) ;
#20894=EDGE_LOOP ( 'NONE', ( #33519, #38162, #12075, #4901 ) ) ;
#20907=MECHANICAL_DESIGN_GEOMETRIC_PRESENTATION_REPRESENTATION('',(#25019),#18440);
#20909=VECTOR ( 'NONE', #47869, 1000.000000000000000 ) ;
#20918=AXIS2_PLACEMENT_3D ( 'NONE', #35788, #39877, #24215 ) ;
#20921=ORIENTED_EDGE ( 'NONE', *, *, #3598, .T. ) ;
#20930=( BOUNDED_CURVE ( )  B_SPLINE_CURVE ( 3, ( #12866, #16219, #35985, #47223 ),
 .UNSPECIFIED., .F., .F. ) 
 B_SPLINE_CURVE_WITH_KNOTS ( ( 4, 4 ),
 ( 3.141592653589793560, 4.712388980384696779 ),
 .UNSPECIFIED. ) 
 CURVE ( )  GEOMETRIC_REPRESENTATION_ITEM ( )  RATIONAL_B_SPLINE_CURVE ( ( 1.000000000000000000, 0.8047378541243634942, 0.8047378541243634942, 1.000000000000000000 ) ) 
 REPRESENTATION_ITEM ( '' )  );
#20934=VECTOR ( 'NONE', #5674, 1000.000000000000000 ) ;
#20936=DIRECTION ( 'NONE',  ( -3.363195139050033768E-16, -0.7071067811865474617, -0.7071067811865475727 ) ) ;
#20937=CARTESIAN_POINT ( 'NONE',  ( 181.0000000000000000, -81.49999999999997158, -340.0000000000001137 ) ) ;
#20940=CARTESIAN_POINT ( 'NONE',  ( -5.000000000000000000, -184.7999999999999545, 340.1999999999997044 ) ) ;
#20942=EDGE_LOOP ( 'NONE', ( #40682, #16348, #15447, #24808 ) ) ;
#20947=VERTEX_POINT ( 'NONE', #2231 ) ;
#20950=CARTESIAN_POINT ( 'NONE',  ( 341.9999999999999432, 181.0000000000001705, -356.0000000000003411 ) ) ;
#20956=VECTOR ( 'NONE', #19873, 1000.000000000000000 ) ;
#20962=CARTESIAN_POINT ( 'NONE',  ( 181.0000000000000000, -5.999999999999950262, -350.0000000000001705 ) ) ;
#20964=ORIENTED_EDGE ( 'NONE', *, *, #12681, .F. ) ;
#20966=CARTESIAN_POINT ( 'NONE',  ( 181.0000000000000000, -79.49999999999997158, -340.0000000000001137 ) ) ;
#20969=EDGE_CURVE ( 'NONE', #11192, #5304, #17868, .T. ) ;
#20970=CARTESIAN_POINT ( 'NONE',  ( -5.000000000000000000, -184.7999999999999545, 359.7999999999997840 ) ) ;
#20971=ADVANCED_FACE ( 'NONE', ( #14527 ), #6839, .T. ) ;
#20976=( LENGTH_UNIT ( ) NAMED_UNIT ( * ) SI_UNIT ( .MILLI., .METRE. ) );
#20977=EDGE_LOOP ( 'NONE', ( #12058, #19908, #34286, #1685 ) ) ;
#20978=CIRCLE ( 'NONE', #42246, 4.000000000000003553 ) ;
#20985=DIRECTION ( 'NONE',  ( 1.110223024625156171E-16, -0.7071067811865474617, 0.7071067811865474617 ) ) ;
#20989=FACE_OUTER_BOUND ( 'NONE', #35829, .T. ) ;
#20990=CARTESIAN_POINT ( 'NONE',  ( 165.0000000000000000, -180.9999999999999716, -115.0000000000001421 ) ) ;
#20997=ORIENTED_EDGE ( 'NONE', *, *, #8468, .T. ) ;
#21004=VECTOR ( 'NONE', #17050, 1000.000000000000000 ) ;
#21014=LINE ( 'NONE', #37193, #354 ) ;
#21019=DIRECTION ( 'NONE',  ( -1.000000000000000000, -0.000000000000000000, -0.000000000000000000 ) ) ;
#21024=DIRECTION ( 'NONE',  ( 1.000000000000000000, 0.000000000000000000, 0.000000000000000000 ) ) ;
#21031=DIRECTION ( 'NONE',  ( 3.364279341222521245E-16, 0.7071067811865474617, -0.7071067811865476838 ) ) ;
#21041=( LENGTH_UNIT ( ) NAMED_UNIT ( * ) SI_UNIT ( .MILLI., .METRE. ) );
#21049=EDGE_LOOP ( 'NONE', ( #33567, #23405, #4801, #26032 ) ) ;
#21054=CYLINDRICAL_SURFACE ( 'NONE', #26491, 4.000000000000003553 ) ;
#21056=DIRECTION ( 'NONE',  ( -1.860490536778032451E-50, 0.000000000000000000, -1.000000000000000000 ) ) ;
#21066=DIRECTION ( 'NONE',  ( 0.000000000000000000, -1.000000000000000000, 3.469446951953611033E-15 ) ) ;
#21071=VECTOR ( 'NONE', #7672, 1000.000000000000000 ) ;
#21078=ORIENTED_EDGE ( 'NONE', *, *, #47118, .T. ) ;
#21080=CARTESIAN_POINT ( 'NONE',  ( 344.0000000000000568, 165.0000000000000000, 349.9999999999998295 ) ) ;
#21087=DIRECTION ( 'NONE',  ( 1.368455531567204171E-48, -1.000000000000000000, -2.265761274745217480E-16 ) ) ;
#21108=LINE ( 'NONE', #5211, #26120 ) ;
#21122=EDGE_CURVE ( 'NONE', #16798, #46080, #17749, .T. ) ;
#21123=DIRECTION ( 'NONE',  ( 1.000000000000000000, -4.758098676964957447E-16, 2.958228394578795584E-31 ) ) ;
#21125=DIRECTION ( 'NONE',  ( 1.333906992743555050E-23, -1.000000000000000000, 0.000000000000000000 ) ) ;
#21135=CARTESIAN_POINT ( 'NONE',  ( 358.0000000000000000, 167.8284271247464972, -342.8284271247466108 ) ) ;
#21142=EDGE_CURVE ( 'NONE', #25272, #2948, #46551, .T. ) ;
#21143=VERTEX_POINT ( 'NONE', #22981 ) ;
#21146=DIRECTION ( 'NONE',  ( 0.000000000000000000, -1.000000000000000000, 3.469446951953611033E-15 ) ) ;
#21149=MANIFOLD_SOLID_BREP ( 'Square tube 20 X 20 X 2(1)[15]', #14630 ) ;
#21157=DIRECTION ( 'NONE',  ( 0.000000000000000000, 0.7071067811865473507, -0.7071067811865476838 ) ) ;
#21163=ORIENTED_EDGE ( 'NONE', *, *, #35294, .T. ) ;
#21170=CARTESIAN_POINT ( 'NONE',  ( 166.9999999999999716, -164.9999999999999432, -344.0000000000001137 ) ) ;
#21182=EDGE_CURVE ( 'NONE', #980, #42696, #33396, .T. ) ;
#21186=CLOSED_SHELL ( 'NONE', ( #33785, #45718, #47504, #3627, #5841, #44016, #46307, #29959, #44168, #5413, #33531, #33127, #34508, #5741, #26187, #2058, #13287, #34707 ) ) ;
#21193=LINE ( 'NONE', #28403, #46215 ) ;
#21201=ORIENTED_EDGE ( 'NONE', *, *, #11103, .T. ) ;
#21205=ORIENTED_EDGE ( 'NONE', *, *, #35919, .T. ) ;
#21217=ORIENTED_EDGE ( 'NONE', *, *, #6826, .F. ) ;
#21224=DIRECTION ( 'NONE',  ( 0.000000000000000000, 0.000000000000000000, 1.000000000000000000 ) ) ;
#21225=ORIENTED_EDGE ( 'NONE', *, *, #36562, .F. ) ;
#21226=AXIS2_PLACEMENT_3D ( 'NONE', #8242, #40296, #39551 ) ;
#21244=CARTESIAN_POINT ( 'NONE',  ( 169.0000000000000000, 165.0000000000000000, 341.9999999999998863 ) ) ;
#21253=DIRECTION ( 'NONE',  ( -1.000000000000000000, 0.000000000000000000, 0.000000000000000000 ) ) ;
#21265=VECTOR ( 'NONE', #7314, 1000.000000000000000 ) ;
#21283=ORIENTED_EDGE ( 'NONE', *, *, #16433, .T. ) ;
#21286=VECTOR ( 'NONE', #47154, 1000.000000000000000 ) ;
#21296=EDGE_LOOP ( 'NONE', ( #21851, #22119, #13518, #18774 ) ) ;
#21309=LINE ( 'NONE', #5150, #34497 ) ;
#21310=EDGE_CURVE ( 'NONE', #2541, #38591, #6283, .T. ) ;
#21313=CARTESIAN_POINT ( 'NONE',  ( 360.0000000000000000, 169.0000000000001990, -344.0000000000002842 ) ) ;
#21316=ORIENTED_EDGE ( 'NONE', *, *, #22169, .T. ) ;
#21317=EDGE_CURVE ( 'NONE', #22263, #11094, #2176, .T. ) ;
#21323=AXIS2_PLACEMENT_3D ( 'NONE', #45708, #19043, #3653 ) ;
#21324=CIRCLE ( 'NONE', #17228, 4.000000000000003553 ) ;
#21333=VERTEX_POINT ( 'NONE', #14980 ) ;
#21343=EDGE_CURVE ( 'NONE', #49858, #50040, #47168, .T. ) ;
#21345=PLANE ( 'NONE',  #21645 ) ;
#21347=VERTEX_POINT ( 'NONE', #50331 ) ;
#21352=FACE_OUTER_BOUND ( 'NONE', #10698, .T. ) ;
#21354=EDGE_LOOP ( 'NONE', ( #41513, #25081, #28028, #49908 ) ) ;
#21360=VECTOR ( 'NONE', #23422, 1000.000000000000000 ) ;
#21363=DIRECTION ( 'NONE',  ( 1.000000000000000000, 0.000000000000000000, 1.612977847700450206E-50 ) ) ;
#21364=ORIENTED_EDGE ( 'NONE', *, *, #35625, .T. ) ;
#21365=DIRECTION ( 'NONE',  ( 1.860490536778032451E-50, 0.000000000000000000, -1.000000000000000000 ) ) ;
#21366=CYLINDRICAL_SURFACE ( 'NONE', #711, 4.000000000000003553 ) ;
#21369=DIRECTION ( 'NONE',  ( -5.551115123125782702E-17, 0.7071067811865477948, 0.7071067811865473507 ) ) ;
#21371=CARTESIAN_POINT ( 'NONE',  ( 181.0000000000000000, 175.0000000000000284, -356.0000000000001705 ) ) ;
#21377=CARTESIAN_POINT ( 'NONE',  ( 181.0000000000000000, -272.4999999999999432, -339.9999999999998863 ) ) ;
#21380=CARTESIAN_POINT ( 'NONE',  ( 185.0000000000000000, -272.5000000000000000, -110.9999999999999005 ) ) ;
#21390=ORIENTED_EDGE ( 'NONE', *, *, #11745, .F. ) ;
#21391=VERTEX_POINT ( 'NONE', #46243 ) ;
#21392=CARTESIAN_POINT ( 'NONE',  ( 168.9999999999999716, -268.5000000000000000, -114.9999999999999147 ) ) ;
#21395=MANIFOLD_SOLID_BREP ( 'Square tube 20 X 20 X 2(1)[12]', #48174 ) ;
#21396=DIRECTION ( 'NONE',  ( -1.000000000000000000, 0.000000000000000000, 0.000000000000000000 ) ) ;
#21398=EDGE_LOOP ( 'NONE', ( #46540, #15511, #28830, #27435 ) ) ;
#21399=VERTEX_POINT ( 'NONE', #2903 ) ;
#21401=EDGE_CURVE ( 'NONE', #12244, #7115, #19069, .T. ) ;
#21402=CARTESIAN_POINT ( 'NONE',  ( 339.9999999999998863, -164.9999999999999432, 343.9999999999997726 ) ) ;
#21404=ORIENTED_EDGE ( 'NONE', *, *, #1218, .F. ) ;
#21405=VERTEX_POINT ( 'NONE', #14723 ) ;
#21413=CARTESIAN_POINT ( 'NONE',  ( 341.9999999999999432, -174.9999999999999432, 343.9999999999998295 ) ) ;
#21416=DIRECTION ( 'NONE',  ( 0.000000000000000000, 1.000000000000000000, 1.544785076050074834E-48 ) ) ;
#21422=LINE ( 'NONE', #47017, #35130 ) ;
#21423=DIRECTION ( 'NONE',  ( 0.000000000000000000, -2.969158215481698263E-48, 1.000000000000000000 ) ) ;
#21424=EDGE_CURVE ( 'NONE', #11094, #44375, #49063, .T. ) ;
#21441=ORIENTED_EDGE ( 'NONE', *, *, #33152, .F. ) ;
#21444=CARTESIAN_POINT ( 'NONE',  ( 357.9999999999998863, -182.1715728752539860, -357.1715728752541281 ) ) ;
#21445=LINE ( 'NONE', #9654, #32037 ) ;
#21446=ORIENTED_EDGE ( 'NONE', *, *, #8974, .T. ) ;
#21448=FACE_OUTER_BOUND ( 'NONE', #39101, .T. ) ;
#21450=ORIENTED_EDGE ( 'NONE', *, *, #11410, .F. ) ;
#21453=ADVANCED_FACE ( 'NONE', ( #103 ), #15737, .F. ) ;
#21458=EDGE_CURVE ( 'NONE', #42814, #2953, #45481, .T. ) ;
#21463=DIRECTION ( 'NONE',  ( 1.000000000000000000, -4.758098676964957447E-16, 2.958228394578795584E-31 ) ) ;
#21465=ORIENTED_EDGE ( 'NONE', *, *, #26928, .T. ) ;
#21471=CARTESIAN_POINT ( 'NONE',  ( 342.8284271247460993, -183.0000000000001137, -358.0000000000003411 ) ) ;
#21474=CARTESIAN_POINT ( 'NONE',  ( 0.000000000000000000, -165.1999999999999602, -340.2000000000001592 ) ) ;
#21477=MANIFOLD_SOLID_BREP ( 'Square tube 20 X 20 X 2(1)[16]', #50667 ) ;
#21488=CARTESIAN_POINT ( 'NONE',  ( 169.0000000000000000, -174.9999999999999716, -95.00000000000014211 ) ) ;
#21491=PLANE ( 'NONE',  #41732 ) ;
#21496=VECTOR ( 'NONE', #647, 1000.000000000000000 ) ;
#21498=VERTEX_POINT ( 'NONE', #32156 ) ;
#21500=CARTESIAN_POINT ( 'NONE',  ( 350.0000000000000000, -184.9999999999999716, -356.0000000000002274 ) ) ;
#21503=VERTEX_POINT ( 'NONE', #4448 ) ;
#21508=DIRECTION ( 'NONE',  ( -1.586032892321652236E-16, -1.000000000000000000, -6.853681917100419162E-49 ) ) ;
#21515=FACE_OUTER_BOUND ( 'NONE', #44925, .T. ) ;
#21516=CARTESIAN_POINT ( 'NONE',  ( 342.0000000000000000, 169.0000000000000000, 343.9999999999998863 ) ) ;
#21523=ADVANCED_FACE ( 'NONE', ( #21604, #14144 ), #22114, .F. ) ;
#21528=ORIENTED_EDGE ( 'NONE', *, *, #47704, .T. ) ;
#21541=ORIENTED_EDGE ( 'NONE', *, *, #13026, .F. ) ;
#21549=PLANE ( 'NONE',  #32294 ) ;
#21556=CARTESIAN_POINT ( 'NONE',  ( 360.0000000000001137, 171.9999999999998295, 3.000000000000003109 ) ) ;
#21557=DIRECTION ( 'NONE',  ( 1.000000000000000000, -4.996003610813203446E-16, 1.033975765691284226E-24 ) ) ;
#21559=ORIENTED_EDGE ( 'NONE', *, *, #1371, .T. ) ;
#21567=CARTESIAN_POINT ( 'NONE',  ( 356.0000000000001137, 165.0000000000000000, 339.9999999999998295 ) ) ;
#21569=VERTEX_POINT ( 'NONE', #41612 ) ;
#21581=DIRECTION ( 'NONE',  ( -1.000000000000000000, -0.000000000000000000, -0.000000000000000000 ) ) ;
#21586=DIRECTION ( 'NONE',  ( 1.000000000000000000, 0.000000000000000000, 0.000000000000000000 ) ) ;
#21587=EDGE_LOOP ( 'NONE', ( #7793, #5501, #11735, #50367, #8891, #9997, #21854, #47987 ) ) ;
#21590=DIRECTION ( 'NONE',  ( 0.000000000000000000, 0.000000000000000000, 1.000000000000000000 ) ) ;
#21598=ORIENTED_EDGE ( 'NONE', *, *, #13718, .F. ) ;
#21601=DIRECTION ( 'NONE',  ( 0.000000000000000000, -2.969158215481698263E-48, 1.000000000000000000 ) ) ;
#21604=FACE_BOUND ( 'NONE', #6592, .T. ) ;
#21615=DIRECTION ( 'NONE',  ( 1.000000000000000000, 0.000000000000000000, 1.612977847700450206E-50 ) ) ;
#21622=DIRECTION ( 'NONE',  ( -1.000000000000000000, 0.000000000000000000, 0.000000000000000000 ) ) ;
#21625=FACE_OUTER_BOUND ( 'NONE', #21049, .T. ) ;
#21630=EDGE_CURVE ( 'NONE', #17911, #32197, #7738, .T. ) ;
#21634=EDGE_CURVE ( 'NONE', #15862, #7447, #15428, .T. ) ;
#21639=DIRECTION ( 'NONE',  ( 0.000000000000000000, 0.000000000000000000, 1.000000000000000000 ) ) ;
#21644=CARTESIAN_POINT ( 'NONE',  ( 350.0000000000000000, 175.0000000000000284, -350.0000000000001705 ) ) ;
#21645=AXIS2_PLACEMENT_3D ( 'NONE', #37034, #1858, #10313 ) ;
#21650=CARTESIAN_POINT ( 'NONE',  ( 350.0000000000001137, 181.0000000000000284, 355.9999999999997726 ) ) ;
#21652=MANIFOLD_SOLID_BREP ( 'Cut-Extrude1[3]', #35172 ) ;
#21660=ORIENTED_EDGE ( 'NONE', *, *, #12940, .F. ) ;
#21662=ADVANCED_FACE ( 'NONE', ( #46689 ), #14921, .F. ) ;
#21669=ORIENTED_EDGE ( 'NONE', *, *, #17045, .T. ) ;
#21673=DIRECTION ( 'NONE',  ( -1.000000000000000000, 0.000000000000000000, 0.000000000000000000 ) ) ;
#21674=AXIS2_PLACEMENT_3D ( 'NONE', #17556, #33227, #44227 ) ;
#21681=DIRECTION ( 'NONE',  ( -1.000000000000000000, 0.000000000000000000, 0.000000000000000000 ) ) ;
#21685=CARTESIAN_POINT ( 'NONE',  ( 339.9999999999998863, 183.3431457505076594, -358.3431457505078583 ) ) ;
#21688=EDGE_LOOP ( 'NONE', ( #2621, #7284, #3145, #31976 ) ) ;
#21689=FACE_OUTER_BOUND ( 'NONE', #26892, .T. ) ;
#21693=AXIS2_PLACEMENT_3D ( 'NONE', #13171, #48024, #40871 ) ;
#21699=DIRECTION ( 'NONE',  ( 0.000000000000000000, 0.000000000000000000, -1.000000000000000000 ) ) ;
#21702=CARTESIAN_POINT ( 'NONE',  ( 168.9999999999999716, -254.5000000000000000, -114.9999999999999574 ) ) ;
#21703=VERTEX_POINT ( 'NONE', #11066 ) ;
#21706=VECTOR ( 'NONE', #28168, 1000.000000000000000 ) ;
#21707=VERTEX_POINT ( 'NONE', #38547 ) ;
#21710=CIRCLE ( 'NONE', #42992, 2.000000000000001776 ) ;
#21714=ORIENTED_EDGE ( 'NONE', *, *, #15577, .T. ) ;
#21721=EDGE_CURVE ( 'NONE', #28407, #46472, #43624, .T. ) ;
#21722=CARTESIAN_POINT ( 'NONE',  ( 356.0000000000001137, 169.0000000000000000, 349.9999999999998295 ) ) ;
#21724=ORIENTED_EDGE ( 'NONE', *, *, #32868, .F. ) ;
#21729=VECTOR ( 'NONE', #48855, 1000.000000000000000 ) ;
#21730=CARTESIAN_POINT ( 'NONE',  ( 181.0000000000000000, 6.000000000000060396, -340.0000000000001137 ) ) ;
#21731=DIRECTION ( 'NONE',  ( 0.000000000000000000, -0.000000000000000000, 1.000000000000000000 ) ) ;
#21741=ADVANCED_FACE ( 'NONE', ( #3874 ), #23630, .T. ) ;
#21746=AXIS2_PLACEMENT_3D ( 'NONE', #28180, #24577, #33301 ) ;
#21747=ORIENTED_EDGE ( 'NONE', *, *, #27593, .T. ) ;
#21749=LINE ( 'NONE', #6353, #41408 ) ;
#21750=EDGE_CURVE ( 'NONE', #38840, #20771, #43132, .T. ) ;
#21756=DIRECTION ( 'NONE',  ( 0.000000000000000000, -1.000000000000000000, -4.687818848539279227E-49 ) ) ;
#21764=ADVANCED_FACE ( 'NONE', ( #20288 ), #1047, .T. ) ;
#21769=FACE_BOUND ( 'NONE', #34096, .T. ) ;
#21787=CARTESIAN_POINT ( 'NONE',  ( 343.9999999999999432, 183.0000000000002274, -358.0000000000003411 ) ) ;
#21788=FACE_OUTER_BOUND ( 'NONE', #30942, .T. ) ;
#21789=VERTEX_POINT ( 'NONE', #41300 ) ;
#21794=EDGE_CURVE ( 'NONE', #45431, #13237, #44612, .T. ) ;
#21803=EDGE_LOOP ( 'NONE', ( #49047, #40901, #48963, #40056 ) ) ;
#21804=DIRECTION ( 'NONE',  ( -1.000000000000000000, 0.000000000000000000, -7.793956916774525800E-48 ) ) ;
#21811=CARTESIAN_POINT ( 'NONE',  ( 168.9999999999999716, -254.4999999999999432, -349.9999999999999432 ) ) ;
#21812=AXIS2_PLACEMENT_3D ( 'NONE', #1589, #17236, #16983 ) ;
#21813=AXIS2_PLACEMENT_3D ( 'NONE', #32083, #19765, #20016 ) ;
#21819=DIRECTION ( 'NONE',  ( -1.000000000000000000, 0.000000000000000000, 1.860490536778032451E-50 ) ) ;
#21826=EDGE_CURVE ( 'NONE', #37534, #17053, #6153, .T. ) ;
#21830=ORIENTED_EDGE ( 'NONE', *, *, #7025, .T. ) ;
#21833=EDGE_LOOP ( 'NONE', ( #48062, #33600, #4242, #16646, #48895, #30843, #11878, #20308 ) ) ;
#21842=VECTOR ( 'NONE', #42395, 1000.000000000000000 ) ;
#21851=ORIENTED_EDGE ( 'NONE', *, *, #23764, .F. ) ;
#21854=ORIENTED_EDGE ( 'NONE', *, *, #16114, .F. ) ;
#21862=CARTESIAN_POINT ( 'NONE',  ( 181.0000000000000000, -97.49999999999998579, -340.0000000000001137 ) ) ;
#21868=CARTESIAN_POINT ( 'NONE',  ( 339.9999999999999432, -171.9999999999999147, -347.0000000000001137 ) ) ;
#21871=VERTEX_POINT ( 'NONE', #44371 ) ;
#21873=CARTESIAN_POINT ( 'NONE',  ( -5.000000000000000000, -165.1999999999999602, -359.8000000000002387 ) ) ;
#21876=CIRCLE ( 'NONE', #32547, 2.000000000000001776 ) ;
#21877=DIRECTION ( 'NONE',  ( 1.333906992743555050E-23, -1.000000000000000000, 0.000000000000000000 ) ) ;
#21878=ORIENTED_EDGE ( 'NONE', *, *, #18322, .F. ) ;
#21883=DIRECTION ( 'NONE',  ( 0.000000000000000000, 0.000000000000000000, 1.000000000000000000 ) ) ;
#21885=EDGE_LOOP ( 'NONE', ( #2619, #9492, #26470, #50435 ) ) ;
#21894=DIRECTION ( 'NONE',  ( 0.000000000000000000, 0.000000000000000000, -1.000000000000000000 ) ) ;
#21905=CARTESIAN_POINT ( 'NONE',  ( 181.0000000000000000, -252.4999999999999432, -339.9999999999998863 ) ) ;
#21907=EDGE_CURVE ( 'NONE', #8209, #39875, #34371, .T. ) ;
#21917=ORIENTED_EDGE ( 'NONE', *, *, #42816, .T. ) ;
#21922=AXIS2_PLACEMENT_3D ( 'NONE', #37364, #29131, #26039 ) ;
#21926=FACE_OUTER_BOUND ( 'NONE', #19555, .T. ) ;
#21927=ORIENTED_EDGE ( 'NONE', *, *, #3520, .T. ) ;
#21928=CARTESIAN_POINT ( 'NONE',  ( 358.0000000000000000, -167.8284271247461845, 342.8284271247460424 ) ) ;
#21931=DIRECTION ( 'NONE',  ( 0.000000000000000000, -1.000000000000000000, 0.000000000000000000 ) ) ;
#21935=CARTESIAN_POINT ( 'NONE',  ( 0.000000000000000000, 181.0000000000000284, 343.9999999999997726 ) ) ;
#21940=CARTESIAN_POINT ( 'NONE',  ( 181.0000000000000000, 165.0000000000000000, -344.0000000000001137 ) ) ;
#21941=DIRECTION ( 'NONE',  ( 0.000000000000000000, 0.000000000000000000, -1.000000000000000000 ) ) ;
#21945=CARTESIAN_POINT ( 'NONE',  ( 342.0000000000000000, 2.999999999999780176, -172.0000000000003126 ) ) ;
#21955=CARTESIAN_POINT ( 'NONE',  ( 342.0000000000000000, -167.8284271247462414, -342.8284271247464972 ) ) ;
#21958=ORIENTED_EDGE ( 'NONE', *, *, #29300, .F. ) ;
#21959=DIRECTION ( 'NONE',  ( -1.586032892321652236E-16, -1.000000000000000000, -2.288264760618012091E-48 ) ) ;
#21960=CARTESIAN_POINT ( 'NONE',  ( 181.0000000000000000, -174.9999999999999716, -356.0000000000001705 ) ) ;
#21961=( BOUNDED_CURVE ( )  B_SPLINE_CURVE ( 3, ( #15071, #46074, #26871, #7896 ),
 .UNSPECIFIED., .F., .F. ) 
 B_SPLINE_CURVE_WITH_KNOTS ( ( 4, 4 ),
 ( 4.712388980384693227, 6.283185307179586232 ),
 .UNSPECIFIED. ) 
 CURVE ( )  GEOMETRIC_REPRESENTATION_ITEM ( )  RATIONAL_B_SPLINE_CURVE ( ( 1.000000000000000000, 0.8047378541243658256, 0.8047378541243658256, 1.000000000000000000 ) ) 
 REPRESENTATION_ITEM ( '' )  );
#21964=CARTESIAN_POINT ( 'NONE',  ( 168.9999999999999716, -174.9999999999999716, -356.0000000000001705 ) ) ;
#21969=DIRECTION ( 'NONE',  ( -0.000000000000000000, 3.186989995019654210E-49, 1.000000000000000000 ) ) ;
#21973=CARTESIAN_POINT ( 'NONE',  ( 350.0000000000001137, 169.0000000000000000, 343.9999999999997726 ) ) ;
#21974=DIRECTION ( 'NONE',  ( 0.000000000000000000, 1.000000000000000000, 0.000000000000000000 ) ) ;
#21976=EDGE_LOOP ( 'NONE', ( #1789, #4380, #17255, #25364 ) ) ;
#21977=ORIENTED_EDGE ( 'NONE', *, *, #35748, .F. ) ;
#21978=CARTESIAN_POINT ( 'NONE',  ( 356.0000000000000000, 175.0000000000000284, -108.0000000000002132 ) ) ;
#21988=CIRCLE ( 'NONE', #31863, 3.749999999999975575 ) ;
#21989=MANIFOLD_SOLID_BREP ( 'Square tube 20 X 20 X 2(1)[11]', #3970 ) ;
#21998=VERTEX_POINT ( 'NONE', #18445 ) ;
#21999=CARTESIAN_POINT ( 'NONE',  ( 339.9999999999999432, -169.0000000000001137, 344.0000000000000000 ) ) ;
#22000=DIRECTION ( 'NONE',  ( -1.000000000000000000, 0.000000000000000000, -1.612977847700450206E-50 ) ) ;
#22007=CARTESIAN_POINT ( 'NONE',  ( 0.000000000000000000, 185.0000000000000284, -344.0000000000001705 ) ) ;
#22012=CARTESIAN_POINT ( 'NONE',  ( 0.000000000000000000, 0.000000000000000000, 0.000000000000000000 ) ) ;
#22013=VECTOR ( 'NONE', #6019, 1000.000000000000000 ) ;
#22019=PLANE ( 'NONE',  #15480 ) ;
#22021=CARTESIAN_POINT ( 'NONE',  ( 168.9999999999999716, -254.4999999999999432, -339.9999999999998863 ) ) ;
#22022=CARTESIAN_POINT ( 'NONE',  ( 341.9999999999999432, 169.0000000000000568, -344.0000000000002842 ) ) ;
#22028=VECTOR ( 'NONE', #1079, 1000.000000000000000 ) ;
#22031=LINE ( 'NONE', #42294, #20413 ) ;
#22033=ORIENTED_EDGE ( 'NONE', *, *, #35406, .F. ) ;
#22034=ORIENTED_EDGE ( 'NONE', *, *, #44390, .T. ) ;
#22035=LINE ( 'NONE', #49193, #48282 ) ;
#22039=EDGE_LOOP ( 'NONE', ( #22868, #7005, #34170, #35170, #13957, #4319, #43495, #37500 ) ) ;
#22057=ORIENTED_EDGE ( 'NONE', *, *, #14350, .F. ) ;
#22063=LINE ( 'NONE', #2560, #9397 ) ;
#22065=VECTOR ( 'NONE', #42698, 1000.000000000000000 ) ;
#22069=ORIENTED_EDGE ( 'NONE', *, *, #40228, .F. ) ;
#22072=MANIFOLD_SOLID_BREP ( 'Square tube 20 X 20 X 2(1)[14]', #10527 ) ;
#22074=CARTESIAN_POINT ( 'NONE',  ( 166.9999999999999716, 6.000000000000060396, 339.9999999999998295 ) ) ;
#22088=EDGE_LOOP ( 'NONE', ( #16857, #37770, #11056, #10157 ) ) ;
#22092=VECTOR ( 'NONE', #47397, 1000.000000000000000 ) ;
#22096=LINE ( 'NONE', #2584, #30539 ) ;
#22102=ORIENTED_EDGE ( 'NONE', *, *, #11250, .F. ) ;
#22108=CARTESIAN_POINT ( 'NONE',  ( 164.9999999999999716, -9.999999999999953815, -99.00000000000014211 ) ) ;
#22114=PLANE ( 'NONE',  #39833 ) ;
#22116=PLANE ( 'NONE',  #30512 ) ;
#22117=VERTEX_POINT ( 'NONE', #2239 ) ;
#22119=ORIENTED_EDGE ( 'NONE', *, *, #45880, .T. ) ;
#22124=DIRECTION ( 'NONE',  ( -1.000000000000000000, 0.000000000000000000, 1.860490536778032451E-50 ) ) ;
#22125=CARTESIAN_POINT ( 'NONE',  ( 341.9999999999999432, -165.0000000000001137, -94.00000000000019895 ) ) ;
#22131=FACE_OUTER_BOUND ( 'NONE', #5099, .T. ) ;
#22133=AXIS2_PLACEMENT_3D ( 'NONE', #39451, #40453, #20425 ) ;
#22134=AXIS2_PLACEMENT_3D ( 'NONE', #10643, #14495, #26557 ) ;
#22135=ADVANCED_FACE ( 'NONE', ( #29439 ), #40238, .F. ) ;
#22136=PLANE ( 'NONE',  #20768 ) ;
#22140=ORIENTED_EDGE ( 'NONE', *, *, #21317, .T. ) ;
#22144=AXIS2_PLACEMENT_3D ( 'NONE', #20780, #36460, #1301 ) ;
#22157=CARTESIAN_POINT ( 'NONE',  ( 339.9999999999999432, 169.0000000000000000, -342.0000000000001705 ) ) ;
#22158=ORIENTED_EDGE ( 'NONE', *, *, #23298, .T. ) ;
#22163=ORIENTED_EDGE ( 'NONE', *, *, #4094, .T. ) ;
#22164=CARTESIAN_POINT ( 'NONE',  ( 340.0000000000000568, 183.0000000000000284, 355.9999999999997726 ) ) ;
#22168=FACE_BOUND ( 'NONE', #34206, .T. ) ;
#22169=EDGE_CURVE ( 'NONE', #39841, #2541, #1742, .T. ) ;
#22170=CIRCLE ( 'NONE', #62, 4.000000000000003553 ) ;
#22175=VECTOR ( 'NONE', #3741, 1000.000000000000000 ) ;
#22183=DIRECTION ( 'NONE',  ( -1.586032892321652482E-16, 0.000000000000000000, -1.000000000000000000 ) ) ;
#22186=ADVANCED_FACE ( 'NONE', ( #49144 ), #30191, .T. ) ;
#22187=CARTESIAN_POINT ( 'NONE',  ( 344.0000000000000000, -165.0000000000001137, -349.9999999999998863 ) ) ;
#22191=CARTESIAN_POINT ( 'NONE',  ( 181.0000000000000284, -174.9999999999999716, -115.0000000000001563 ) ) ;
#22192=ORIENTED_EDGE ( 'NONE', *, *, #41640, .T. ) ;
#22199=DIRECTION ( 'NONE',  ( 0.000000000000000000, 5.664403186863042467E-17, 1.000000000000000000 ) ) ;
#22200=DIRECTION ( 'NONE',  ( -1.000000000000000000, 0.000000000000000000, 0.000000000000000000 ) ) ;
#22216=EDGE_CURVE ( 'NONE', #5029, #49726, #11216, .T. ) ;
#22219=CARTESIAN_POINT ( 'NONE',  ( 342.8284271247462129, 183.0000000000000000, -358.0000000000001137 ) ) ;
#22222=EDGE_LOOP ( 'NONE', ( #33587, #10319, #30751, #29918 ) ) ;
#22226=VERTEX_POINT ( 'NONE', #45307 ) ;
#22227=EDGE_CURVE ( 'NONE', #21569, #23180, #45447, .T. ) ;
#22228=DIRECTION ( 'NONE',  ( 0.000000000000000000, 0.000000000000000000, 1.000000000000000000 ) ) ;
#22236=VECTOR ( 'NONE', #40977, 1000.000000000000000 ) ;
#22240=EDGE_CURVE ( 'NONE', #35337, #17816, #25847, .T. ) ;
#22244=MANIFOLD_SOLID_BREP ( 'Square tube 20 X 20 X 2(1)[18]', #30197 ) ;
#22251=VECTOR ( 'NONE', #41133, 1000.000000000000000 ) ;
#22254=CARTESIAN_POINT ( 'NONE',  ( 181.0000000000000284, -174.9999999999999716, -115.0000000000001563 ) ) ;
#22256=DIRECTION ( 'NONE',  ( -1.000000000000000000, 0.000000000000000000, 0.000000000000000000 ) ) ;
#22260=EDGE_LOOP ( 'NONE', ( #18216, #42890, #8094, #31726 ) ) ;
#22263=VERTEX_POINT ( 'NONE', #4954 ) ;
#22264=DIRECTION ( 'NONE',  ( -1.586032892321652236E-16, -1.000000000000000000, -2.288264760618012091E-48 ) ) ;
#22265=CYLINDRICAL_SURFACE ( 'NONE', #98, 4.000000000000003553 ) ;
#22267=LINE ( 'NONE', #15076, #36483 ) ;
#22271=CARTESIAN_POINT ( 'NONE',  ( 0.000000000000000000, 165.2000000000000171, -359.8000000000002387 ) ) ;
#22275=DIRECTION ( 'NONE',  ( -1.000000000000000000, 0.000000000000000000, 1.860490536778032451E-50 ) ) ;
#22285=DIRECTION ( 'NONE',  ( -1.586032892321652236E-16, -1.000000000000000000, -6.853681917100419162E-49 ) ) ;
#22286=ORIENTED_EDGE ( 'NONE', *, *, #38113, .F. ) ;
#22289=EDGE_LOOP ( 'NONE', ( #38551, #37330, #35474, #45264 ) ) ;
#22296=( NAMED_UNIT ( * ) PLANE_ANGLE_UNIT ( ) SI_UNIT ( $, .RADIAN. ) );
#22304=ORIENTED_EDGE ( 'NONE', *, *, #35606, .F. ) ;
#22309=DIRECTION ( 'NONE',  ( 0.000000000000000000, 0.000000000000000000, 1.000000000000000000 ) ) ;
#22310=VERTEX_POINT ( 'NONE', #12904 ) ;
#22315=CARTESIAN_POINT ( 'NONE',  ( 183.0000000000000000, -164.9999999999999432, 343.9999999999998863 ) ) ;
#22322=ORIENTED_EDGE ( 'NONE', *, *, #13266, .F. ) ;
#22325=VECTOR ( 'NONE', #44229, 1000.000000000000000 ) ;
#22338=DIRECTION ( 'NONE',  ( -1.860490536778032451E-50, 0.000000000000000000, 1.000000000000000000 ) ) ;
#22340=ORIENTED_EDGE ( 'NONE', *, *, #46642, .T. ) ;
#22341=CIRCLE ( 'NONE', #250, 2.000000000000001776 ) ;
#22348=ORIENTED_EDGE ( 'NONE', *, *, #50105, .T. ) ;
#22352=DIRECTION ( 'NONE',  ( 1.000000000000000000, -4.758098676964954489E-16, 2.958228394578795584E-31 ) ) ;
#22354=ORIENTED_EDGE ( 'NONE', *, *, #24038, .F. ) ;
#22358=DIRECTION ( 'NONE',  ( -0.000000000000000000, -1.000000000000000000, 2.537652627714643577E-15 ) ) ;
#22368=VECTOR ( 'NONE', #10969, 1000.000000000000000 ) ;
#22369=CARTESIAN_POINT ( 'NONE',  ( 356.0000000000000000, -165.0000000000001137, 339.9999999999999432 ) ) ;
#22380=AXIS2_PLACEMENT_3D ( 'NONE', #31358, #46949, #11850 ) ;
#22381=CARTESIAN_POINT ( 'NONE',  ( 166.9999999999999716, 6.000000000000060396, -350.0000000000001705 ) ) ;
#22392=VERTEX_POINT ( 'NONE', #8570 ) ;
#22393=LINE ( 'NONE', #30877, #36145 ) ;
#22402=ORIENTED_EDGE ( 'NONE', *, *, #4528, .T. ) ;
#22406=CYLINDRICAL_SURFACE ( 'NONE', #33008, 3.749999999999975575 ) ;
#22415=EDGE_CURVE ( 'NONE', #1107, #32259, #49523, .T. ) ;
#22416=ORIENTED_EDGE ( 'NONE', *, *, #189, .F. ) ;
#22431=DIRECTION ( 'NONE',  ( -0.000000000000000000, -0.000000000000000000, 1.000000000000000000 ) ) ;
#22433=DIRECTION ( 'NONE',  ( 0.000000000000000000, -1.000000000000000000, 2.537652627714642000E-15 ) ) ;
#22440=DIRECTION ( 'NONE',  ( 1.000000000000000000, 0.000000000000000000, 0.000000000000000000 ) ) ;
#22441=VECTOR ( 'NONE', #29476, 1000.000000000000000 ) ;
#22446=FACE_OUTER_BOUND ( 'NONE', #46744, .T. ) ;
#22448=AXIS2_PLACEMENT_3D ( 'NONE', #33018, #13238, #29161 ) ;
#22449=VERTEX_POINT ( 'NONE', #45689 ) ;
#22451=EDGE_CURVE ( 'NONE', #50718, #1522, #16845, .T. ) ;
#22458=VERTEX_POINT ( 'NONE', #26231 ) ;
#22460=ORIENTED_EDGE ( 'NONE', *, *, #43989, .F. ) ;
#22464=ADVANCED_FACE ( 'NONE', ( #25986 ), #25730, .F. ) ;
#22468=CARTESIAN_POINT ( 'NONE',  ( 181.0000000000000000, -174.9999999999999716, -342.0000000000001137 ) ) ;
#22473=FACE_OUTER_BOUND ( 'NONE', #10161, .T. ) ;
#22479=CARTESIAN_POINT ( 'NONE',  ( 358.0000000000000568, 167.8284271247464972, 342.8284271247462129 ) ) ;
#22481=ORIENTED_EDGE ( 'NONE', *, *, #42831, .F. ) ;
#22488=AXIS2_PLACEMENT_3D ( 'NONE', #15670, #15169, #20024 ) ;
#22492=CARTESIAN_POINT ( 'NONE',  ( 350.0000000000001137, 181.0000000000000284, 339.9999999999997726 ) ) ;
#22493=MANIFOLD_SOLID_BREP ( 'Square tube 20 X 20 X 2(1)[1]', #31872 ) ;
#22495=ORIENTED_EDGE ( 'NONE', *, *, #1171, .T. ) ;
#22501=ORIENTED_EDGE ( 'NONE', *, *, #5454, .F. ) ;
#22503=LINE ( 'NONE', #14037, #37342 ) ;
#22508=CARTESIAN_POINT ( 'NONE',  ( 181.0000000000000284, 2.775557561562891351E-14, -113.0000000000001563 ) ) ;
#22512=DIRECTION ( 'NONE',  ( 0.000000000000000000, 0.000000000000000000, 1.000000000000000000 ) ) ;
#22515=EDGE_CURVE ( 'NONE', #9965, #19479, #42114, .T. ) ;
#22518=ORIENTED_EDGE ( 'NONE', *, *, #14345, .F. ) ;
#22521=FACE_OUTER_BOUND ( 'NONE', #12750, .T. ) ;
#22524=CYLINDRICAL_SURFACE ( 'NONE', #14727, 2.000000000000001776 ) ;
#22534=AXIS2_PLACEMENT_3D ( 'NONE', #10154, #41709, #29908 ) ;
#22535=ORIENTED_EDGE ( 'NONE', *, *, #17336, .T. ) ;
#22542=LINE ( 'NONE', #14846, #881 ) ;
#22545=DIRECTION ( 'NONE',  ( 1.000000000000000000, 0.000000000000000000, -1.860490536778032451E-50 ) ) ;
#22550=CIRCLE ( 'NONE', #26665, 2.000000000000001776 ) ;
#22554=EDGE_CURVE ( 'NONE', #38131, #48818, #18763, .T. ) ;
#22557=PLANE ( 'NONE',  #47799 ) ;
#22564=CYLINDRICAL_SURFACE ( 'NONE', #49873, 4.000000000000003553 ) ;
#22565=( BOUNDED_CURVE ( )  B_SPLINE_CURVE ( 3, ( #5648, #5398, #17711, #13836 ),
 .UNSPECIFIED., .F., .F. ) 
 B_SPLINE_CURVE_WITH_KNOTS ( ( 4, 4 ),
 ( 4.712388980384689674, 6.283185307179253165 ),
 .UNSPECIFIED. ) 
 CURVE ( )  GEOMETRIC_REPRESENTATION_ITEM ( )  RATIONAL_B_SPLINE_CURVE ( ( 1.000000000000000000, 0.8047378541243649375, 0.8047378541243649375, 1.000000000000000000 ) ) 
 REPRESENTATION_ITEM ( '' )  );
#22567=DIRECTION ( 'NONE',  ( 0.000000000000000000, -2.265761274745217480E-16, 1.000000000000000000 ) ) ;
#22571=LINE ( 'NONE', #34907, #7590 ) ;
#22575=VECTOR ( 'NONE', #14718, 1000.000000000000000 ) ;
#22578=DIRECTION ( 'NONE',  ( 0.000000000000000000, 2.969158215481698263E-48, -1.000000000000000000 ) ) ;
#22579=AXIS2_PLACEMENT_3D ( 'NONE', #28256, #43887, #20790 ) ;
#22581=VERTEX_POINT ( 'NONE', #35728 ) ;
#22582=LINE ( 'NONE', #42332, #30595 ) ;
#22584=VECTOR ( 'NONE', #11502, 1000.000000000000000 ) ;
#22588=DIRECTION ( 'NONE',  ( 1.000000000000000000, 0.000000000000000000, 1.612977847700450206E-50 ) ) ;
#22602=EDGE_LOOP ( 'NONE', ( #7800, #50143, #29483, #7801 ) ) ;
#22605=ORIENTED_EDGE ( 'NONE', *, *, #39809, .T. ) ;
#22612=FACE_BOUND ( 'NONE', #17410, .T. ) ;
#22616=CIRCLE ( 'NONE', #47992, 4.000000000000003553 ) ;
#22624=AXIS2_PLACEMENT_3D ( 'NONE', #7087, #11194, #15033 ) ;
#22632=CARTESIAN_POINT ( 'NONE',  ( 183.0000000000000000, -256.4999999999999432, -349.9999999999999432 ) ) ;
#22634=AXIS2_PLACEMENT_3D ( 'NONE', #3856, #43351, #39276 ) ;
#22635=( LENGTH_UNIT ( ) NAMED_UNIT ( * ) SI_UNIT ( .MILLI., .METRE. ) );
#22636=ORIENTED_EDGE ( 'NONE', *, *, #33113, .F. ) ;
#22639=CARTESIAN_POINT ( 'NONE',  ( 168.9999999999999716, -164.9999999999999432, -344.0000000000001137 ) ) ;
#22651=ORIENTED_EDGE ( 'NONE', *, *, #48795, .F. ) ;
#22653=CARTESIAN_POINT ( 'NONE',  ( -5.000000000000000000, 175.0000000000000284, 346.2500000000002274 ) ) ;
#22659=CARTESIAN_POINT ( 'NONE',  ( 344.0000000000000568, 167.0000000000000000, 341.9999999999998863 ) ) ;
#22663=EDGE_CURVE ( 'NONE', #27818, #26389, #36540, .T. ) ;
#22665=DIRECTION ( 'NONE',  ( 0.000000000000000000, -2.265761274745217480E-16, 1.000000000000000000 ) ) ;
#22666=AXIS2_PLACEMENT_3D ( 'NONE', #9975, #2772, #1781 ) ;
#22671=ORIENTED_EDGE ( 'NONE', *, *, #40725, .F. ) ;
#22672=ORIENTED_EDGE ( 'NONE', *, *, #22998, .T. ) ;
#22673=CARTESIAN_POINT ( 'NONE',  ( 340.0000000000001137, 183.3431457505076594, 358.3431457505074604 ) ) ;
#22674=CARTESIAN_POINT ( 'NONE',  ( 181.0000000000000000, -164.9999999999999432, 343.9999999999998863 ) ) ;
#22676=DIRECTION ( 'NONE',  ( 1.586032892321652236E-16, 1.000000000000000000, 6.853681917100419162E-49 ) ) ;
#22687=LINE ( 'NONE', #2188, #41330 ) ;
#22688=ORIENTED_EDGE ( 'NONE', *, *, #25406, .T. ) ;
#22702=ADVANCED_FACE ( 'NONE', ( #7405 ), #46095, .F. ) ;
#22704=FACE_BOUND ( 'NONE', #792, .T. ) ;
#22706=CARTESIAN_POINT ( 'NONE',  ( 356.0000000000000568, 175.0000000000000284, -92.00000000000019895 ) ) ;
#22709=EDGE_LOOP ( 'NONE', ( #41320, #19393, #23088, #17162 ) ) ;
#22723=VERTEX_POINT ( 'NONE', #26890 ) ;
#22728=ORIENTED_EDGE ( 'NONE', *, *, #30543, .T. ) ;
#22729=CARTESIAN_POINT ( 'NONE',  ( 181.0000000000000000, -168.9999999999999432, -350.0000000000001705 ) ) ;
#22732=ADVANCED_FACE ( 'NONE', ( #35382 ), #50180, .F. ) ;
#22738=ADVANCED_FACE ( 'NONE', ( #50448 ), #23558, .F. ) ;
#22739=ORIENTED_EDGE ( 'NONE', *, *, #35355, .F. ) ;
#22740=DIRECTION ( 'NONE',  ( -3.172065784643302499E-16, -1.000000000000000000, 2.537652627714641605E-15 ) ) ;
#22742=EDGE_CURVE ( 'NONE', #45973, #27971, #15852, .T. ) ;
#22746=CARTESIAN_POINT ( 'NONE',  ( 356.0000000000000000, 165.0000000000000000, -106.0000000000001990 ) ) ;
#22748=( LENGTH_UNIT ( ) NAMED_UNIT ( * ) SI_UNIT ( .MILLI., .METRE. ) );
#22756=CARTESIAN_POINT ( 'NONE',  ( 344.0000000000000000, -167.0000000000001137, 342.0000000000000000 ) ) ;
#22761=ORIENTED_EDGE ( 'NONE', *, *, #7992, .T. ) ;
#22764=CARTESIAN_POINT ( 'NONE',  ( 339.9999999999999432, 165.0000000000000000, -344.0000000000001705 ) ) ;
#22768=CARTESIAN_POINT ( 'NONE',  ( 360.0000000000000000, 181.0000000000000284, -356.0000000000001705 ) ) ;
#22778=CARTESIAN_POINT ( 'NONE',  ( 357.9999999999999432, 174.9999999999996589, -356.0000000000003411 ) ) ;
#22782=DIRECTION ( 'NONE',  ( -2.775557561562891351E-16, -0.7071067811865477948, -0.7071067811865473507 ) ) ;
#22784=CARTESIAN_POINT ( 'NONE',  ( 344.0000000000000568, 169.0000000000000000, 349.9999999999998295 ) ) ;
#22793=ORIENTED_EDGE ( 'NONE', *, *, #33065, .T. ) ;
#22799=DIRECTION ( 'NONE',  ( 0.000000000000000000, 1.000000000000000000, 3.186989995019654210E-49 ) ) ;
#22805=CARTESIAN_POINT ( 'NONE',  ( 168.9999999999999716, -95.49999999999997158, -115.0000000000001563 ) ) ;
#22812=EDGE_CURVE ( 'NONE', #913, #50273, #18675, .T. ) ;
#22820=EDGE_CURVE ( 'NONE', #37811, #5747, #42290, .T. ) ;
#22823=CARTESIAN_POINT ( 'NONE',  ( 339.9999999999998863, -168.9999999999999716, -360.0000000000003411 ) ) ;
#22827=VERTEX_POINT ( 'NONE', #37461 ) ;
#22832=ORIENTED_EDGE ( 'NONE', *, *, #34471, .T. ) ;
#22855=VECTOR ( 'NONE', #49882, 1000.000000000000000 ) ;
#22861=ORIENTED_EDGE ( 'NONE', *, *, #42456, .T. ) ;
#22868=ORIENTED_EDGE ( 'NONE', *, *, #28499, .T. ) ;
#22881=DIRECTION ( 'NONE',  ( 1.000000000000000000, 0.000000000000000000, 0.000000000000000000 ) ) ;
#22891=DIRECTION ( 'NONE',  ( -1.942330104924128867E-32, 0.000000000000000000, -1.000000000000000000 ) ) ;
#22898=VERTEX_POINT ( 'NONE', #45844 ) ;
#22903=VECTOR ( 'NONE', #254, 1000.000000000000000 ) ;
#22907=LINE ( 'NONE', #38586, #20589 ) ;
#22911=VERTEX_POINT ( 'NONE', #38964 ) ;
#22913=CARTESIAN_POINT ( 'NONE',  ( 183.0000000000000000, -174.9999999999999716, -356.0000000000001705 ) ) ;
#22914=MANIFOLD_SOLID_BREP ( 'Square tube 20 X 20 X 2(1)[6]', #2363 ) ;
#22915=DIRECTION ( 'NONE',  ( 0.000000000000000000, 0.000000000000000000, 1.000000000000000000 ) ) ;
#22922=ORIENTED_EDGE ( 'NONE', *, *, #31822, .F. ) ;
#22932=CIRCLE ( 'NONE', #24555, 4.000000000000003553 ) ;
#22933=ORIENTED_EDGE ( 'NONE', *, *, #18598, .F. ) ;
#22934=DIRECTION ( 'NONE',  ( 0.000000000000000000, 1.000000000000000000, 0.000000000000000000 ) ) ;
#22936=DIRECTION ( 'NONE',  ( 0.000000000000000000, 0.000000000000000000, 1.000000000000000000 ) ) ;
#22946=DIRECTION ( 'NONE',  ( 0.000000000000000000, 1.000000000000000000, -2.969158215481698263E-48 ) ) ;
#22961=ORIENTED_EDGE ( 'NONE', *, *, #35914, .T. ) ;
#22967=ORIENTED_EDGE ( 'NONE', *, *, #44628, .F. ) ;
#22970=VECTOR ( 'NONE', #47882, 1000.000000000000000 ) ;
#22972=DIRECTION ( 'NONE',  ( -0.000000000000000000, -1.000000000000000000, 2.537652627714643577E-15 ) ) ;
#22973=DIRECTION ( 'NONE',  ( 0.000000000000000000, 5.664403186863042467E-17, 1.000000000000000000 ) ) ;
#22975=CARTESIAN_POINT ( 'NONE',  ( 0.000000000000000000, 0.000000000000000000, 0.000000000000000000 ) ) ;
#22981=CARTESIAN_POINT ( 'NONE',  ( 344.0000000000000000, 165.0000000000001990, -340.0000000000002842 ) ) ;
#22985=CARTESIAN_POINT ( 'NONE',  ( 350.0000000000000000, 181.0000000000000284, -358.0000000000002274 ) ) ;
#22991=DIRECTION ( 'NONE',  ( 0.000000000000000000, 0.000000000000000000, -1.000000000000000000 ) ) ;
#22993=DIRECTION ( 'NONE',  ( 0.000000000000000000, 0.000000000000000000, -1.000000000000000000 ) ) ;
#22994=CARTESIAN_POINT ( 'NONE',  ( -5.000000000000000000, -184.7999999999999545, 359.7999999999997840 ) ) ;
#22998=EDGE_CURVE ( 'NONE', #18651, #9239, #23559, .T. ) ;
#22999=VECTOR ( 'NONE', #17158, 1000.000000000000000 ) ;
#23000=LINE ( 'NONE', #10697, #19956 ) ;
#23008=DIRECTION ( 'NONE',  ( -7.793956916774525800E-48, 0.000000000000000000, -1.000000000000000000 ) ) ;
#23015=ORIENTED_EDGE ( 'NONE', *, *, #3628, .T. ) ;
#23019=ORIENTED_EDGE ( 'NONE', *, *, #24683, .T. ) ;
#23022=EDGE_CURVE ( 'NONE', #46658, #38055, #8690, .T. ) ;
#23023=EDGE_CURVE ( 'NONE', #24437, #37912, #31014, .T. ) ;
#23026=CYLINDRICAL_SURFACE ( 'NONE', #17543, 2.000000000000001776 ) ;
#23028=EDGE_CURVE ( 'NONE', #6887, #14195, #47106, .T. ) ;
#23032=VECTOR ( 'NONE', #37826, 1000.000000000000000 ) ;
#23036=ORIENTED_EDGE ( 'NONE', *, *, #21634, .F. ) ;
#23039=VERTEX_POINT ( 'NONE', #32536 ) ;
#23044=CARTESIAN_POINT ( 'NONE',  ( 181.0000000000000000, -268.4999999999999432, -339.9999999999998863 ) ) ;
#23058=DIRECTION ( 'NONE',  ( -1.000000000000000000, 0.000000000000000000, -1.586032872232979935E-16 ) ) ;
#23060=CARTESIAN_POINT ( 'NONE',  ( 166.9999999999999716, -256.4999999999999432, -349.9999999999999432 ) ) ;
#23062=CYLINDRICAL_SURFACE ( 'NONE', #46134, 4.000000000000003553 ) ;
#23067=DIRECTION ( 'NONE',  ( 3.172065745548403743E-16, 1.000000000000000000, 0.000000000000000000 ) ) ;
#23080=CARTESIAN_POINT ( 'NONE',  ( 169.0000000000000568, -166.9999999999999432, -115.0000000000001847 ) ) ;
#23082=VECTOR ( 'NONE', #7384, 1000.000000000000000 ) ;
#23088=ORIENTED_EDGE ( 'NONE', *, *, #24297, .T. ) ;
#23094=CARTESIAN_POINT ( 'NONE',  ( 164.9999999999999716, -256.4999999999999432, -349.9999999999999432 ) ) ;
#23095=ORIENTED_EDGE ( 'NONE', *, *, #8408, .F. ) ;
#23097=ORIENTED_EDGE ( 'NONE', *, *, #15224, .F. ) ;
#23098=CARTESIAN_POINT ( 'NONE',  ( 339.9999999999999432, 183.0000000000000284, -356.0000000000002274 ) ) ;
#23107=CIRCLE ( 'NONE', #1002, 2.000000000000001776 ) ;
#23117=VECTOR ( 'NONE', #7470, 1000.000000000000000 ) ;
#23122=ORIENTED_EDGE ( 'NONE', *, *, #19532, .F. ) ;
#23123=ORIENTED_EDGE ( 'NONE', *, *, #18583, .F. ) ;
#23130=ORIENTED_EDGE ( 'NONE', *, *, #3312, .F. ) ;
#23131=CARTESIAN_POINT ( 'NONE',  ( 168.9999999999999716, -5.999999999999950262, -350.0000000000001705 ) ) ;
#23140=CIRCLE ( 'NONE', #9231, 2.000000000000001776 ) ;
#23148=ADVANCED_FACE ( 'NONE', ( #5051 ), #14007, .T. ) ;
#23149=AXIS2_PLACEMENT_3D ( 'NONE', #16263, #44197, #47271 ) ;
#23164=EDGE_LOOP ( 'NONE', ( #33584, #33238, #48198, #35002 ) ) ;
#23166=DIRECTION ( 'NONE',  ( -0.000000000000000000, -1.000000000000000000, 2.537652627714643577E-15 ) ) ;
#23170=EDGE_CURVE ( 'NONE', #47056, #13420, #16079, .T. ) ;
#23176=CARTESIAN_POINT ( 'NONE',  ( 181.0000000000000000, -95.49999999999998579, -350.0000000000001705 ) ) ;
#23177=CYLINDRICAL_SURFACE ( 'NONE', #14049, 4.000000000000003553 ) ;
#23178=VERTEX_POINT ( 'NONE', #33788 ) ;
#23180=VERTEX_POINT ( 'NONE', #18611 ) ;
#23181=DIRECTION ( 'NONE',  ( 0.000000000000000000, 0.000000000000000000, -1.000000000000000000 ) ) ;
#23186=ORIENTED_EDGE ( 'NONE', *, *, #6265, .T. ) ;
#23188=EDGE_LOOP ( 'NONE', ( #3125, #26392, #40057, #710, #25819, #23594, #11412, #37632 ) ) ;
#23189=CARTESIAN_POINT ( 'NONE',  ( 169.0000000000000000, 2.775557561562891351E-14, -95.00000000000014211 ) ) ;
#23197=DIRECTION ( 'NONE',  ( 0.000000000000000000, 0.000000000000000000, -1.000000000000000000 ) ) ;
#23202=CARTESIAN_POINT ( 'NONE',  ( 342.0000000000000568, 169.0000000000000000, 349.9999999999998863 ) ) ;
#23206=DIRECTION ( 'NONE',  ( 0.000000000000000000, 0.000000000000000000, -1.000000000000000000 ) ) ;
#23207=ORIENTED_EDGE ( 'NONE', *, *, #13619, .F. ) ;
#23208=LINE ( 'NONE', #3967, #36871 ) ;
#23217=AXIS2_PLACEMENT_3D ( 'NONE', #41632, #10344, #45192 ) ;
#23220=CARTESIAN_POINT ( 'NONE',  ( 4.999999999999999112, -175.0000000000000284, -353.7500000000001705 ) ) ;
#23226=LINE ( 'NONE', #30955, #44676 ) ;
#23244=FACE_OUTER_BOUND ( 'NONE', #14133, .T. ) ;
#23252=STYLED_ITEM('',(#50747),#39816);
#23253=EDGE_CURVE ( 'NONE', #11545, #26016, #2224, .T. ) ;
#23257=CARTESIAN_POINT ( 'NONE',  ( 166.9999999999999716, -93.50000000000005684, -340.0000000000001137 ) ) ;
#23267=CARTESIAN_POINT ( 'NONE',  ( 185.0000000000000000, -93.49999999999998579, -340.0000000000001137 ) ) ;
#23272=ORIENTED_EDGE ( 'NONE', *, *, #28385, .T. ) ;
#23275=FACE_OUTER_BOUND ( 'NONE', #21976, .T. ) ;
#23278=VECTOR ( 'NONE', #35312, 1000.000000000000000 ) ;
#23280=VECTOR ( 'NONE', #19801, 1000.000000000000000 ) ;
#23283=CIRCLE ( 'NONE', #1196, 2.000000000000001776 ) ;
#23287=DIRECTION ( 'NONE',  ( -1.000000000000000000, 0.000000000000000000, 0.000000000000000000 ) ) ;
#23294=ORIENTED_EDGE ( 'NONE', *, *, #10781, .T. ) ;
#23298=EDGE_CURVE ( 'NONE', #18793, #3991, #39159, .T. ) ;
#23299=DIRECTION ( 'NONE',  ( 0.000000000000000000, 0.000000000000000000, 1.000000000000000000 ) ) ;
#23316=EDGE_CURVE ( 'NONE', #22117, #26100, #41489, .T. ) ;
#23326=ORIENTED_EDGE ( 'NONE', *, *, #873, .T. ) ;
#23327=FACE_BOUND ( 'NONE', #13634, .T. ) ;
#23330=CARTESIAN_POINT ( 'NONE',  ( 344.0000000000000000, -167.0000000000001137, -342.0000000000002842 ) ) ;
#23338=CARTESIAN_POINT ( 'NONE',  ( 339.9999999999998863, -185.0000000000001421, 355.9999999999997726 ) ) ;
#23340=ORIENTED_EDGE ( 'NONE', *, *, #26476, .T. ) ;
#23341=CARTESIAN_POINT ( 'NONE',  ( 340.0000000000000568, 185.0000000000000284, 343.9999999999997726 ) ) ;
#23346=EDGE_CURVE ( 'NONE', #45648, #4709, #30692, .T. ) ;
#23355=CYLINDRICAL_SURFACE ( 'NONE', #6250, 4.000000000000003553 ) ;
#23359=FACE_OUTER_BOUND ( 'NONE', #17606, .T. ) ;
#23361=CARTESIAN_POINT ( 'NONE',  ( 339.9999999999999432, 181.0000000000000284, -356.0000000000002274 ) ) ;
#23366=DIRECTION ( 'NONE',  ( 1.000000000000000000, 0.000000000000000000, 0.000000000000000000 ) ) ;
#23368=DIRECTION ( 'NONE',  ( 1.000000000000000000, 0.000000000000000000, 0.000000000000000000 ) ) ;
#23370=DIRECTION ( 'NONE',  ( 6.203854594147707562E-25, -2.067951531382569187E-25, 1.000000000000000000 ) ) ;
#23385=CARTESIAN_POINT ( 'NONE',  ( 341.6568542494923690, -164.9999999999999716, 339.9999999999998295 ) ) ;
#23387=VECTOR ( 'NONE', #5235, 1000.000000000000000 ) ;
#23388=EDGE_CURVE ( 'NONE', #27797, #49664, #44175, .T. ) ;
#23396=EDGE_CURVE ( 'NONE', #43423, #34859, #524, .T. ) ;
#23397=CIRCLE ( 'NONE', #34068, 4.000000000000003553 ) ;
#23399=CARTESIAN_POINT ( 'NONE',  ( 339.9999999999999432, -164.9999999999999432, -356.0000000000002274 ) ) ;
#23401=ADVANCED_FACE ( 'NONE', ( #10049 ), #16995, .F. ) ;
#23404=CARTESIAN_POINT ( 'NONE',  ( 0.000000000000000000, 165.2000000000000171, 340.1999999999997044 ) ) ;
#23405=ORIENTED_EDGE ( 'NONE', *, *, #35355, .T. ) ;
#23408=VECTOR ( 'NONE', #5122, 1000.000000000000000 ) ;
#23417=EDGE_LOOP ( 'NONE', ( #50131, #2596, #43230, #3462 ) ) ;
#23419=EDGE_CURVE ( 'NONE', #30554, #14213, #37737, .T. ) ;
#23422=DIRECTION ( 'NONE',  ( 1.000000000000000000, 0.000000000000000000, 0.000000000000000000 ) ) ;
#23423=DIRECTION ( 'NONE',  ( 4.758098676964956461E-16, 1.000000000000000000, 0.000000000000000000 ) ) ;
#23426=UNCERTAINTY_MEASURE_WITH_UNIT (LENGTH_MEASURE( 1.000000000000000082E-05 ), #10973, 'distance_accuracy_value', 'NONE');
#23430=DIRECTION ( 'NONE',  ( -0.000000000000000000, -6.123233995736766036E-17, 1.000000000000000000 ) ) ;
#23431=ORIENTED_EDGE ( 'NONE', *, *, #17092, .F. ) ;
#23434=DIRECTION ( 'NONE',  ( -4.758098676964956461E-16, 0.000000000000000000, -1.000000000000000000 ) ) ;
#23451=ORIENTED_EDGE ( 'NONE', *, *, #37886, .F. ) ;
#23455=VERTEX_POINT ( 'NONE', #5188 ) ;
#23459=EDGE_CURVE ( 'NONE', #37912, #16652, #8727, .T. ) ;
#23465=EDGE_CURVE ( 'NONE', #891, #47169, #48248, .T. ) ;
#23466=ADVANCED_FACE ( 'NONE', ( #24954, #40603 ), #2344, .T. ) ;
#23479=LINE ( 'NONE', #3445, #19761 ) ;
#23482=AXIS2_PLACEMENT_3D ( 'NONE', #5436, #36771, #1604 ) ;
#23487=ORIENTED_EDGE ( 'NONE', *, *, #35999, .T. ) ;
#23489=LINE ( 'NONE', #19372, #34079 ) ;
#23490=CIRCLE ( 'NONE', #25102, 3.749999999999975575 ) ;
#23492=VERTEX_POINT ( 'NONE', #37284 ) ;
#23500=VERTEX_POINT ( 'NONE', #7215 ) ;
#23502=LINE ( 'NONE', #26333, #34910 ) ;
#23507=DIRECTION ( 'NONE',  ( -3.172065784643302499E-16, -1.000000000000000000, 2.537652627714642000E-15 ) ) ;
#23512=CARTESIAN_POINT ( 'NONE',  ( 166.9999999999999716, -184.9999999999999716, -344.0000000000001137 ) ) ;
#23537=ORIENTED_EDGE ( 'NONE', *, *, #12430, .T. ) ;
#23553=DIRECTION ( 'NONE',  ( 0.000000000000000000, 0.000000000000000000, -1.000000000000000000 ) ) ;
#23554=DIRECTION ( 'NONE',  ( -1.586032892321652236E-16, -1.000000000000000000, -6.853681917100419162E-49 ) ) ;
#23555=ORIENTED_EDGE ( 'NONE', *, *, #13688, .T. ) ;
#23557=CARTESIAN_POINT ( 'NONE',  ( 169.0000000000000000, 2.775557561562891351E-14, -111.0000000000001563 ) ) ;
#23558=PLANE ( 'NONE',  #27507 ) ;
#23559=LINE ( 'NONE', #19704, #16043 ) ;
#23562=CARTESIAN_POINT ( 'NONE',  ( 339.9999999999999432, -168.9999999999999432, -356.0000000000002274 ) ) ;
#23567=CARTESIAN_POINT ( 'NONE',  ( 167.0000000000000000, -168.9999999999993747, -115.0000000000001847 ) ) ;
#23574=AXIS2_PLACEMENT_3D ( 'NONE', #41994, #41490, #49141 ) ;
#23575=DIRECTION ( 'NONE',  ( -0.000000000000000000, -1.000000000000000000, -0.000000000000000000 ) ) ;
#23576=CARTESIAN_POINT ( 'NONE',  ( 181.0000000000000000, -184.9999999999999716, -344.0000000000001137 ) ) ;
#23579=FACE_OUTER_BOUND ( 'NONE', #21354, .T. ) ;
#23584=EDGE_CURVE ( 'NONE', #15590, #541, #2588, .T. ) ;
#23585=CARTESIAN_POINT ( 'NONE',  ( 181.0000000000000568, 175.0000000000000284, 343.9999999999998863 ) ) ;
#23587=CARTESIAN_POINT ( 'NONE',  ( 5.551115123125782702E-14, -168.9999999999999432, 343.9999999999997726 ) ) ;
#23594=ORIENTED_EDGE ( 'NONE', *, *, #43218, .F. ) ;
#23603=CARTESIAN_POINT ( 'NONE',  ( 341.6568542494922553, -165.0000000000001137, -340.0000000000002842 ) ) ;
#23604=VERTEX_POINT ( 'NONE', #41852 ) ;
#23610=DIRECTION ( 'NONE',  ( 0.000000000000000000, -0.000000000000000000, -1.000000000000000000 ) ) ;
#23623=ORIENTED_EDGE ( 'NONE', *, *, #10586, .F. ) ;
#23627=LINE ( 'NONE', #7734, #50087 ) ;
#23630=PLANE ( 'NONE',  #11982 ) ;
#23645=ORIENTED_EDGE ( 'NONE', *, *, #9852, .T. ) ;
#23648=FACE_OUTER_BOUND ( 'NONE', #20942, .T. ) ;
#23652=DIRECTION ( 'NONE',  ( 2.958228394578793832E-31, 0.000000000000000000, 1.000000000000000000 ) ) ;
#23654=CARTESIAN_POINT ( 'NONE',  ( 343.9999999999999432, -174.9999999999999432, 359.9999999999998295 ) ) ;
#23659=DIRECTION ( 'NONE',  ( 0.000000000000000000, -1.000000000000000000, -3.186989995019654210E-49 ) ) ;
#23660=( NAMED_UNIT ( * ) SI_UNIT ( $, .STERADIAN. ) SOLID_ANGLE_UNIT ( ) );
#23661=ORIENTED_EDGE ( 'NONE', *, *, #42760, .T. ) ;
#23662=CARTESIAN_POINT ( 'NONE',  ( 181.0000000000000000, -272.4999999999999432, -339.9999999999998863 ) ) ;
#23666=CARTESIAN_POINT ( 'NONE',  ( 169.0000000000000000, -174.9999999999999716, -111.0000000000001563 ) ) ;
#23668=DIRECTION ( 'NONE',  ( 1.333906992743555050E-23, -1.000000000000000000, 0.000000000000000000 ) ) ;
#23669=ORIENTED_EDGE ( 'NONE', *, *, #24063, .T. ) ;
#23670=EDGE_CURVE ( 'NONE', #13422, #47734, #31844, .T. ) ;
#23671=VERTEX_POINT ( 'NONE', #15419 ) ;
#23674=AXIS2_PLACEMENT_3D ( 'NONE', #14992, #41681, #6294 ) ;
#23676=ADVANCED_FACE ( 'NONE', ( #32087 ), #39794, .T. ) ;
#23687=ORIENTED_EDGE ( 'NONE', *, *, #29644, .F. ) ;
#23688=EDGE_CURVE ( 'NONE', #50585, #48233, #8745, .T. ) ;
#23690=AXIS2_PLACEMENT_3D ( 'NONE', #37233, #48446, #44863 ) ;
#23692=AXIS2_PLACEMENT_3D ( 'NONE', #37013, #14633, #1832 ) ;
#23694=VERTEX_POINT ( 'NONE', #35708 ) ;
#23696=ORIENTED_EDGE ( 'NONE', *, *, #4094, .F. ) ;
#23699=CARTESIAN_POINT ( 'NONE',  ( 183.0000000000000000, -81.49999999999997158, -350.0000000000001705 ) ) ;
#23703=EDGE_CURVE ( 'NONE', #14213, #31506, #11829, .T. ) ;
#23705=ORIENTED_EDGE ( 'NONE', *, *, #5754, .F. ) ;
#23707=CARTESIAN_POINT ( 'NONE',  ( 0.000000000000000000, 181.0000000000000284, -360.0000000000002274 ) ) ;
#23710=EDGE_CURVE ( 'NONE', #44854, #42571, #27589, .T. ) ;
#23712=CARTESIAN_POINT ( 'NONE',  ( 166.9999999999999716, -272.5000000000000000, -110.9999999999999005 ) ) ;
#23718=VECTOR ( 'NONE', #20936, 1000.000000000000000 ) ;
#23721=DIRECTION ( 'NONE',  ( -0.000000000000000000, 1.000000000000000000, 0.000000000000000000 ) ) ;
#23733=VERTEX_POINT ( 'NONE', #35447 ) ;
#23736=DIRECTION ( 'NONE',  ( 2.775557561562891351E-16, 0.7071067811865477948, 0.7071067811865473507 ) ) ;
#23737=ADVANCED_FACE ( 'NONE', ( #11574 ), #8489, .F. ) ;
#23740=ORIENTED_EDGE ( 'NONE', *, *, #28688, .F. ) ;
#23744=DIRECTION ( 'NONE',  ( 0.000000000000000000, 2.537652627714643577E-15, 1.000000000000000000 ) ) ;
#23750=EDGE_CURVE ( 'NONE', #50718, #36234, #31337, .T. ) ;
#23755=VECTOR ( 'NONE', #42693, 1000.000000000000000 ) ;
#23756=FACE_OUTER_BOUND ( 'NONE', #33041, .T. ) ;
#23761=DIRECTION ( 'NONE',  ( -1.000000000000000000, 1.586032892321652236E-16, 1.586032892321651989E-16 ) ) ;
#23764=EDGE_CURVE ( 'NONE', #48770, #46883, #9481, .T. ) ;
#23765=DIRECTION ( 'NONE',  ( -1.586032892321652236E-16, -1.000000000000000000, -2.288264760618012091E-48 ) ) ;
#23766=EDGE_LOOP ( 'NONE', ( #30684, #9488, #9826, #26676 ) ) ;
#23767=ORIENTED_EDGE ( 'NONE', *, *, #41926, .F. ) ;
#23769=EDGE_LOOP ( 'NONE', ( #1645, #17406, #6687, #33480 ) ) ;
#23774=ORIENTED_EDGE ( 'NONE', *, *, #25661, .T. ) ;
#23777=DIRECTION ( 'NONE',  ( 1.000000000000000000, 0.000000000000000000, -4.758098676964956461E-16 ) ) ;
#23779=( BOUNDED_CURVE ( )  B_SPLINE_CURVE ( 3, ( #10314, #25710, #25972, #49511 ),
 .UNSPECIFIED., .F., .F. ) 
 B_SPLINE_CURVE_WITH_KNOTS ( ( 4, 4 ),
 ( 3.141592653589793116, 4.712388980384693227 ),
 .UNSPECIFIED. ) 
 CURVE ( )  GEOMETRIC_REPRESENTATION_ITEM ( )  RATIONAL_B_SPLINE_CURVE ( ( 1.000000000000000000, 0.8047378541243641603, 0.8047378541243641603, 1.000000000000000000 ) ) 
 REPRESENTATION_ITEM ( '' )  );
#23780=LINE ( 'NONE', #11983, #48237 ) ;
#23792=CARTESIAN_POINT ( 'NONE',  ( 181.0000000000000000, -272.4999999999999432, -339.9999999999998863 ) ) ;
#23802=EDGE_CURVE ( 'NONE', #34812, #29100, #48934, .T. ) ;
#23804=EDGE_LOOP ( 'NONE', ( #3422, #12310, #46836, #7743 ) ) ;
#23810=LINE ( 'NONE', #12758, #20909 ) ;
#23813=EDGE_CURVE ( 'NONE', #9286, #16306, #2045, .T. ) ;
#23820=ORIENTED_EDGE ( 'NONE', *, *, #8244, .F. ) ;
#23821=DIRECTION ( 'NONE',  ( -7.793956916774524585E-48, 0.000000000000000000, -1.000000000000000000 ) ) ;
#23822=ADVANCED_FACE ( 'NONE', ( #24890 ), #13582, .F. ) ;
#23828=CARTESIAN_POINT ( 'NONE',  ( 340.0000000000000568, 181.0000000000000284, 355.9999999999998295 ) ) ;
#23830=CYLINDRICAL_SURFACE ( 'NONE', #16179, 4.000000000000003553 ) ;
#23839=FACE_BOUND ( 'NONE', #11685, .T. ) ;
#23862=EDGE_LOOP ( 'NONE', ( #40980, #13091, #49446, #974 ) ) ;
#23872=DIRECTION ( 'NONE',  ( 0.000000000000000000, -1.000000000000000000, 0.000000000000000000 ) ) ;
#23878=EDGE_CURVE ( 'NONE', #12755, #27291, #25391, .T. ) ;
#23880=ORIENTED_EDGE ( 'NONE', *, *, #29405, .F. ) ;
#23884=CYLINDRICAL_SURFACE ( 'NONE', #14090, 2.000000000000001776 ) ;
#23891=AXIS2_PLACEMENT_3D ( 'NONE', #39742, #12778, #35898 ) ;
#23895=PLANE ( 'NONE',  #30764 ) ;
#23896=CARTESIAN_POINT ( 'NONE',  ( 356.0000000000000000, -165.0000000000001137, -94.00000000000019895 ) ) ;
#23899=CARTESIAN_POINT ( 'NONE',  ( 343.9999999999999432, -185.0000000000000284, 359.9999999999998295 ) ) ;
#23902=DIRECTION ( 'NONE',  ( 1.000000000000000000, 0.000000000000000000, 0.000000000000000000 ) ) ;
#23903=LINE ( 'NONE', #12344, #13321 ) ;
#23908=EDGE_LOOP ( 'NONE', ( #15718, #26406, #38888, #16487 ) ) ;
#23911=LINE ( 'NONE', #16974, #6003 ) ;
#23929=CARTESIAN_POINT ( 'NONE',  ( 344.0000000000000000, 175.0000000000000284, -106.0000000000001990 ) ) ;
#23937=VERTEX_POINT ( 'NONE', #32599 ) ;
#23951=FACE_OUTER_BOUND ( 'NONE', #46554, .T. ) ;
#23952=EDGE_LOOP ( 'NONE', ( #47469, #20083, #37706, #35222 ) ) ;
#23955=ADVANCED_FACE ( 'NONE', ( #34115 ), #42043, .T. ) ;
#23956=DIRECTION ( 'NONE',  ( 1.000000000000000000, 0.000000000000000000, 0.000000000000000000 ) ) ;
#23965=AXIS2_PLACEMENT_3D ( 'NONE', #20600, #36280, #48010 ) ;
#23969=EDGE_CURVE ( 'NONE', #11650, #7708, #46216, .T. ) ;
#23970=CIRCLE ( 'NONE', #31378, 4.000000000000003553 ) ;
#23975=CARTESIAN_POINT ( 'NONE',  ( 358.3431457505076310, 165.0000000000002274, -340.0000000000002842 ) ) ;
#23982=DIRECTION ( 'NONE',  ( 0.000000000000000000, 0.000000000000000000, -1.000000000000000000 ) ) ;
#23984=DIRECTION ( 'NONE',  ( 0.000000000000000000, -1.000000000000000000, 0.000000000000000000 ) ) ;
#23987=VERTEX_POINT ( 'NONE', #15103 ) ;
#23991=EDGE_CURVE ( 'NONE', #47198, #45035, #445, .T. ) ;
#23999=CARTESIAN_POINT ( 'NONE',  ( 181.0000000000000000, -97.49999999999998579, -350.0000000000001705 ) ) ;
#24008=DIRECTION ( 'NONE',  ( -7.793956916774524585E-48, 0.000000000000000000, -1.000000000000000000 ) ) ;
#24011=DIRECTION ( 'NONE',  ( 1.000000000000000000, -0.000000000000000000, 0.000000000000000000 ) ) ;
#24014=DIRECTION ( 'NONE',  ( 0.000000000000000000, 0.000000000000000000, 1.000000000000000000 ) ) ;
#24016=ORIENTED_EDGE ( 'NONE', *, *, #16404, .F. ) ;
#24019=EDGE_CURVE ( 'NONE', #2059, #13008, #16017, .T. ) ;
#24032=CARTESIAN_POINT ( 'NONE',  ( 168.9999999999999716, -272.4999999999999432, -341.9999999999999432 ) ) ;
#24036=VECTOR ( 'NONE', #6360, 1000.000000000000000 ) ;
#24038=EDGE_CURVE ( 'NONE', #5374, #42585, #22550, .T. ) ;
#24039=CARTESIAN_POINT ( 'NONE',  ( 168.9999999999999716, -7.999999999999952038, 339.9999999999998295 ) ) ;
#24040=VECTOR ( 'NONE', #1938, 1000.000000000000000 ) ;
#24042=LINE ( 'NONE', #20940, #29111 ) ;
#24045=EDGE_CURVE ( 'NONE', #2948, #5419, #46286, .T. ) ;
#24047=ORIENTED_EDGE ( 'NONE', *, *, #42164, .T. ) ;
#24048=DIRECTION ( 'NONE',  ( 0.000000000000000000, 0.000000000000000000, -1.000000000000000000 ) ) ;
#24063=EDGE_CURVE ( 'NONE', #15809, #10936, #42540, .T. ) ;
#24065=CARTESIAN_POINT ( 'NONE',  ( 344.0000000000000568, 167.0000000000000000, 341.9999999999998863 ) ) ;
#24069=DIRECTION ( 'NONE',  ( 0.000000000000000000, 0.000000000000000000, -1.000000000000000000 ) ) ;
#24075=CARTESIAN_POINT ( 'NONE',  ( 359.9999999999999432, -181.0000000000001421, 356.0000000000000000 ) ) ;
#24084=STYLED_ITEM('',(#50747),#39561);
#24085=CARTESIAN_POINT ( 'NONE',  ( 339.9999999999999432, -168.9999999999999432, -344.0000000000001705 ) ) ;
#24091=PLANE ( 'NONE',  #23891 ) ;
#24099=EDGE_CURVE ( 'NONE', #15667, #16553, #39228, .T. ) ;
#24100=CIRCLE ( 'NONE', #31456, 2.000000000000001776 ) ;
#24115=VECTOR ( 'NONE', #1283, 1000.000000000000000 ) ;
#24116=CARTESIAN_POINT ( 'NONE',  ( 164.9999999999999716, -93.49999999999998579, -350.0000000000001705 ) ) ;
#24118=ORIENTED_EDGE ( 'NONE', *, *, #14543, .T. ) ;
#24121=CARTESIAN_POINT ( 'NONE',  ( 344.0000000000000568, 167.0000000000000000, 341.9999999999998863 ) ) ;
#24123=EDGE_CURVE ( 'NONE', #36125, #19216, #46614, .T. ) ;
#24125=DIRECTION ( 'NONE',  ( -3.172065784643302499E-16, -1.000000000000000000, 0.000000000000000000 ) ) ;
#24127=AXIS2_PLACEMENT_3D ( 'NONE', #12809, #28468, #24125 ) ;
#24132=CARTESIAN_POINT ( 'NONE',  ( 167.0000000000000000, -174.9999999999999716, -99.00000000000014211 ) ) ;
#24137=CARTESIAN_POINT ( 'NONE',  ( 164.9999999999999716, -272.4999999999999432, -349.9999999999999432 ) ) ;
#24147=FACE_OUTER_BOUND ( 'NONE', #45887, .T. ) ;
#24150=DIRECTION ( 'NONE',  ( -1.586032892321652236E-16, 3.421138828918010427E-49, -1.000000000000000000 ) ) ;
#24152=AXIS2_PLACEMENT_3D ( 'NONE', #44972, #37581, #37339 ) ;
#24163=FACE_OUTER_BOUND ( 'NONE', #15413, .T. ) ;
#24170=ORIENTED_EDGE ( 'NONE', *, *, #38744, .T. ) ;
#24174=CARTESIAN_POINT ( 'NONE',  ( 343.9999999999999432, -165.0000000000001137, -106.0000000000001990 ) ) ;
#24177=ADVANCED_FACE ( 'NONE', ( #43809 ), #13013, .T. ) ;
#24184=CARTESIAN_POINT ( 'NONE',  ( 359.9999999999998295, 183.3431457505078015, -358.3431457505079152 ) ) ;
#24185=VERTEX_POINT ( 'NONE', #44299 ) ;
#24189=CARTESIAN_POINT ( 'NONE',  ( 360.0000000000000568, 169.0000000000000284, 343.9999999999998863 ) ) ;
#24190=CARTESIAN_POINT ( 'NONE',  ( 4.999999999999999112, 175.0000000000000284, -350.0000000000002274 ) ) ;
#24197=DIRECTION ( 'NONE',  ( 1.000000000000000000, 0.000000000000000000, 0.000000000000000000 ) ) ;
#24199=ORIENTED_EDGE ( 'NONE', *, *, #23802, .T. ) ;
#24201=EDGE_CURVE ( 'NONE', #26366, #46042, #9677, .T. ) ;
#24206=ORIENTED_EDGE ( 'NONE', *, *, #34597, .F. ) ;
#24207=VERTEX_POINT ( 'NONE', #36913 ) ;
#24208=LINE ( 'NONE', #32155, #8299 ) ;
#24209=LINE ( 'NONE', #48509, #43708 ) ;
#24213=CARTESIAN_POINT ( 'NONE',  ( 344.0000000000000000, 167.0000000000001990, -342.0000000000002842 ) ) ;
#24215=DIRECTION ( 'NONE',  ( -1.000000000000000000, 0.000000000000000000, 0.000000000000000000 ) ) ;
#24216=ORIENTED_EDGE ( 'NONE', *, *, #50355, .T. ) ;
#24220=DIRECTION ( 'NONE',  ( -0.000000000000000000, 1.000000000000000000, 6.123233995736766036E-17 ) ) ;
#24223=AXIS2_PLACEMENT_3D ( 'NONE', #23044, #8430, #7666 ) ;
#24244=CARTESIAN_POINT ( 'NONE',  ( 181.0000000000000000, -164.9999999999999432, -342.0000000000001137 ) ) ;
#24255=VERTEX_POINT ( 'NONE', #5060 ) ;
#24266=VECTOR ( 'NONE', #9596, 1000.000000000000000 ) ;
#24268=EDGE_CURVE ( 'NONE', #23500, #14588, #38035, .T. ) ;
#24269=EDGE_CURVE ( 'NONE', #9972, #6508, #1488, .T. ) ;
#24270=CYLINDRICAL_SURFACE ( 'NONE', #4961, 4.000000000000003553 ) ;
#24272=EDGE_LOOP ( 'NONE', ( #29093, #36348, #34870, #34736 ) ) ;
#24282=VECTOR ( 'NONE', #50376, 1000.000000000000000 ) ;
#24287=CARTESIAN_POINT ( 'NONE',  ( 0.000000000000000000, 181.0000000000000284, -340.0000000000001705 ) ) ;
#24292=CARTESIAN_POINT ( 'NONE',  ( 358.0000000000001137, 180.9999999999999716, 355.9999999999997726 ) ) ;
#24296=EDGE_CURVE ( 'NONE', #41468, #4473, #32545, .T. ) ;
#24297=EDGE_CURVE ( 'NONE', #28175, #15426, #36545, .T. ) ;
#24300=EDGE_CURVE ( 'NONE', #3318, #9286, #11948, .T. ) ;
#24303=EDGE_CURVE ( 'NONE', #19185, #18367, #11497, .T. ) ;
#24306=CARTESIAN_POINT ( 'NONE',  ( 358.0000000000001137, 171.9999999999998295, 3.000000000000002665 ) ) ;
#24314=EDGE_LOOP ( 'NONE', ( #12419, #33224, #15410, #41338 ) ) ;
#24315=ORIENTED_EDGE ( 'NONE', *, *, #3172, .T. ) ;
#24318=AXIS2_PLACEMENT_3D ( 'NONE', #39221, #28172, #7658 ) ;
#24327=ORIENTED_EDGE ( 'NONE', *, *, #14300, .T. ) ;
#24335=LINE ( 'NONE', #11505, #44999 ) ;
#24342=DIRECTION ( 'NONE',  ( 1.000000000000000000, -3.172065799423185948E-16, 1.587271980518778491E-16 ) ) ;
#24345=DIRECTION ( 'NONE',  ( -3.172065784643302499E-16, -1.000000000000000000, 2.537652627714642000E-15 ) ) ;
#24349=CARTESIAN_POINT ( 'NONE',  ( 360.0000000000000568, 165.0000000000000000, -94.00000000000019895 ) ) ;
#24350=CARTESIAN_POINT ( 'NONE',  ( -5.000000000000000000, -165.1999999999999602, 340.1999999999997044 ) ) ;
#24353=DIRECTION ( 'NONE',  ( 0.000000000000000000, -1.000000000000000000, 3.469446951953611033E-15 ) ) ;
#24356=AXIS2_PLACEMENT_3D ( 'NONE', #1606, #10310, #24956 ) ;
#24360=DIRECTION ( 'NONE',  ( 0.000000000000000000, 0.000000000000000000, -1.000000000000000000 ) ) ;
#24364=ORIENTED_EDGE ( 'NONE', *, *, #22216, .F. ) ;
#24366=DIRECTION ( 'NONE',  ( 0.000000000000000000, -1.000000000000000000, 0.000000000000000000 ) ) ;
#24372=VERTEX_POINT ( 'NONE', #18871 ) ;
#24386=DIRECTION ( 'NONE',  ( 0.000000000000000000, 0.000000000000000000, -1.000000000000000000 ) ) ;
#24390=AXIS2_PLACEMENT_3D ( 'NONE', #42732, #2981, #30972 ) ;
#24393=ORIENTED_EDGE ( 'NONE', *, *, #34201, .F. ) ;
#24397=DIRECTION ( 'NONE',  ( 1.000000000000000000, 0.000000000000000000, 4.758098658057970186E-16 ) ) ;
#24398=ORIENTED_EDGE ( 'NONE', *, *, #48979, .T. ) ;
#24409=EDGE_CURVE ( 'NONE', #1177, #45648, #14019, .T. ) ;
#24412=VERTEX_POINT ( 'NONE', #45554 ) ;
#24419=ORIENTED_EDGE ( 'NONE', *, *, #16124, .T. ) ;
#24420=DIRECTION ( 'NONE',  ( -0.000000000000000000, -0.000000000000000000, 1.000000000000000000 ) ) ;
#24427=CARTESIAN_POINT ( 'NONE',  ( 342.0000000000000000, 175.0000000000000284, -94.00000000000019895 ) ) ;
#24430=CARTESIAN_POINT ( 'NONE',  ( 341.9999999999999432, -182.1715728752539576, -357.1715728752541281 ) ) ;
#24432=DIRECTION ( 'NONE',  ( -1.000000000000000000, 0.000000000000000000, 0.000000000000000000 ) ) ;
#24435=CARTESIAN_POINT ( 'NONE',  ( 0.000000000000000000, -165.1999999999999602, -359.8000000000002387 ) ) ;
#24436=CARTESIAN_POINT ( 'NONE',  ( 0.000000000000000000, 169.0000000000000000, -344.0000000000001705 ) ) ;
#24437=VERTEX_POINT ( 'NONE', #416 ) ;
#24441=CARTESIAN_POINT ( 'NONE',  ( 356.0000000000000000, 174.9999999999996589, -342.0000000000002842 ) ) ;
#24451=PLANE ( 'NONE',  #29729 ) ;
#24464=EDGE_CURVE ( 'NONE', #9708, #10975, #30966, .T. ) ;
#24465=CARTESIAN_POINT ( 'NONE',  ( 358.0000000000000568, 182.1715728752538439, -357.1715728752539576 ) ) ;
#24471=LINE ( 'NONE', #1122, #40104 ) ;
#24473=FACE_OUTER_BOUND ( 'NONE', #36511, .T. ) ;
#24480=DIRECTION ( 'NONE',  ( 0.000000000000000000, 1.000000000000000000, 0.000000000000000000 ) ) ;
#24484=DIRECTION ( 'NONE',  ( 0.000000000000000000, -1.000000000000000000, -3.186989995019654210E-49 ) ) ;
#24488=EDGE_CURVE ( 'NONE', #38490, #8840, #27103, .T. ) ;
#24490=ORIENTED_EDGE ( 'NONE', *, *, #39068, .T. ) ;
#24492=FACE_OUTER_BOUND ( 'NONE', #23417, .T. ) ;
#24496=ORIENTED_EDGE ( 'NONE', *, *, #20011, .T. ) ;
#24500=ORIENTED_EDGE ( 'NONE', *, *, #813, .F. ) ;
#24502=CARTESIAN_POINT ( 'NONE',  ( 181.0000000000000284, -9.999999999999953815, -99.00000000000014211 ) ) ;
#24511=ORIENTED_EDGE ( 'NONE', *, *, #16749, .F. ) ;
#24512=ORIENTED_EDGE ( 'NONE', *, *, #16433, .F. ) ;
#24536=AXIS2_PLACEMENT_3D ( 'NONE', #29893, #50540, #26305 ) ;
#24550=ORIENTED_EDGE ( 'NONE', *, *, #41794, .F. ) ;
#24555=AXIS2_PLACEMENT_3D ( 'NONE', #36943, #1760, #37187 ) ;
#24556=VECTOR ( 'NONE', #44320, 1000.000000000000000 ) ;
#24557=ORIENTED_EDGE ( 'NONE', *, *, #46642, .F. ) ;
#24560=EDGE_LOOP ( 'NONE', ( #33276, #29752, #25514, #24315 ) ) ;
#24566=LINE ( 'NONE', #16872, #6176 ) ;
#24576=EDGE_CURVE ( 'NONE', #25177, #9422, #8114, .T. ) ;
#24577=DIRECTION ( 'NONE',  ( -1.000000000000000000, 0.000000000000000000, 0.000000000000000000 ) ) ;
#24582=LINE ( 'NONE', #25777, #15785 ) ;
#24591=AXIS2_PLACEMENT_3D ( 'NONE', #37950, #10719, #38959 ) ;
#24592=CIRCLE ( 'NONE', #22133, 2.000000000000001776 ) ;
#24594=UNCERTAINTY_MEASURE_WITH_UNIT (LENGTH_MEASURE( 1.000000000000000082E-05 ), #8368, 'distance_accuracy_value', 'NONE');
#24598=VECTOR ( 'NONE', #5059, 1000.000000000000000 ) ;
#24604=EDGE_CURVE ( 'NONE', #8293, #43828, #27620, .T. ) ;
#24611=CARTESIAN_POINT ( 'NONE',  ( 344.0000000000000568, 165.0000000000000000, 339.9999999999998295 ) ) ;
#24615=CYLINDRICAL_SURFACE ( 'NONE', #29776, 2.000000000000001776 ) ;
#24618=VERTEX_POINT ( 'NONE', #48319 ) ;
#24619=CARTESIAN_POINT ( 'NONE',  ( 350.0000000000000000, -182.9999999999999716, -344.0000000000001705 ) ) ;
#24621=ORIENTED_EDGE ( 'NONE', *, *, #5599, .F. ) ;
#24628=PLANE ( 'NONE',  #16586 ) ;
#24630=ADVANCED_FACE ( 'NONE', ( #40170 ), #8859, .T. ) ;
#24631=ORIENTED_EDGE ( 'NONE', *, *, #8308, .T. ) ;
#24633=DIRECTION ( 'NONE',  ( -1.000000000000000000, 0.000000000000000000, -7.793956916774525800E-48 ) ) ;
#24643=AXIS2_PLACEMENT_3D ( 'NONE', #11833, #46432, #34687 ) ;
#24644=DIRECTION ( 'NONE',  ( 0.000000000000000000, -5.664403186863042467E-17, -1.000000000000000000 ) ) ;
#24656=VERTEX_POINT ( 'NONE', #36599 ) ;
#24662=CARTESIAN_POINT ( 'NONE',  ( -5.000000000000000000, 165.2000000000000171, 359.7999999999997840 ) ) ;
#24664=DIRECTION ( 'NONE',  ( 6.203854594147707562E-25, -2.067951531382569187E-25, 1.000000000000000000 ) ) ;
#24665=CARTESIAN_POINT ( 'NONE',  ( 360.0000000000000000, -169.0000000000001137, -344.0000000000003411 ) ) ;
#24670=AXIS2_PLACEMENT_3D ( 'NONE', #10465, #34086, #26105 ) ;
#24675=EDGE_LOOP ( 'NONE', ( #30163, #16665, #45460, #44654 ) ) ;
#24683=EDGE_CURVE ( 'NONE', #23180, #18208, #44986, .T. ) ;
#24701=CARTESIAN_POINT ( 'NONE',  ( 169.0000000000000284, 165.0000000000000000, 357.9999999999998863 ) ) ;
#24703=ORIENTED_EDGE ( 'NONE', *, *, #21424, .F. ) ;
#24705=CARTESIAN_POINT ( 'NONE',  ( 0.000000000000000000, -180.9999999999999716, -356.0000000000002274 ) ) ;
#24710=DIRECTION ( 'NONE',  ( 6.203854594147707562E-25, -2.067951531382569187E-25, 1.000000000000000000 ) ) ;
#24718=CYLINDRICAL_SURFACE ( 'NONE', #23965, 2.000000000000001776 ) ;
#24721=DIRECTION ( 'NONE',  ( 1.000000000000000000, 0.000000000000000000, 2.958228394578794708E-31 ) ) ;
#24725=CARTESIAN_POINT ( 'NONE',  ( 164.9999999999999716, -164.9999999999999432, 343.9999999999998863 ) ) ;
#24727=CARTESIAN_POINT ( 'NONE',  ( 166.9999999999999716, -168.9999999999999432, -340.0000000000001137 ) ) ;
#24728=CARTESIAN_POINT ( 'NONE',  ( 340.0000000000000568, 167.0000000000000000, 355.9999999999997726 ) ) ;
#24732=CARTESIAN_POINT ( 'NONE',  ( 181.0000000000000568, 165.0000000000000000, 355.9999999999998863 ) ) ;
#24733=EDGE_CURVE ( 'NONE', #6508, #541, #11784, .T. ) ;
#24734=FACE_OUTER_BOUND ( 'NONE', #48046, .T. ) ;
#24737=CARTESIAN_POINT ( 'NONE',  ( -5.000000000000000000, -165.1999999999999602, -359.8000000000002387 ) ) ;
#24738=EDGE_LOOP ( 'NONE', ( #8247, #23451, #10707, #28401 ) ) ;
#24740=VECTOR ( 'NONE', #17601, 1000.000000000000000 ) ;
#24745=VERTEX_POINT ( 'NONE', #33241 ) ;
#24746=ADVANCED_FACE ( 'NONE', ( #21926 ), #38093, .F. ) ;
#24748=ORIENTED_EDGE ( 'NONE', *, *, #2457, .T. ) ;
#24752=CARTESIAN_POINT ( 'NONE',  ( 168.9999999999999716, -174.9999999999999716, -340.0000000000001137 ) ) ;
#24755=VERTEX_POINT ( 'NONE', #37847 ) ;
#24756=ORIENTED_EDGE ( 'NONE', *, *, #32958, .T. ) ;
#24759=VERTEX_POINT ( 'NONE', #49818 ) ;
#24764=CARTESIAN_POINT ( 'NONE',  ( 360.0000000000001137, 181.0000000000000568, 355.9999999999998863 ) ) ;
#24766=EDGE_LOOP ( 'NONE', ( #46573, #2604, #32933, #21225 ) ) ;
#24771=( BOUNDED_CURVE ( )  B_SPLINE_CURVE ( 3, ( #21567, #25425, #5916, #37259 ),
 .UNSPECIFIED., .F., .F. ) 
 B_SPLINE_CURVE_WITH_KNOTS ( ( 4, 4 ),
 ( 8.635508522760760582E-16, 1.570796326794897002 ),
 .UNSPECIFIED. ) 
 CURVE ( )  GEOMETRIC_REPRESENTATION_ITEM ( )  RATIONAL_B_SPLINE_CURVE ( ( 1.000000000000000000, 0.8047378541243650485, 0.8047378541243650485, 1.000000000000000000 ) ) 
 REPRESENTATION_ITEM ( '' )  );
#24774=CARTESIAN_POINT ( 'NONE',  ( 359.9999999999999432, 166.6568542494923975, -341.6568542494925396 ) ) ;
#24775=VECTOR ( 'NONE', #9552, 1000.000000000000000 ) ;
#24786=DIRECTION ( 'NONE',  ( 0.000000000000000000, -3.186989995019654210E-49, -1.000000000000000000 ) ) ;
#24789=EDGE_LOOP ( 'NONE', ( #40621, #35161, #44984, #19423 ) ) ;
#24793=CARTESIAN_POINT ( 'NONE',  ( 359.9999999999998863, -183.3431457505077731, -358.3431457505079152 ) ) ;
#24794=DIRECTION ( 'NONE',  ( -0.000000000000000000, -1.000000000000000000, 2.537652627714643577E-15 ) ) ;
#24807=DIRECTION ( 'NONE',  ( 0.000000000000000000, 0.000000000000000000, -1.000000000000000000 ) ) ;
#24808=ORIENTED_EDGE ( 'NONE', *, *, #16276, .F. ) ;
#24811=DIRECTION ( 'NONE',  ( 0.000000000000000000, -1.000000000000000000, -3.186989995019654210E-49 ) ) ;
#24815=CARTESIAN_POINT ( 'NONE',  ( 341.9999999999999432, -169.0000000000001137, -344.0000000000002842 ) ) ;
#24825=DIRECTION ( 'NONE',  ( 0.000000000000000000, 1.580451535867971417E-48, -1.000000000000000000 ) ) ;
#24829=ORIENTED_EDGE ( 'NONE', *, *, #8964, .F. ) ;
#24833=EDGE_LOOP ( 'NONE', ( #43539, #50547, #50151, #37720 ) ) ;
#24838=CARTESIAN_POINT ( 'NONE',  ( 350.0000000000001137, 175.0000000000000000, 349.9999999999998295 ) ) ;
#24841=DIRECTION ( 'NONE',  ( 0.000000000000000000, 0.000000000000000000, 1.000000000000000000 ) ) ;
#24849=EDGE_LOOP ( 'NONE', ( #10435, #29522, #46723, #37567 ) ) ;
#24851=CARTESIAN_POINT ( 'NONE',  ( 168.9999999999999716, -166.9999999999999432, -115.0000000000001847 ) ) ;
#24865=ORIENTED_EDGE ( 'NONE', *, *, #25889, .F. ) ;
#24867=FACE_OUTER_BOUND ( 'NONE', #8342, .T. ) ;
#24871=CARTESIAN_POINT ( 'NONE',  ( 350.0000000000001137, 175.0000000000000284, 349.9999999999998295 ) ) ;
#24875=CARTESIAN_POINT ( 'NONE',  ( 355.9999999999999432, -183.0000000000001421, -349.9999999999998863 ) ) ;
#24879=MECHANICAL_DESIGN_GEOMETRIC_PRESENTATION_REPRESENTATION('',(#24084),#9310);
#24881=EDGE_CURVE ( 'NONE', #50273, #43723, #24100, .T. ) ;
#24890=FACE_OUTER_BOUND ( 'NONE', #32416, .T. ) ;
#24892=EDGE_CURVE ( 'NONE', #1975, #17667, #3681, .T. ) ;
#24895=CARTESIAN_POINT ( 'NONE',  ( 168.9999999999999716, 175.0000000000000284, -340.0000000000001137 ) ) ;
#24910=VECTOR ( 'NONE', #7648, 1000.000000000000000 ) ;
#24918=EDGE_CURVE ( 'NONE', #24759, #26029, #11645, .T. ) ;
#24919=VECTOR ( 'NONE', #4782, 1000.000000000000000 ) ;
#24922=ORIENTED_EDGE ( 'NONE', *, *, #3172, .F. ) ;
#24924=DIRECTION ( 'NONE',  ( 1.132880637372608740E-16, 4.718402560806925739E-50, 1.000000000000000000 ) ) ;
#24925=ORIENTED_EDGE ( 'NONE', *, *, #4243, .F. ) ;
#24932=DIRECTION ( 'NONE',  ( -1.000000000000000000, 0.000000000000000000, -2.958228394578794270E-31 ) ) ;
#24939=CARTESIAN_POINT ( 'NONE',  ( 185.0000000000000284, -81.49999999999988631, -115.0000000000001563 ) ) ;
#24945=PLANE ( 'NONE',  #8737 ) ;
#24946=ORIENTED_EDGE ( 'NONE', *, *, #36517, .T. ) ;
#24951=ORIENTED_EDGE ( 'NONE', *, *, #3692, .F. ) ;
#24954=FACE_BOUND ( 'NONE', #9122, .T. ) ;
#24956=DIRECTION ( 'NONE',  ( 0.000000000000000000, -1.000000000000000000, 0.000000000000000000 ) ) ;
#24960=EDGE_CURVE ( 'NONE', #22117, #21998, #24209, .T. ) ;
#24961=EDGE_CURVE ( 'NONE', #43962, #7928, #24968, .T. ) ;
#24963=VERTEX_POINT ( 'NONE', #12391 ) ;
#24966=ADVANCED_FACE ( 'NONE', ( #4450 ), #8309, .T. ) ;
#24968=LINE ( 'NONE', #35783, #4418 ) ;
#24973=DIRECTION ( 'NONE',  ( 1.000000000000000000, 0.000000000000000000, -1.860490536778032451E-50 ) ) ;
#24977=DIRECTION ( 'NONE',  ( 0.000000000000000000, 0.000000000000000000, 1.000000000000000000 ) ) ;
#24980=CARTESIAN_POINT ( 'NONE',  ( 341.9999999999999432, -181.0000000000001421, -356.0000000000003411 ) ) ;
#24998=LINE ( 'NONE', #36812, #43443 ) ;
#25008=ORIENTED_EDGE ( 'NONE', *, *, #47216, .F. ) ;
#25014=AXIS2_PLACEMENT_3D ( 'NONE', #33941, #49530, #18523 ) ;
#25019=STYLED_ITEM('',(#50747),#22244);
#25020=EDGE_CURVE ( 'NONE', #11492, #26100, #20346, .T. ) ;
#25027=EDGE_CURVE ( 'NONE', #27082, #35344, #28811, .T. ) ;
#25042=LINE ( 'NONE', #40182, #10299 ) ;
#25044=ADVANCED_FACE ( 'NONE', ( #21352 ), #13658, .T. ) ;
#25054=AXIS2_PLACEMENT_3D ( 'NONE', #11501, #46362, #34867 ) ;
#25060=EDGE_LOOP ( 'NONE', ( #44688, #39951, #4926, #28341, #11224, #42514, #44741, #17547 ) ) ;
#25067=ORIENTED_EDGE ( 'NONE', *, *, #21310, .T. ) ;
#25068=CARTESIAN_POINT ( 'NONE',  ( 342.0000000000000568, 181.0000000000000284, 349.9999999999998863 ) ) ;
#25069=DIRECTION ( 'NONE',  ( 0.000000000000000000, 0.000000000000000000, 1.000000000000000000 ) ) ;
#25076=CIRCLE ( 'NONE', #29179, 4.000000000000003553 ) ;
#25078=DIRECTION ( 'NONE',  ( -1.000000000000000000, 0.000000000000000000, -1.612977847700450206E-50 ) ) ;
#25081=ORIENTED_EDGE ( 'NONE', *, *, #8276, .T. ) ;
#25082=VECTOR ( 'NONE', #18859, 1000.000000000000000 ) ;
#25084=VERTEX_POINT ( 'NONE', #9560 ) ;
#25085=CARTESIAN_POINT ( 'NONE',  ( 183.0000000000000284, -174.9999999999999716, -111.0000000000001563 ) ) ;
#25094=FACE_OUTER_BOUND ( 'NONE', #42780, .T. ) ;
#25096=AXIS2_PLACEMENT_3D ( 'NONE', #5202, #39871, #17004 ) ;
#25101=PLANE ( 'NONE',  #2279 ) ;
#25102=AXIS2_PLACEMENT_3D ( 'NONE', #41846, #21581, #14394 ) ;
#25105=ORIENTED_EDGE ( 'NONE', *, *, #45940, .F. ) ;
#25112=VECTOR ( 'NONE', #26712, 1000.000000000000000 ) ;
#25119=EDGE_LOOP ( 'NONE', ( #17299, #24419, #30827, #20649 ) ) ;
#25125=AXIS2_PLACEMENT_3D ( 'NONE', #27226, #23370, #39036 ) ;
#25126=ORIENTED_EDGE ( 'NONE', *, *, #26632, .T. ) ;
#25130=VECTOR ( 'NONE', #33994, 1000.000000000000000 ) ;
#25135=( BOUNDED_CURVE ( )  B_SPLINE_CURVE ( 3, ( #32183, #23975, #8580, #20624 ),
 .UNSPECIFIED., .F., .F. ) 
 B_SPLINE_CURVE_WITH_KNOTS ( ( 4, 4 ),
 ( 1.586958686267286008E-16, 1.570796326794896780 ),
 .UNSPECIFIED. ) 
 CURVE ( )  GEOMETRIC_REPRESENTATION_ITEM ( )  RATIONAL_B_SPLINE_CURVE ( ( 1.000000000000000000, 0.8047378541243649375, 0.8047378541243649375, 1.000000000000000000 ) ) 
 REPRESENTATION_ITEM ( '' )  );
#25138=VECTOR ( 'NONE', #32842, 1000.000000000000000 ) ;
#25139=DIRECTION ( 'NONE',  ( -1.000000000000000000, 0.000000000000000000, -2.958228394578794708E-31 ) ) ;
#25143=EDGE_LOOP ( 'NONE', ( #28574, #42154, #35649, #21669 ) ) ;
#25145=ORIENTED_EDGE ( 'NONE', *, *, #37116, .F. ) ;
#25148=ORIENTED_EDGE ( 'NONE', *, *, #48841, .F. ) ;
#25153=VERTEX_POINT ( 'NONE', #44680 ) ;
#25166=FACE_OUTER_BOUND ( 'NONE', #223, .T. ) ;
#25168=VECTOR ( 'NONE', #31902, 1000.000000000000000 ) ;
#25173=CARTESIAN_POINT ( 'NONE',  ( 341.9999999999999432, -181.0000000000001421, -356.0000000000003411 ) ) ;
#25174=ADVANCED_FACE ( 'NONE', ( #34887 ), #2360, .F. ) ;
#25177=VERTEX_POINT ( 'NONE', #21873 ) ;
#25179=AXIS2_PLACEMENT_3D ( 'NONE', #35922, #47404, #28956 ) ;
#25186=VERTEX_POINT ( 'NONE', #17998 ) ;
#25187=ORIENTED_EDGE ( 'NONE', *, *, #30567, .T. ) ;
#25191=CARTESIAN_POINT ( 'NONE',  ( 0.000000000000000000, -180.9999999999999716, -356.0000000000002274 ) ) ;
#25193=CARTESIAN_POINT ( 'NONE',  ( 181.0000000000000000, 10.00000000000006395, 339.9999999999998295 ) ) ;
#25201=EDGE_CURVE ( 'NONE', #15011, #40834, #33674, .T. ) ;
#25206=CARTESIAN_POINT ( 'NONE',  ( 356.0000000000001137, 167.0000000000000000, 349.9999999999998863 ) ) ;
#25212=EDGE_CURVE ( 'NONE', #7227, #27797, #15921, .T. ) ;
#25228=DIRECTION ( 'NONE',  ( 0.000000000000000000, -1.000000000000000000, -3.186989995019654210E-49 ) ) ;
#25232=AXIS2_PLACEMENT_3D ( 'NONE', #19843, #38613, #23956 ) ;
#25238=EDGE_CURVE ( 'NONE', #1115, #14362, #35146, .T. ) ;
#25242=ADVANCED_FACE ( 'NONE', ( #27175 ), #15618, .F. ) ;
#25245=VERTEX_POINT ( 'NONE', #20470 ) ;
#25251=CARTESIAN_POINT ( 'NONE',  ( 183.0000000000000284, -174.9999999999999716, -111.0000000000001563 ) ) ;
#25256=VERTEX_POINT ( 'NONE', #36148 ) ;
#25260=( BOUNDED_CURVE ( )  B_SPLINE_CURVE ( 3, ( #4170, #24184, #35486, #333 ),
 .UNSPECIFIED., .F., .F. ) 
 B_SPLINE_CURVE_WITH_KNOTS ( ( 4, 4 ),
 ( 1.570796326794896780, 3.141592653589793116 ),
 .UNSPECIFIED. ) 
 CURVE ( )  GEOMETRIC_REPRESENTATION_ITEM ( )  RATIONAL_B_SPLINE_CURVE ( ( 1.000000000000000000, 0.8047378541243650485, 0.8047378541243650485, 1.000000000000000000 ) ) 
 REPRESENTATION_ITEM ( '' )  );
#25261=DIRECTION ( 'NONE',  ( -4.485344387572531843E-16, -0.7071067811865476838, -0.7071067811865473507 ) ) ;
#25265=EDGE_LOOP ( 'NONE', ( #29979, #14259, #1018, #19133, #31911, #32021, #4746, #26943 ) ) ;
#25266=( BOUNDED_CURVE ( )  B_SPLINE_CURVE ( 3, ( #13892, #10064, #41111, #25719 ),
 .UNSPECIFIED., .F., .F. ) 
 B_SPLINE_CURVE_WITH_KNOTS ( ( 4, 4 ),
 ( 0.000000000000000000, 1.570796326794896558 ),
 .UNSPECIFIED. ) 
 CURVE ( )  GEOMETRIC_REPRESENTATION_ITEM ( )  RATIONAL_B_SPLINE_CURVE ( ( 1.000000000000000000, 0.8047378541243649375, 0.8047378541243649375, 1.000000000000000000 ) ) 
 REPRESENTATION_ITEM ( '' )  );
#25268=ORIENTED_EDGE ( 'NONE', *, *, #42860, .T. ) ;
#25272=VERTEX_POINT ( 'NONE', #32045 ) ;
#25285=VECTOR ( 'NONE', #32179, 1000.000000000000000 ) ;
#25289=FACE_OUTER_BOUND ( 'NONE', #1489, .T. ) ;
#25300=FACE_OUTER_BOUND ( 'NONE', #19701, .T. ) ;
#25303=PLANE ( 'NONE',  #22448 ) ;
#25306=CARTESIAN_POINT ( 'NONE',  ( 357.9999999999999432, -181.0000000000001421, -356.0000000000003979 ) ) ;
#25307=EDGE_CURVE ( 'NONE', #5304, #9422, #40237, .T. ) ;
#25308=DIRECTION ( 'NONE',  ( 0.000000000000000000, -2.537652627714643577E-15, -1.000000000000000000 ) ) ;
#25310=EDGE_LOOP ( 'NONE', ( #25579, #38470, #4651, #42961 ) ) ;
#25313=ORIENTED_EDGE ( 'NONE', *, *, #32601, .T. ) ;
#25314=VERTEX_POINT ( 'NONE', #20990 ) ;
#25339=CARTESIAN_POINT ( 'NONE',  ( 343.9999999999999432, -185.0000000000001421, -360.0000000000003979 ) ) ;
#25343=DIRECTION ( 'NONE',  ( 0.000000000000000000, 0.000000000000000000, 1.000000000000000000 ) ) ;
#25350=CARTESIAN_POINT ( 'NONE',  ( 181.0000000000000000, -272.4999999999999432, -359.9999999999999432 ) ) ;
#25353=EDGE_CURVE ( 'NONE', #16301, #7708, #41232, .T. ) ;
#25357=( BOUNDED_CURVE ( )  B_SPLINE_CURVE ( 3, ( #10290, #44896, #29790, #48734 ),
 .UNSPECIFIED., .F., .F. ) 
 B_SPLINE_CURVE_WITH_KNOTS ( ( 4, 4 ),
 ( 3.141592653589793116, 4.712388980384693227 ),
 .UNSPECIFIED. ) 
 CURVE ( )  GEOMETRIC_REPRESENTATION_ITEM ( )  RATIONAL_B_SPLINE_CURVE ( ( 1.000000000000000000, 0.8047378541243641603, 0.8047378541243641603, 1.000000000000000000 ) ) 
 REPRESENTATION_ITEM ( '' )  );
#25358=EDGE_LOOP ( 'NONE', ( #41970, #27995, #14308, #7735 ) ) ;
#25362=VECTOR ( 'NONE', #44557, 1000.000000000000000 ) ;
#25364=ORIENTED_EDGE ( 'NONE', *, *, #36811, .F. ) ;
#25368=ADVANCED_FACE ( 'NONE', ( #40493 ), #44813, .F. ) ;
#25378=EDGE_CURVE ( 'NONE', #20650, #15814, #28933, .T. ) ;
#25383=CARTESIAN_POINT ( 'NONE',  ( 350.0000000000000000, 169.0000000000000000, -360.0000000000002274 ) ) ;
#25385=DIRECTION ( 'NONE',  ( 0.000000000000000000, 3.186989995019654210E-49, 1.000000000000000000 ) ) ;
#25387=ORIENTED_EDGE ( 'NONE', *, *, #28836, .T. ) ;
#25388=VERTEX_POINT ( 'NONE', #25339 ) ;
#25390=DIRECTION ( 'NONE',  ( -0.000000000000000000, -1.000000000000000000, 2.537652627714643577E-15 ) ) ;
#25391=LINE ( 'NONE', #13075, #23408 ) ;
#25394=VECTOR ( 'NONE', #41251, 1000.000000000000000 ) ;
#25399=CARTESIAN_POINT ( 'NONE',  ( 4.999999999999999112, -175.0000000000000284, 350.0000000000002274 ) ) ;
#25406=EDGE_CURVE ( 'NONE', #28419, #3854, #31495, .T. ) ;
#25408=CIRCLE ( 'NONE', #3265, 3.749999999999975575 ) ;
#25410=DIRECTION ( 'NONE',  ( 0.000000000000000000, -1.000000000000000000, -3.186989995019654210E-49 ) ) ;
#25425=CARTESIAN_POINT ( 'NONE',  ( 358.3431457505076310, 165.0000000000000284, 339.9999999999997726 ) ) ;
#25427=AXIS2_PLACEMENT_3D ( 'NONE', #31767, #7912, #42520 ) ;
#25433=DIRECTION ( 'NONE',  ( -1.000000000000000000, 3.172065799423185948E-16, -1.587271980518778491E-16 ) ) ;
#25458=VERTEX_POINT ( 'NONE', #18878 ) ;
#25466=EDGE_CURVE ( 'NONE', #19947, #23987, #18630, .T. ) ;
#25479=CARTESIAN_POINT ( 'NONE',  ( 181.0000000000000284, -272.5000000000000000, -114.9999999999999147 ) ) ;
#25484=PLANE ( 'NONE',  #36072 ) ;
#25489=CARTESIAN_POINT ( 'NONE',  ( 166.9999999999999716, -268.5000000000000000, -339.9999999999998863 ) ) ;
#25492=ORIENTED_EDGE ( 'NONE', *, *, #15569, .T. ) ;
#25497=AXIS2_PLACEMENT_3D ( 'NONE', #17295, #13692, #1903 ) ;
#25501=DIRECTION ( 'NONE',  ( 1.000000000000000000, 0.000000000000000000, 2.958228394578794270E-31 ) ) ;
#25505=ORIENTED_EDGE ( 'NONE', *, *, #26298, .F. ) ;
#25514=ORIENTED_EDGE ( 'NONE', *, *, #38085, .F. ) ;
#25522=DIRECTION ( 'NONE',  ( 1.000000000000000000, -0.000000000000000000, 0.000000000000000000 ) ) ;
#25523=VERTEX_POINT ( 'NONE', #42489 ) ;
#25534=CIRCLE ( 'NONE', #48409, 2.000000000000001776 ) ;
#25539=CARTESIAN_POINT ( 'NONE',  ( 5.551115123125782702E-14, -168.9999999999999432, 343.9999999999997726 ) ) ;
#25544=AXIS2_PLACEMENT_3D ( 'NONE', #14949, #50296, #15207 ) ;
#25548=CARTESIAN_POINT ( 'NONE',  ( 350.0000000000001137, 165.0000000000000000, 355.9999999999997726 ) ) ;
#25561=( BOUNDED_CURVE ( )  B_SPLINE_CURVE ( 3, ( #47351, #32760, #16603, #9149 ),
 .UNSPECIFIED., .F., .F. ) 
 B_SPLINE_CURVE_WITH_KNOTS ( ( 4, 4 ),
 ( 0.000000000000000000, 1.570796326794931197 ),
 .UNSPECIFIED. ) 
 CURVE ( )  GEOMETRIC_REPRESENTATION_ITEM ( )  RATIONAL_B_SPLINE_CURVE ( ( 1.000000000000000000, 0.8047378541243568328, 0.8047378541243568328, 1.000000000000000000 ) ) 
 REPRESENTATION_ITEM ( '' )  );
#25566=VERTEX_POINT ( 'NONE', #42999 ) ;
#25569=VERTEX_POINT ( 'NONE', #50409 ) ;
#25575=FACE_OUTER_BOUND ( 'NONE', #24314, .T. ) ;
#25576=CIRCLE ( 'NONE', #42769, 4.000000000000003553 ) ;
#25579=ORIENTED_EDGE ( 'NONE', *, *, #27130, .T. ) ;
#25587=DIRECTION ( 'NONE',  ( -2.958228394578793832E-31, 0.000000000000000000, -1.000000000000000000 ) ) ;
#25597=EDGE_CURVE ( 'NONE', #18727, #10108, #40689, .T. ) ;
#25610=EDGE_LOOP ( 'NONE', ( #33350, #19190, #21747, #25505 ) ) ;
#25613=VECTOR ( 'NONE', #39622, 1000.000000000000000 ) ;
#25616=DIRECTION ( 'NONE',  ( -1.000000000000000000, 0.000000000000000000, -2.958228394578794270E-31 ) ) ;
#25632=EDGE_CURVE ( 'NONE', #50040, #50273, #36093, .T. ) ;
#25634=CIRCLE ( 'NONE', #20720, 4.000000000000003553 ) ;
#25635=CARTESIAN_POINT ( 'NONE',  ( 169.0000000000000284, 165.0000000000000000, 359.9999999999997726 ) ) ;
#25638=DIRECTION ( 'NONE',  ( 1.000000000000000000, 0.000000000000000000, 2.958228394578794270E-31 ) ) ;
#25641=DIRECTION ( 'NONE',  ( -7.793956916774525800E-48, 0.000000000000000000, -1.000000000000000000 ) ) ;
#25657=VECTOR ( 'NONE', #29327, 1000.000000000000000 ) ;
#25658=ORIENTED_EDGE ( 'NONE', *, *, #14350, .T. ) ;
#25659=LINE ( 'NONE', #13335, #1569 ) ;
#25661=EDGE_CURVE ( 'NONE', #38870, #31478, #33253, .T. ) ;
#25668=( BOUNDED_CURVE ( )  B_SPLINE_CURVE ( 3, ( #22756, #38428, #18891, #34570 ),
 .UNSPECIFIED., .F., .F. ) 
 B_SPLINE_CURVE_WITH_KNOTS ( ( 4, 4 ),
 ( 3.141592653589793560, 4.712388980384731418 ),
 .UNSPECIFIED. ) 
 CURVE ( )  GEOMETRIC_REPRESENTATION_ITEM ( )  RATIONAL_B_SPLINE_CURVE ( ( 1.000000000000000000, 0.8047378541243551675, 0.8047378541243551675, 1.000000000000000000 ) ) 
 REPRESENTATION_ITEM ( '' )  );
#25676=CARTESIAN_POINT ( 'NONE',  ( 0.000000000000000000, 165.0000000000000000, -344.0000000000001705 ) ) ;
#25678=CARTESIAN_POINT ( 'NONE',  ( 168.9999999999999716, -184.9999999999999716, -358.0000000000001705 ) ) ;
#25691=CARTESIAN_POINT ( 'NONE',  ( 168.9999999999999716, 10.00000000000006395, -340.0000000000001137 ) ) ;
#25697=ORIENTED_EDGE ( 'NONE', *, *, #8762, .T. ) ;
#25701=CARTESIAN_POINT ( 'NONE',  ( -5.000000000000000000, 184.8000000000000114, 340.1999999999997044 ) ) ;
#25703=ORIENTED_EDGE ( 'NONE', *, *, #28449, .T. ) ;
#25710=CARTESIAN_POINT ( 'NONE',  ( 341.6568542494922553, 185.0000000000002558, -360.0000000000003411 ) ) ;
#25714=AXIS2_PLACEMENT_3D ( 'NONE', #23666, #43656, #43407 ) ;
#25717=AXIS2_PLACEMENT_3D ( 'NONE', #17810, #1918, #33477 ) ;
#25719=CARTESIAN_POINT ( 'NONE',  ( 360.0000000000000000, -168.9999999999999432, 343.9999999999998295 ) ) ;
#25730=CYLINDRICAL_SURFACE ( 'NONE', #20100, 2.000000000000001776 ) ;
#25734=EDGE_CURVE ( 'NONE', #12204, #4741, #5776, .T. ) ;
#25751=CIRCLE ( 'NONE', #42947, 2.000000000000001776 ) ;
#25752=FACE_OUTER_BOUND ( 'NONE', #43804, .T. ) ;
#25754=ORIENTED_EDGE ( 'NONE', *, *, #30354, .F. ) ;
#25755=VERTEX_POINT ( 'NONE', #48074 ) ;
#25761=ORIENTED_EDGE ( 'NONE', *, *, #21424, .T. ) ;
#25765=ORIENTED_EDGE ( 'NONE', *, *, #13352, .F. ) ;
#25776=VERTEX_POINT ( 'NONE', #24287 ) ;
#25777=CARTESIAN_POINT ( 'NONE',  ( 341.9999999999999432, -169.0000000000001137, -349.9999999999998863 ) ) ;
#25778=VERTEX_POINT ( 'NONE', #20410 ) ;
#25779=CARTESIAN_POINT ( 'NONE',  ( 340.0000000000000568, 185.0000000000000284, 349.9999999999998295 ) ) ;
#25784=CARTESIAN_POINT ( 'NONE',  ( 183.0000000000000000, -174.9999999999999716, -356.0000000000001705 ) ) ;
#25786=VECTOR ( 'NONE', #6889, 1000.000000000000000 ) ;
#25788=ORIENTED_EDGE ( 'NONE', *, *, #6863, .F. ) ;
#25793=PLANE ( 'NONE',  #1206 ) ;
#25803=ORIENTED_EDGE ( 'NONE', *, *, #5184, .F. ) ;
#25807=AXIS2_PLACEMENT_3D ( 'NONE', #29332, #17780, #5716 ) ;
#25813=EDGE_CURVE ( 'NONE', #5419, #7227, #22687, .T. ) ;
#25814=ORIENTED_EDGE ( 'NONE', *, *, #9185, .T. ) ;
#25819=ORIENTED_EDGE ( 'NONE', *, *, #15761, .F. ) ;
#25822=VECTOR ( 'NONE', #23575, 1000.000000000000000 ) ;
#25823=ORIENTED_EDGE ( 'NONE', *, *, #49816, .T. ) ;
#25826=VECTOR ( 'NONE', #11526, 1000.000000000000000 ) ;
#25829=CARTESIAN_POINT ( 'NONE',  ( 357.9999999999999432, -181.0000000000001421, -349.9999999999999432 ) ) ;
#25843=DIRECTION ( 'NONE',  ( 0.000000000000000000, -0.000000000000000000, 1.000000000000000000 ) ) ;
#25845=DIRECTION ( 'NONE',  ( 0.000000000000000000, 1.000000000000000000, 7.004339610132985974E-48 ) ) ;
#25847=LINE ( 'NONE', #42491, #40580 ) ;
#25851=CARTESIAN_POINT ( 'NONE',  ( 168.9999999999999716, 175.0000000000000284, -342.0000000000001137 ) ) ;
#25857=FACE_BOUND ( 'NONE', #10003, .T. ) ;
#25865=ADVANCED_FACE ( 'NONE', ( #10392 ), #6532, .F. ) ;
#25866=EDGE_LOOP ( 'NONE', ( #1361, #9455, #274, #7961 ) ) ;
#25867=FACE_OUTER_BOUND ( 'NONE', #35709, .T. ) ;
#25868=FACE_OUTER_BOUND ( 'NONE', #9794, .T. ) ;
#25872=ORIENTED_EDGE ( 'NONE', *, *, #46859, .T. ) ;
#25878=CYLINDRICAL_SURFACE ( 'NONE', #31192, 2.000000000000001776 ) ;
#25879=EDGE_CURVE ( 'NONE', #12765, #8645, #14996, .T. ) ;
#25882=ORIENTED_EDGE ( 'NONE', *, *, #23703, .T. ) ;
#25883=DIRECTION ( 'NONE',  ( 1.000000000000000000, 0.000000000000000000, -1.586032892321652482E-16 ) ) ;
#25889=EDGE_CURVE ( 'NONE', #39539, #32832, #42682, .T. ) ;
#25892=DIRECTION ( 'NONE',  ( 0.000000000000000000, 0.000000000000000000, 1.000000000000000000 ) ) ;
#25893=VERTEX_POINT ( 'NONE', #30655 ) ;
#25901=ORIENTED_EDGE ( 'NONE', *, *, #5333, .F. ) ;
#25903=ORIENTED_EDGE ( 'NONE', *, *, #47261, .F. ) ;
#25905=DIRECTION ( 'NONE',  ( 0.000000000000000000, 1.000000000000000000, 7.004339610132985974E-48 ) ) ;
#25914=ADVANCED_FACE ( 'NONE', ( #35795 ), #19846, .F. ) ;
#25917=( LENGTH_UNIT ( ) NAMED_UNIT ( * ) SI_UNIT ( .MILLI., .METRE. ) );
#25922=VECTOR ( 'NONE', #9605, 1000.000000000000000 ) ;
#25925=AXIS2_PLACEMENT_3D ( 'NONE', #14138, #36774, #10054 ) ;
#25930=DIRECTION ( 'NONE',  ( 0.000000000000000000, 0.000000000000000000, -1.000000000000000000 ) ) ;
#25931=DIRECTION ( 'NONE',  ( 0.000000000000000000, -1.000000000000000000, 0.000000000000000000 ) ) ;
#25934=AXIS2_PLACEMENT_3D ( 'NONE', #37525, #32915, #21590 ) ;
#25936=CARTESIAN_POINT ( 'NONE',  ( 359.9999999999999432, -180.9999999999999716, 355.9999999999998295 ) ) ;
#25940=EDGE_CURVE ( 'NONE', #27545, #49709, #12534, .T. ) ;
#25948=ADVANCED_FACE ( 'NONE', ( #35276 ), #35527, .F. ) ;
#25949=ORIENTED_EDGE ( 'NONE', *, *, #13130, .F. ) ;
#25960=EDGE_CURVE ( 'NONE', #23178, #38152, #27045, .T. ) ;
#25961=ORIENTED_EDGE ( 'NONE', *, *, #14196, .F. ) ;
#25962=CIRCLE ( 'NONE', #18573, 2.000000000000001776 ) ;
#25964=CARTESIAN_POINT ( 'NONE',  ( 344.0000000000000568, 185.0000000000000284, 349.9999999999998295 ) ) ;
#25972=CARTESIAN_POINT ( 'NONE',  ( 339.9999999999999432, 183.3431457505078583, -358.3431457505080857 ) ) ;
#25974=EDGE_LOOP ( 'NONE', ( #640, #12734, #41477, #41964 ) ) ;
#25985=CARTESIAN_POINT ( 'NONE',  ( 168.9999999999999716, -7.999999999999952038, -350.0000000000001705 ) ) ;
#25986=FACE_OUTER_BOUND ( 'NONE', #46217, .T. ) ;
#25993=EDGE_CURVE ( 'NONE', #48807, #19760, #32173, .T. ) ;
#25994=FACE_OUTER_BOUND ( 'NONE', #29676, .T. ) ;
#25999=CARTESIAN_POINT ( 'NONE',  ( 185.0000000000000284, 2.775557561562891351E-14, -111.0000000000001563 ) ) ;
#26000=LINE ( 'NONE', #34722, #29046 ) ;
#26002=ORIENTED_EDGE ( 'NONE', *, *, #12856, .T. ) ;
#26009=LINE ( 'NONE', #5988, #23387 ) ;
#26011=ORIENTED_EDGE ( 'NONE', *, *, #45883, .T. ) ;
#26016=VERTEX_POINT ( 'NONE', #24727 ) ;
#26026=FACE_OUTER_BOUND ( 'NONE', #42990, .T. ) ;
#26029=VERTEX_POINT ( 'NONE', #31929 ) ;
#26031=CARTESIAN_POINT ( 'NONE',  ( 181.0000000000000284, -174.9999999999999716, -99.00000000000014211 ) ) ;
#26032=ORIENTED_EDGE ( 'NONE', *, *, #11274, .T. ) ;
#26033=DIRECTION ( 'NONE',  ( -1.000000000000000000, 3.172065745548403743E-16, -1.587271980518778491E-16 ) ) ;
#26039=DIRECTION ( 'NONE',  ( 1.000000000000000000, 0.000000000000000000, 0.000000000000000000 ) ) ;
#26059=DIRECTION ( 'NONE',  ( 1.000000000000000000, 0.000000000000000000, -0.000000000000000000 ) ) ;
#26062=EDGE_LOOP ( 'NONE', ( #17219, #35520, #47165, #34434 ) ) ;
#26078=ORIENTED_EDGE ( 'NONE', *, *, #21721, .F. ) ;
#26083=VERTEX_POINT ( 'NONE', #24980 ) ;
#26084=CARTESIAN_POINT ( 'NONE',  ( 5.551115123125782702E-14, -184.9999999999999716, 355.9999999999997726 ) ) ;
#26097=CARTESIAN_POINT ( 'NONE',  ( 181.0000000000000284, -9.999999999999953815, -113.0000000000001563 ) ) ;
#26099=LINE ( 'NONE', #42261, #50028 ) ;
#26100=VERTEX_POINT ( 'NONE', #9573 ) ;
#26105=DIRECTION ( 'NONE',  ( 0.000000000000000000, -0.7071067811865473507, 0.7071067811865475727 ) ) ;
#26106=DIRECTION ( 'NONE',  ( 1.000000000000000000, 0.000000000000000000, -1.586032892321652482E-16 ) ) ;
#26112=CARTESIAN_POINT ( 'NONE',  ( 360.0000000000000568, 166.6568542494923975, 341.6568542494921985 ) ) ;
#26116=ORIENTED_EDGE ( 'NONE', *, *, #28043, .F. ) ;
#26118=CARTESIAN_POINT ( 'NONE',  ( 359.9999999999999432, -181.0000000000001421, -356.0000000000003411 ) ) ;
#26120=VECTOR ( 'NONE', #4950, 1000.000000000000000 ) ;
#26121=VECTOR ( 'NONE', #12015, 1000.000000000000000 ) ;
#26129=CARTESIAN_POINT ( 'NONE',  ( 169.0000000000000000, -174.9999999999999716, -97.00000000000014211 ) ) ;
#26133=VERTEX_POINT ( 'NONE', #33687 ) ;
#26134=CARTESIAN_POINT ( 'NONE',  ( 344.0000000000000000, -167.0000000000001137, -349.9999999999998863 ) ) ;
#26135=DIRECTION ( 'NONE',  ( 0.000000000000000000, 0.000000000000000000, -1.000000000000000000 ) ) ;
#26139=CARTESIAN_POINT ( 'NONE',  ( 185.0000000000000000, -168.9999999999999432, -340.0000000000001137 ) ) ;
#26141=CARTESIAN_POINT ( 'NONE',  ( 342.8284271247460424, -183.0000000000001421, 358.0000000000001705 ) ) ;
#26143=ORIENTED_EDGE ( 'NONE', *, *, #10803, .T. ) ;
#26145=CARTESIAN_POINT ( 'NONE',  ( 181.0000000000000568, 165.0000000000000000, 357.9999999999998863 ) ) ;
#26151=( NAMED_UNIT ( * ) SI_UNIT ( $, .STERADIAN. ) SOLID_ANGLE_UNIT ( ) );
#26154=EDGE_CURVE ( 'NONE', #15166, #5729, #14170, .T. ) ;
#26158=DIRECTION ( 'NONE',  ( 1.587271980518778491E-16, -5.169878828456422968E-26, -1.000000000000000000 ) ) ;
#26170=CARTESIAN_POINT ( 'NONE',  ( 183.0000000000000000, -268.4999999999993747, -114.9999999999999147 ) ) ;
#26172=ADVANCED_FACE ( 'NONE', ( #10568 ), #5965, .F. ) ;
#26174=DIRECTION ( 'NONE',  ( 0.000000000000000000, 1.000000000000000000, 0.000000000000000000 ) ) ;
#26176=VERTEX_POINT ( 'NONE', #6979 ) ;
#26187=ADVANCED_FACE ( 'NONE', ( #49524 ), #10824, .T. ) ;
#26190=ORIENTED_EDGE ( 'NONE', *, *, #41700, .F. ) ;
#26192=CARTESIAN_POINT ( 'NONE',  ( 164.9999999999999716, 165.0000000000000000, -344.0000000000001137 ) ) ;
#26199=CIRCLE ( 'NONE', #42588, 4.000000000000003553 ) ;
#26202=VECTOR ( 'NONE', #6356, 1000.000000000000000 ) ;
#26205=LINE ( 'NONE', #42090, #39857 ) ;
#26206=LINE ( 'NONE', #42349, #17425 ) ;
#26216=VECTOR ( 'NONE', #30106, 1000.000000000000000 ) ;
#26219=EDGE_CURVE ( 'NONE', #25523, #48356, #6469, .T. ) ;
#26221=CARTESIAN_POINT ( 'NONE',  ( 168.9999999999999716, -182.9999999999999716, -350.0000000000001705 ) ) ;
#26223=ORIENTED_EDGE ( 'NONE', *, *, #25466, .F. ) ;
#26231=CARTESIAN_POINT ( 'NONE',  ( 165.0000000000000000, -168.9999999999999432, -115.0000000000001705 ) ) ;
#26235=CARTESIAN_POINT ( 'NONE',  ( 339.9999999999999432, -174.9999999999999432, 343.9999999999998295 ) ) ;
#26238=CARTESIAN_POINT ( 'NONE',  ( 181.0000000000000000, -164.9999999999999432, -344.0000000000001137 ) ) ;
#26244=DIRECTION ( 'NONE',  ( -1.000000000000000000, 0.000000000000000000, -2.958228394578794708E-31 ) ) ;
#26251=LINE ( 'NONE', #25999, #12313 ) ;
#26252=VECTOR ( 'NONE', #35954, 1000.000000000000000 ) ;
#26254=ORIENTED_EDGE ( 'NONE', *, *, #3585, .F. ) ;
#26261=CARTESIAN_POINT ( 'NONE',  ( 165.0000000000000000, 2.775557561562891351E-14, -111.0000000000001563 ) ) ;
#26263=EDGE_LOOP ( 'NONE', ( #18227, #49180, #20261, #31763 ) ) ;
#26273=FACE_OUTER_BOUND ( 'NONE', #31391, .T. ) ;
#26275=DIRECTION ( 'NONE',  ( 0.000000000000000000, 1.000000000000000000, -5.664403186863042467E-17 ) ) ;
#26279=ORIENTED_EDGE ( 'NONE', *, *, #8284, .T. ) ;
#26283=CARTESIAN_POINT ( 'NONE',  ( 357.1715728752538439, -166.9999999999999432, 341.9999999999998295 ) ) ;
#26284=VECTOR ( 'NONE', #8947, 1000.000000000000000 ) ;
#26287=CARTESIAN_POINT ( 'NONE',  ( 166.9999999999999716, -272.4999999999999432, -344.0000000000001137 ) ) ;
#26288=ORIENTED_EDGE ( 'NONE', *, *, #19588, .F. ) ;
#26289=DIRECTION ( 'NONE',  ( 0.000000000000000000, -2.537652627714643577E-15, -1.000000000000000000 ) ) ;
#26292=LINE ( 'NONE', #45998, #1557 ) ;
#26293=ADVANCED_FACE ( 'NONE', ( #30588 ), #4147, .F. ) ;
#26298=EDGE_CURVE ( 'NONE', #29620, #22392, #11335, .T. ) ;
#26302=EDGE_CURVE ( 'NONE', #36488, #1107, #20859, .T. ) ;
#26305=DIRECTION ( 'NONE',  ( 0.000000000000000000, 0.000000000000000000, 1.000000000000000000 ) ) ;
#26310=VECTOR ( 'NONE', #40656, 1000.000000000000000 ) ;
#26312=DIRECTION ( 'NONE',  ( -0.000000000000000000, 1.000000000000000000, 0.000000000000000000 ) ) ;
#26313=CARTESIAN_POINT ( 'NONE',  ( 181.0000000000000284, 2.775557561562891351E-14, -115.0000000000001563 ) ) ;
#26318=ORIENTED_EDGE ( 'NONE', *, *, #8064, .T. ) ;
#26333=CARTESIAN_POINT ( 'NONE',  ( 169.0000000000000000, -174.9999999999999716, -97.00000000000014211 ) ) ;
#26336=CYLINDRICAL_SURFACE ( 'NONE', #15304, 4.000000000000003553 ) ;
#26356=LINE ( 'NONE', #18634, #16662 ) ;
#26361=ORIENTED_EDGE ( 'NONE', *, *, #1064, .F. ) ;
#26364=DIRECTION ( 'NONE',  ( -1.000000000000000000, 0.000000000000000000, -1.612977847700450206E-50 ) ) ;
#26365=CARTESIAN_POINT ( 'NONE',  ( 0.000000000000000000, 0.000000000000000000, 0.000000000000000000 ) ) ;
#26366=VERTEX_POINT ( 'NONE', #45588 ) ;
#26367=CARTESIAN_POINT ( 'NONE',  ( 350.0000000000000000, -168.9999999999999432, -356.0000000000002274 ) ) ;
#26380=CARTESIAN_POINT ( 'NONE',  ( 168.9999999999999716, -81.49999999999997158, -350.0000000000001705 ) ) ;
#26384=ORIENTED_EDGE ( 'NONE', *, *, #9875, .T. ) ;
#26389=VERTEX_POINT ( 'NONE', #18154 ) ;
#26391=ORIENTED_EDGE ( 'NONE', *, *, #16276, .T. ) ;
#26392=ORIENTED_EDGE ( 'NONE', *, *, #24019, .F. ) ;
#26394=DIRECTION ( 'NONE',  ( 0.000000000000000000, 0.000000000000000000, 1.000000000000000000 ) ) ;
#26395=CARTESIAN_POINT ( 'NONE',  ( 341.9999999999998863, -182.1715728752539292, 357.1715728752539007 ) ) ;
#26406=ORIENTED_EDGE ( 'NONE', *, *, #31588, .F. ) ;
#26408=CARTESIAN_POINT ( 'NONE',  ( 168.9999999999999716, -164.9999999999999432, -356.0000000000001705 ) ) ;
#26418=ORIENTED_EDGE ( 'NONE', *, *, #24409, .F. ) ;
#26429=DIRECTION ( 'NONE',  ( -1.000000000000000000, 0.000000000000000000, 0.000000000000000000 ) ) ;
#26431=EDGE_CURVE ( 'NONE', #42347, #22458, #42199, .T. ) ;
#26434=PLANE ( 'NONE',  #47475 ) ;
#26435=FACE_OUTER_BOUND ( 'NONE', #42318, .T. ) ;
#26436=MECHANICAL_DESIGN_GEOMETRIC_PRESENTATION_REPRESENTATION('',(#45229),#19882);
#26440=CARTESIAN_POINT ( 'NONE',  ( 350.0000000000001137, 169.0000000000000000, 359.9999999999997726 ) ) ;
#26452=LINE ( 'NONE', #50510, #16619 ) ;
#26453=ORIENTED_EDGE ( 'NONE', *, *, #48497, .T. ) ;
#26470=ORIENTED_EDGE ( 'NONE', *, *, #27418, .T. ) ;
#26476=EDGE_CURVE ( 'NONE', #9422, #48932, #37191, .T. ) ;
#26478=VECTOR ( 'NONE', #43277, 1000.000000000000000 ) ;
#26479=CARTESIAN_POINT ( 'NONE',  ( 341.9999999999999432, 174.9999999999996589, -344.0000000000002842 ) ) ;
#26489=FACE_OUTER_BOUND ( 'NONE', #33178, .T. ) ;
#26491=AXIS2_PLACEMENT_3D ( 'NONE', #9007, #6162, #33626 ) ;
#26501=EDGE_CURVE ( 'NONE', #37542, #12765, #22267, .T. ) ;
#26505=ORIENTED_EDGE ( 'NONE', *, *, #26928, .F. ) ;
#26508=EDGE_CURVE ( 'NONE', #25153, #16301, #3257, .T. ) ;
#26514=AXIS2_PLACEMENT_3D ( 'NONE', #4850, #36179, #32328 ) ;
#26517=FACE_OUTER_BOUND ( 'NONE', #19958, .T. ) ;
#26519=VECTOR ( 'NONE', #37732, 1000.000000000000000 ) ;
#26522=LINE ( 'NONE', #11126, #18935 ) ;
#26523=VECTOR ( 'NONE', #7707, 1000.000000000000000 ) ;
#26527=ORIENTED_EDGE ( 'NONE', *, *, #27586, .T. ) ;
#26544=VERTEX_POINT ( 'NONE', #46840 ) ;
#26557=DIRECTION ( 'NONE',  ( 0.000000000000000000, 1.000000000000000000, 0.000000000000000000 ) ) ;
#26566=ORIENTED_EDGE ( 'NONE', *, *, #45015, .T. ) ;
#26569=AXIS2_PLACEMENT_3D ( 'NONE', #24350, #35901, #492 ) ;
#26573=CARTESIAN_POINT ( 'NONE',  ( 344.0000000000000000, 165.0000000000000000, -94.00000000000019895 ) ) ;
#26574=CARTESIAN_POINT ( 'NONE',  ( 343.9999999999994316, 183.0000000000000284, -358.0000000000001705 ) ) ;
#26589=ORIENTED_EDGE ( 'NONE', *, *, #1690, .F. ) ;
#26591=CARTESIAN_POINT ( 'NONE',  ( 167.0000000000000000, -9.999999999999953815, -99.00000000000014211 ) ) ;
#26602=DIRECTION ( 'NONE',  ( -1.000000000000000000, 0.000000000000000000, -1.612977847700450206E-50 ) ) ;
#26611=AXIS2_PLACEMENT_3D ( 'NONE', #10512, #26174, #29769 ) ;
#26617=ORIENTED_EDGE ( 'NONE', *, *, #933, .T. ) ;
#26619=CARTESIAN_POINT ( 'NONE',  ( 340.0000000000000568, 183.0000000000000284, 343.9999999999997726 ) ) ;
#26620=VECTOR ( 'NONE', #34283, 1000.000000000000000 ) ;
#26630=AXIS2_PLACEMENT_3D ( 'NONE', #17570, #21931, #41676 ) ;
#26632=EDGE_CURVE ( 'NONE', #2845, #18735, #27389, .T. ) ;
#26634=EDGE_LOOP ( 'NONE', ( #23645, #16066, #23880, #8074 ) ) ;
#26637=CARTESIAN_POINT ( 'NONE',  ( 165.0000000000000284, 175.0000000000000284, 355.9999999999998863 ) ) ;
#26642=FACE_OUTER_BOUND ( 'NONE', #24560, .T. ) ;
#26645=EDGE_CURVE ( 'NONE', #10986, #42541, #28404, .T. ) ;
#26647=VECTOR ( 'NONE', #12742, 1000.000000000000000 ) ;
#26651=ORIENTED_EDGE ( 'NONE', *, *, #47726, .T. ) ;
#26653=ORIENTED_EDGE ( 'NONE', *, *, #18249, .T. ) ;
#26655=DIRECTION ( 'NONE',  ( 1.000000000000000000, 0.000000000000000000, 7.793956916774525800E-48 ) ) ;
#26662=CARTESIAN_POINT ( 'NONE',  ( 344.0000000000000000, -165.0000000000001137, -340.0000000000003411 ) ) ;
#26663=CARTESIAN_POINT ( 'NONE',  ( 340.0000000000000000, 165.0000000000000000, -106.0000000000001990 ) ) ;
#26664=AXIS2_PLACEMENT_3D ( 'NONE', #18071, #26289, #22934 ) ;
#26665=AXIS2_PLACEMENT_3D ( 'NONE', #20219, #3808, #47369 ) ;
#26674=LINE ( 'NONE', #42315, #38847 ) ;
#26676=ORIENTED_EDGE ( 'NONE', *, *, #30989, .F. ) ;
#26684=AXIS2_PLACEMENT_3D ( 'NONE', #24190, #36248, #20323 ) ;
#26695=ORIENTED_EDGE ( 'NONE', *, *, #23688, .F. ) ;
#26706=ORIENTED_EDGE ( 'NONE', *, *, #13026, .T. ) ;
#26708=AXIS2_PLACEMENT_3D ( 'NONE', #38932, #39185, #30718 ) ;
#26712=DIRECTION ( 'NONE',  ( -1.000000000000000000, 0.000000000000000000, 0.000000000000000000 ) ) ;
#26721=CARTESIAN_POINT ( 'NONE',  ( 339.9999999999999432, -180.9999999999999716, -358.0000000000002274 ) ) ;
#26722=DIRECTION ( 'NONE',  ( -3.364279341222521245E-16, -0.7071067811865474617, 0.7071067811865476838 ) ) ;
#26727=LINE ( 'NONE', #3358, #29433 ) ;
#26733=ORIENTED_EDGE ( 'NONE', *, *, #7078, .F. ) ;
#26735=LINE ( 'NONE', #42367, #49835 ) ;
#26736=VECTOR ( 'NONE', #11058, 1000.000000000000000 ) ;
#26740=( GEOMETRIC_REPRESENTATION_CONTEXT ( 3 ) GLOBAL_UNCERTAINTY_ASSIGNED_CONTEXT ( ( #996 ) ) GLOBAL_UNIT_ASSIGNED_CONTEXT ( ( #25917, #30018, #26151 ) ) REPRESENTATION_CONTEXT ( 'NONE', 'WORKASPACE' ) );
#26745=VECTOR ( 'NONE', #34996, 1000.000000000000000 ) ;
#26751=CARTESIAN_POINT ( 'NONE',  ( 164.9999999999999716, -272.5000000000000000, -99.00000000000014211 ) ) ;
#26759=MECHANICAL_DESIGN_GEOMETRIC_PRESENTATION_REPRESENTATION('',(#15308),#39894);
#26769=ORIENTED_EDGE ( 'NONE', *, *, #12063, .F. ) ;
#26770=FACE_OUTER_BOUND ( 'NONE', #39820, .T. ) ;
#26771=DIRECTION ( 'NONE',  ( 1.000000000000000000, -4.758098676964957447E-16, 2.958228394578795584E-31 ) ) ;
#26775=EDGE_CURVE ( 'NONE', #29100, #2097, #19735, .T. ) ;
#26780=CIRCLE ( 'NONE', #7111, 4.000000000000003553 ) ;
#26784=ORIENTED_EDGE ( 'NONE', *, *, #29028, .T. ) ;
#26793=ORIENTED_EDGE ( 'NONE', *, *, #3883, .F. ) ;
#26798=AXIS2_PLACEMENT_3D ( 'NONE', #6894, #8169, #31269 ) ;
#26803=DIRECTION ( 'NONE',  ( -1.000000000000000000, 7.930164457481157120E-16, -1.587271980518778491E-16 ) ) ;
#26805=EDGE_CURVE ( 'NONE', #18208, #3827, #16340, .T. ) ;
#26812=ORIENTED_EDGE ( 'NONE', *, *, #32471, .F. ) ;
#26819=CARTESIAN_POINT ( 'NONE',  ( 357.9999999999999432, -174.9999999999999716, 355.9999999999998295 ) ) ;
#26824=ADVANCED_FACE ( 'NONE', ( #25300 ), #18097, .T. ) ;
#26838=DIRECTION ( 'NONE',  ( 3.172065745548403743E-16, 1.000000000000000000, 0.000000000000000000 ) ) ;
#26844=DIRECTION ( 'NONE',  ( 0.000000000000000000, 0.000000000000000000, 1.000000000000000000 ) ) ;
#26847=VERTEX_POINT ( 'NONE', #5801 ) ;
#26848=LINE ( 'NONE', #27624, #37322 ) ;
#26856=DIRECTION ( 'NONE',  ( 0.000000000000000000, -0.000000000000000000, 1.000000000000000000 ) ) ;
#26861=FACE_OUTER_BOUND ( 'NONE', #29112, .T. ) ;
#26867=ADVANCED_FACE ( 'NONE', ( #29159 ), #44518, .F. ) ;
#26868=EDGE_CURVE ( 'NONE', #9910, #980, #33275, .T. ) ;
#26871=CARTESIAN_POINT ( 'NONE',  ( 341.6568542494924827, 185.0000000000000568, 359.9999999999998295 ) ) ;
#26872=ORIENTED_EDGE ( 'NONE', *, *, #20315, .F. ) ;
#26873=LINE ( 'NONE', #49668, #38636 ) ;
#26874=CARTESIAN_POINT ( 'NONE',  ( 355.9999999999999432, 183.0000000000002558, -358.0000000000003411 ) ) ;
#26889=DIRECTION ( 'NONE',  ( -1.000000000000000000, 0.000000000000000000, 0.000000000000000000 ) ) ;
#26890=CARTESIAN_POINT ( 'NONE',  ( 168.9999999999999716, -272.4999999999999432, -339.9999999999998863 ) ) ;
#26892=EDGE_LOOP ( 'NONE', ( #35877, #41877, #41031, #30477, #33195, #44038, #153, #45048 ) ) ;
#26896=EDGE_LOOP ( 'NONE', ( #12813, #7535, #49159, #19399 ) ) ;
#26906=CARTESIAN_POINT ( 'NONE',  ( 168.9999999999999716, -272.4999999999999432, -357.9999999999999432 ) ) ;
#26917=ADVANCED_FACE ( 'NONE', ( #15520 ), #50622, .T. ) ;
#26918=EDGE_CURVE ( 'NONE', #50401, #26389, #49606, .T. ) ;
#26919=DIRECTION ( 'NONE',  ( -1.000000000000000000, 0.000000000000000000, -2.958228394578794270E-31 ) ) ;
#26921=CARTESIAN_POINT ( 'NONE',  ( 344.0000000000000568, 181.0000000000000284, 349.9999999999998295 ) ) ;
#26922=FACE_OUTER_BOUND ( 'NONE', #31816, .T. ) ;
#26923=( BOUNDED_CURVE ( )  B_SPLINE_CURVE ( 3, ( #41967, #20513, #44583, #21516 ),
 .UNSPECIFIED., .F., .F. ) 
 B_SPLINE_CURVE_WITH_KNOTS ( ( 4, 4 ),
 ( 3.141592653589793116, 4.712388980384703885 ),
 .UNSPECIFIED. ) 
 CURVE ( )  GEOMETRIC_REPRESENTATION_ITEM ( )  RATIONAL_B_SPLINE_CURVE ( ( 1.000000000000000000, 0.8047378541243617178, 0.8047378541243617178, 1.000000000000000000 ) ) 
 REPRESENTATION_ITEM ( '' )  );
#26924=ADVANCED_FACE ( 'NONE', ( #30158, #38379 ), #46771, .T. ) ;
#26928=EDGE_CURVE ( 'NONE', #36302, #31660, #7840, .T. ) ;
#26930=ORIENTED_EDGE ( 'NONE', *, *, #25813, .F. ) ;
#26934=CARTESIAN_POINT ( 'NONE',  ( 339.9999999999999432, 165.0000000000000000, -344.0000000000001705 ) ) ;
#26937=DIRECTION ( 'NONE',  ( 0.000000000000000000, 0.000000000000000000, -1.000000000000000000 ) ) ;
#26943=ORIENTED_EDGE ( 'NONE', *, *, #12596, .T. ) ;
#26951=VERTEX_POINT ( 'NONE', #38633 ) ;
#26952=DIRECTION ( 'NONE',  ( 0.000000000000000000, -2.265761274745217480E-16, 1.000000000000000000 ) ) ;
#26957=VERTEX_POINT ( 'NONE', #3449 ) ;
#26963=DIRECTION ( 'NONE',  ( 0.000000000000000000, 1.000000000000000000, 6.123233995736766036E-17 ) ) ;
#26973=CARTESIAN_POINT ( 'NONE',  ( 168.9999999999999716, -79.49999999999997158, -350.0000000000001705 ) ) ;
#26977=ORIENTED_EDGE ( 'NONE', *, *, #5796, .F. ) ;
#26979=LINE ( 'NONE', #43376, #4013 ) ;
#26991=LINE ( 'NONE', #16214, #43362 ) ;
#26993=VERTEX_POINT ( 'NONE', #2945 ) ;
#26998=VECTOR ( 'NONE', #19488, 1000.000000000000000 ) ;
#27000=AXIS2_PLACEMENT_3D ( 'NONE', #24174, #9017, #28268 ) ;
#27001=AXIS2_PLACEMENT_3D ( 'NONE', #890, #40137, #40639 ) ;
#27010=ORIENTED_EDGE ( 'NONE', *, *, #17678, .F. ) ;
#27014=CIRCLE ( 'NONE', #8167, 4.000000000000003553 ) ;
#27016=ORIENTED_EDGE ( 'NONE', *, *, #46512, .F. ) ;
#27029=ORIENTED_EDGE ( 'NONE', *, *, #32201, .F. ) ;
#27034=VECTOR ( 'NONE', #6433, 1000.000000000000000 ) ;
#27037=VECTOR ( 'NONE', #12541, 1000.000000000000000 ) ;
#27040=DIRECTION ( 'NONE',  ( 7.793956916774525800E-48, 0.000000000000000000, 1.000000000000000000 ) ) ;
#27043=CARTESIAN_POINT ( 'NONE',  ( 355.9999999999999432, -165.0000000000001137, -106.0000000000001990 ) ) ;
#27045=LINE ( 'NONE', #3694, #2033 ) ;
#27051=CARTESIAN_POINT ( 'NONE',  ( 355.9999999999999432, -185.0000000000000284, 359.9999999999998295 ) ) ;
#27052=DIRECTION ( 'NONE',  ( -0.000000000000000000, -0.000000000000000000, 1.000000000000000000 ) ) ;
#27058=CARTESIAN_POINT ( 'NONE',  ( 358.0000000000000568, -3.000000000000197176, -178.0000000000003979 ) ) ;
#27059=FACE_OUTER_BOUND ( 'NONE', #49169, .T. ) ;
#27065=LINE ( 'NONE', #35051, #22065 ) ;
#27071=ORIENTED_EDGE ( 'NONE', *, *, #29090, .F. ) ;
#27082=VERTEX_POINT ( 'NONE', #12677 ) ;
#27085=AXIS2_PLACEMENT_3D ( 'NONE', #17057, #16812, #29809 ) ;
#27090=CARTESIAN_POINT ( 'NONE',  ( 181.0000000000000000, -77.49999999999997158, -350.0000000000001705 ) ) ;
#27091=ADVANCED_FACE ( 'NONE', ( #39640 ), #39400, .T. ) ;
#27092=VERTEX_POINT ( 'NONE', #24244 ) ;
#27094=CARTESIAN_POINT ( 'NONE',  ( 357.1715728752542418, 167.0000000000003411, 342.0000000000001137 ) ) ;
#27103=LINE ( 'NONE', #42727, #12575 ) ;
#27106=VERTEX_POINT ( 'NONE', #16037 ) ;
#27109=DIRECTION ( 'NONE',  ( 1.333906992743555050E-23, -1.000000000000000000, 0.000000000000000000 ) ) ;
#27110=ORIENTED_EDGE ( 'NONE', *, *, #3537, .F. ) ;
#27111=DIRECTION ( 'NONE',  ( 0.000000000000000000, 1.000000000000000000, 0.000000000000000000 ) ) ;
#27113=CARTESIAN_POINT ( 'NONE',  ( 357.9999999999999432, -181.0000000000000568, -356.0000000000002842 ) ) ;
#27122=EDGE_CURVE ( 'NONE', #9291, #33463, #19867, .T. ) ;
#27128=VECTOR ( 'NONE', #49098, 1000.000000000000000 ) ;
#27130=EDGE_CURVE ( 'NONE', #28471, #39841, #39903, .T. ) ;
#27131=ORIENTED_EDGE ( 'NONE', *, *, #50234, .F. ) ;
#27134=ORIENTED_EDGE ( 'NONE', *, *, #38022, .F. ) ;
#27139=VERTEX_POINT ( 'NONE', #20125 ) ;
#27140=CARTESIAN_POINT ( 'NONE',  ( 4.999999999999999112, -175.0000000000000284, 353.7500000000001705 ) ) ;
#27142=VERTEX_POINT ( 'NONE', #35816 ) ;
#27143=EDGE_CURVE ( 'NONE', #46256, #5374, #4733, .T. ) ;
#27148=CARTESIAN_POINT ( 'NONE',  ( 181.0000000000000284, -174.9999999999999716, -97.00000000000014211 ) ) ;
#27151=CARTESIAN_POINT ( 'NONE',  ( 168.9999999999999716, -81.49999999999997158, -340.0000000000001137 ) ) ;
#27158=DIRECTION ( 'NONE',  ( -1.000000000000000000, 0.000000000000000000, -2.958228394578794270E-31 ) ) ;
#27164=AXIS2_PLACEMENT_3D ( 'NONE', #47075, #432, #8386 ) ;
#27172=CARTESIAN_POINT ( 'NONE',  ( 165.0000000000000000, -174.9999999999999716, -111.0000000000001563 ) ) ;
#27174=FACE_OUTER_BOUND ( 'NONE', #29374, .T. ) ;
#27175=FACE_OUTER_BOUND ( 'NONE', #16686, .T. ) ;
#27181=DIRECTION ( 'NONE',  ( 0.000000000000000000, 1.000000000000000000, 4.687818848539279227E-49 ) ) ;
#27182=EDGE_CURVE ( 'NONE', #33773, #27818, #26009, .T. ) ;
#27183=DIRECTION ( 'NONE',  ( 1.121065046350011585E-16, 0.7071067811865475727, 0.7071067811865474617 ) ) ;
#27185=EDGE_LOOP ( 'NONE', ( #50504, #8759, #35166, #8142 ) ) ;
#27186=CYLINDRICAL_SURFACE ( 'NONE', #8332, 2.000000000000001776 ) ;
#27189=AXIS2_PLACEMENT_3D ( 'NONE', #20159, #11454, #27111 ) ;
#27199=FACE_OUTER_BOUND ( 'NONE', #18986, .T. ) ;
#27203=( NAMED_UNIT ( * ) PLANE_ANGLE_UNIT ( ) SI_UNIT ( $, .RADIAN. ) );
#27208=ORIENTED_EDGE ( 'NONE', *, *, #33534, .F. ) ;
#27210=DIRECTION ( 'NONE',  ( -1.000000000000000000, 0.000000000000000000, 1.860490536778032451E-50 ) ) ;
#27211=LINE ( 'NONE', #20515, #2766 ) ;
#27217=ORIENTED_EDGE ( 'NONE', *, *, #8134, .F. ) ;
#27226=CARTESIAN_POINT ( 'NONE',  ( 355.9999999999999432, -181.0000000000001421, -349.9999999999999432 ) ) ;
#27229=DIRECTION ( 'NONE',  ( -1.000000000000000000, 4.996003610813203446E-16, -1.033975765691284410E-24 ) ) ;
#27242=EDGE_LOOP ( 'NONE', ( #8487, #48988, #47337, #49767 ) ) ;
#27244=LINE ( 'NONE', #38797, #47398 ) ;
#27245=DIRECTION ( 'NONE',  ( -1.000000000000000000, 1.586032892321652236E-16, 9.711650524620651178E-33 ) ) ;
#27251=LINE ( 'NONE', #19529, #36810 ) ;
#27263=DIRECTION ( 'NONE',  ( 0.000000000000000000, 0.000000000000000000, -1.000000000000000000 ) ) ;
#27268=CIRCLE ( 'NONE', #23149, 2.000000000000001776 ) ;
#27286=CARTESIAN_POINT ( 'NONE',  ( -5.000000000000000000, -184.7999999999999545, -340.2000000000001592 ) ) ;
#27287=DIRECTION ( 'NONE',  ( -1.000000000000000000, 0.000000000000000000, 1.860490536778032451E-50 ) ) ;
#27290=CARTESIAN_POINT ( 'NONE',  ( 181.0000000000000000, -272.5000000000000000, -112.9999999999999005 ) ) ;
#27291=VERTEX_POINT ( 'NONE', #38067 ) ;
#27293=ORIENTED_EDGE ( 'NONE', *, *, #44019, .F. ) ;
#27294=DIRECTION ( 'NONE',  ( 4.440892098500625176E-16, 0.7071067811865474617, 0.7071067811865475727 ) ) ;
#27295=ADVANCED_FACE ( 'NONE', ( #10596 ), #7520, .T. ) ;
#27296=CARTESIAN_POINT ( 'NONE',  ( 168.9999999999999716, -164.9999999999999432, 343.9999999999998863 ) ) ;
#27298=CARTESIAN_POINT ( 'NONE',  ( 356.0000000000000000, -174.9999999999999432, 341.9999999999998295 ) ) ;
#27301=ORIENTED_EDGE ( 'NONE', *, *, #34048, .T. ) ;
#27302=AXIS2_PLACEMENT_3D ( 'NONE', #25548, #13739, #9644 ) ;
#27303=EDGE_LOOP ( 'NONE', ( #32356, #48547, #39481, #42040 ) ) ;
#27304=CARTESIAN_POINT ( 'NONE',  ( 356.0000000000000000, 185.0000000000000284, -360.0000000000002274 ) ) ;
#27307=VECTOR ( 'NONE', #742, 1000.000000000000000 ) ;
#27309=ORIENTED_EDGE ( 'NONE', *, *, #10302, .F. ) ;
#27316=( BOUNDED_CURVE ( )  B_SPLINE_CURVE ( 3, ( #18272, #38571, #14948, #30603 ),
 .UNSPECIFIED., .F., .F. ) 
 B_SPLINE_CURVE_WITH_KNOTS ( ( 4, 4 ),
 ( 4.712388980384669246, 6.283185307179586232 ),
 .UNSPECIFIED. ) 
 CURVE ( )  GEOMETRIC_REPRESENTATION_ITEM ( )  RATIONAL_B_SPLINE_CURVE ( ( 1.000000000000000000, 0.8047378541243601635, 0.8047378541243601635, 1.000000000000000000 ) ) 
 REPRESENTATION_ITEM ( '' )  );
#27319=DIRECTION ( 'NONE',  ( 1.000000000000000000, -1.586032892321652236E-16, -9.711650524620651178E-33 ) ) ;
#27321=EDGE_CURVE ( 'NONE', #38840, #17911, #34469, .T. ) ;
#27326=CARTESIAN_POINT ( 'NONE',  ( 181.0000000000000000, -7.999999999999952038, -350.0000000000001705 ) ) ;
#27335=DIRECTION ( 'NONE',  ( 1.333906992743555050E-23, -1.000000000000000000, 0.000000000000000000 ) ) ;
#27346=DIRECTION ( 'NONE',  ( -7.793956916774525800E-48, 0.000000000000000000, 1.000000000000000000 ) ) ;
#27347=CYLINDRICAL_SURFACE ( 'NONE', #5281, 2.000000000000001776 ) ;
#27351=DIRECTION ( 'NONE',  ( -1.586032892321652236E-16, -1.000000000000000000, -6.853681917100419162E-49 ) ) ;
#27358=ORIENTED_EDGE ( 'NONE', *, *, #38085, .T. ) ;
#27363=ORIENTED_EDGE ( 'NONE', *, *, #30339, .F. ) ;
#27364=AXIS2_PLACEMENT_3D ( 'NONE', #7369, #38676, #33732 ) ;
#27367=CARTESIAN_POINT ( 'NONE',  ( 341.6568542494922553, -185.0000000000000853, -360.0000000000003411 ) ) ;
#27373=( BOUNDED_CURVE ( )  B_SPLINE_CURVE ( 3, ( #473, #16116, #31778, #24075 ),
 .UNSPECIFIED., .F., .F. ) 
 B_SPLINE_CURVE_WITH_KNOTS ( ( 4, 4 ),
 ( 6.280369834735098695E-16, 1.570796326794897002 ),
 .UNSPECIFIED. ) 
 CURVE ( )  GEOMETRIC_REPRESENTATION_ITEM ( )  RATIONAL_B_SPLINE_CURVE ( ( 1.000000000000000000, 0.8047378541243650485, 0.8047378541243650485, 1.000000000000000000 ) ) 
 REPRESENTATION_ITEM ( '' )  );
#27374=ORIENTED_EDGE ( 'NONE', *, *, #18686, .T. ) ;
#27380=CARTESIAN_POINT ( 'NONE',  ( 181.0000000000000284, -174.9999999999999716, -97.00000000000014211 ) ) ;
#27383=LINE ( 'NONE', #12474, #20734 ) ;
#27389=LINE ( 'NONE', #28640, #26647 ) ;
#27390=ORIENTED_EDGE ( 'NONE', *, *, #18991, .F. ) ;
#27394=CARTESIAN_POINT ( 'NONE',  ( 164.9999999999999716, -5.999999999999950262, -350.0000000000001705 ) ) ;
#27397=CARTESIAN_POINT ( 'NONE',  ( 181.0000000000000568, 175.0000000000000284, 339.9999999999998863 ) ) ;
#27401=CARTESIAN_POINT ( 'NONE',  ( 360.0000000000001137, 178.0000000000000284, 352.9999999999998295 ) ) ;
#27403=ORIENTED_EDGE ( 'NONE', *, *, #24063, .F. ) ;
#27405=CYLINDRICAL_SURFACE ( 'NONE', #9409, 4.000000000000003553 ) ;
#27408=ADVANCED_FACE ( 'NONE', ( #34218 ), #15217, .F. ) ;
#27410=DIRECTION ( 'NONE',  ( 0.000000000000000000, -1.000000000000000000, 2.537652627714643577E-15 ) ) ;
#27412=ORIENTED_EDGE ( 'NONE', *, *, #15569, .F. ) ;
#27418=EDGE_CURVE ( 'NONE', #2035, #29662, #35491, .T. ) ;
#27432=AXIS2_PLACEMENT_3D ( 'NONE', #27151, #42777, #38705 ) ;
#27435=ORIENTED_EDGE ( 'NONE', *, *, #26508, .T. ) ;
#27436=DIRECTION ( 'NONE',  ( -1.586032892321652482E-16, 0.000000000000000000, -1.000000000000000000 ) ) ;
#27457=ORIENTED_EDGE ( 'NONE', *, *, #41675, .F. ) ;
#27462=CIRCLE ( 'NONE', #2040, 4.000000000000003553 ) ;
#27466=DIRECTION ( 'NONE',  ( 0.000000000000000000, -1.000000000000000000, 0.000000000000000000 ) ) ;
#27467=EDGE_LOOP ( 'NONE', ( #39829, #5095, #14845, #32212 ) ) ;
#27473=ADVANCED_FACE ( 'NONE', ( #27775 ), #4425, .F. ) ;
#27476=DIRECTION ( 'NONE',  ( 0.000000000000000000, 0.000000000000000000, 1.000000000000000000 ) ) ;
#27479=DIRECTION ( 'NONE',  ( 0.000000000000000000, -2.265761274745217480E-16, 1.000000000000000000 ) ) ;
#27481=AXIS2_PLACEMENT_3D ( 'NONE', #10066, #24973, #13663 ) ;
#27489=EDGE_CURVE ( 'NONE', #1426, #25177, #19552, .T. ) ;
#27507=AXIS2_PLACEMENT_3D ( 'NONE', #39216, #4054, #216 ) ;
#27511=ADVANCED_FACE ( 'NONE', ( #20821 ), #9034, .T. ) ;
#27519=CARTESIAN_POINT ( 'NONE',  ( 350.0000000000000000, -184.9999999999999716, -344.0000000000001705 ) ) ;
#27521=VECTOR ( 'NONE', #14028, 1000.000000000000000 ) ;
#27528=DIRECTION ( 'NONE',  ( 0.000000000000000000, -1.000000000000000000, -1.544785076050074834E-48 ) ) ;
#27530=CARTESIAN_POINT ( 'NONE',  ( 181.0000000000000000, -95.49999999999997158, -115.0000000000001563 ) ) ;
#27540=VERTEX_POINT ( 'NONE', #28783 ) ;
#27545=VERTEX_POINT ( 'NONE', #44407 ) ;
#27547=ORIENTED_EDGE ( 'NONE', *, *, #26805, .T. ) ;
#27550=DIRECTION ( 'NONE',  ( 1.000000000000000000, 0.000000000000000000, 0.000000000000000000 ) ) ;
#27552=AXIS2_PLACEMENT_3D ( 'NONE', #10172, #29927, #2470 ) ;
#27563=VECTOR ( 'NONE', #280, 1000.000000000000000 ) ;
#27567=DIRECTION ( 'NONE',  ( 1.000000000000000000, -0.000000000000000000, 1.860490536778032451E-50 ) ) ;
#27569=CARTESIAN_POINT ( 'NONE',  ( 181.0000000000000284, -174.9999999999999716, -111.0000000000001563 ) ) ;
#27571=CARTESIAN_POINT ( 'NONE',  ( 344.0000000000000000, -165.0000000000001137, -340.0000000000003411 ) ) ;
#27586=EDGE_CURVE ( 'NONE', #6873, #37811, #33158, .T. ) ;
#27589=CIRCLE ( 'NONE', #18545, 2.000000000000001776 ) ;
#27591=VECTOR ( 'NONE', #29688, 1000.000000000000000 ) ;
#27592=DIRECTION ( 'NONE',  ( 0.000000000000000000, -1.000000000000000000, 3.469446951953611033E-15 ) ) ;
#27593=EDGE_CURVE ( 'NONE', #41767, #22392, #38206, .T. ) ;
#27598=VECTOR ( 'NONE', #34412, 1000.000000000000000 ) ;
#27599=DIRECTION ( 'NONE',  ( 1.000000000000000000, 0.000000000000000000, 0.000000000000000000 ) ) ;
#27601=ORIENTED_EDGE ( 'NONE', *, *, #3763, .F. ) ;
#27605=DIRECTION ( 'NONE',  ( -1.586032892321652236E-16, -1.000000000000000000, -2.288264760618012091E-48 ) ) ;
#27608=VERTEX_POINT ( 'NONE', #32639 ) ;
#27610=ORIENTED_EDGE ( 'NONE', *, *, #46137, .F. ) ;
#27620=LINE ( 'NONE', #43248, #6020 ) ;
#27624=CARTESIAN_POINT ( 'NONE',  ( 165.0000000000000000, -174.9999999999999716, -115.0000000000001563 ) ) ;
#27637=CARTESIAN_POINT ( 'NONE',  ( 166.9999999999999716, -272.5000000000000000, -98.99999999999874944 ) ) ;
#27646=EDGE_CURVE ( 'NONE', #25388, #19871, #33406, .T. ) ;
#27647=CARTESIAN_POINT ( 'NONE',  ( 339.9999999999999432, 174.9999999999996589, -344.0000000000002842 ) ) ;
#27655=CARTESIAN_POINT ( 'NONE',  ( 356.0000000000001137, 165.0000000000000000, 349.9999999999998295 ) ) ;
#27656=CARTESIAN_POINT ( 'NONE',  ( 350.0000000000000000, 183.0000000000000284, -344.0000000000001705 ) ) ;
#27659=FACE_OUTER_BOUND ( 'NONE', #11622, .T. ) ;
#27662=CARTESIAN_POINT ( 'NONE',  ( 358.0000000000000000, -169.0000000000001137, -344.0000000000002842 ) ) ;
#27668=DIRECTION ( 'NONE',  ( 0.000000000000000000, -1.000000000000000000, -3.186989995019654210E-49 ) ) ;
#27671=CYLINDRICAL_SURFACE ( 'NONE', #33618, 2.000000000000001776 ) ;
#27674=FACE_OUTER_BOUND ( 'NONE', #24738, .T. ) ;
#27676=AXIS2_PLACEMENT_3D ( 'NONE', #44003, #39434, #8627 ) ;
#27688=CARTESIAN_POINT ( 'NONE',  ( 350.0000000000000000, -180.9999999999999716, -358.0000000000002274 ) ) ;
#27690=CARTESIAN_POINT ( 'NONE',  ( 168.9999999999999716, 8.000000000000062172, 339.9999999999998295 ) ) ;
#27695=ORIENTED_EDGE ( 'NONE', *, *, #24733, .T. ) ;
#27701=CYLINDRICAL_SURFACE ( 'NONE', #37754, 2.000000000000001776 ) ;
#27709=VECTOR ( 'NONE', #4336, 1000.000000000000000 ) ;
#27710=ORIENTED_EDGE ( 'NONE', *, *, #10135, .T. ) ;
#27712=CARTESIAN_POINT ( 'NONE',  ( 339.9999999999999432, -169.0000000000001137, -344.0000000000002842 ) ) ;
#27713=ORIENTED_EDGE ( 'NONE', *, *, #6379, .F. ) ;
#27717=EDGE_CURVE ( 'NONE', #27106, #5103, #30812, .T. ) ;
#27719=PLANE ( 'NONE',  #49291 ) ;
#27721=ORIENTED_EDGE ( 'NONE', *, *, #18115, .F. ) ;
#27729=ORIENTED_EDGE ( 'NONE', *, *, #12107, .F. ) ;
#27742=VERTEX_POINT ( 'NONE', #37760 ) ;
#27752=FACE_OUTER_BOUND ( 'NONE', #5990, .T. ) ;
#27754=EDGE_CURVE ( 'NONE', #4028, #17487, #2577, .T. ) ;
#27764=DIRECTION ( 'NONE',  ( 0.000000000000000000, 0.000000000000000000, -1.000000000000000000 ) ) ;
#27775=FACE_OUTER_BOUND ( 'NONE', #49450, .T. ) ;
#27777=ORIENTED_EDGE ( 'NONE', *, *, #14535, .F. ) ;
#27785=ORIENTED_EDGE ( 'NONE', *, *, #48139, .F. ) ;
#27789=ORIENTED_EDGE ( 'NONE', *, *, #14067, .F. ) ;
#27791=VECTOR ( 'NONE', #2027, 1000.000000000000000 ) ;
#27795=EDGE_LOOP ( 'NONE', ( #37408, #33898, #30368, #36828 ) ) ;
#27797=VERTEX_POINT ( 'NONE', #42837 ) ;
#27798=FACE_OUTER_BOUND ( 'NONE', #40436, .T. ) ;
#27801=EDGE_CURVE ( 'NONE', #35970, #4444, #2928, .T. ) ;
#27809=ORIENTED_EDGE ( 'NONE', *, *, #14067, .T. ) ;
#27811=DIRECTION ( 'NONE',  ( 1.860490536778032451E-50, 0.000000000000000000, -1.000000000000000000 ) ) ;
#27815=CARTESIAN_POINT ( 'NONE',  ( 358.0000000000000000, -169.0000000000001137, 344.0000000000000000 ) ) ;
#27816=CARTESIAN_POINT ( 'NONE',  ( 168.9999999999999716, 175.0000000000000284, -344.0000000000001137 ) ) ;
#27818=VERTEX_POINT ( 'NONE', #276 ) ;
#27822=AXIS2_PLACEMENT_3D ( 'NONE', #29389, #45008, #36621 ) ;
#27824=AXIS2_PLACEMENT_3D ( 'NONE', #5225, #20875, #29086 ) ;
#27826=EDGE_CURVE ( 'NONE', #15345, #3809, #39528, .T. ) ;
#27828=MECHANICAL_DESIGN_GEOMETRIC_PRESENTATION_REPRESENTATION('',(#14697),#48350);
#27834=ORIENTED_EDGE ( 'NONE', *, *, #12596, .F. ) ;
#27836=DIRECTION ( 'NONE',  ( 0.000000000000000000, 0.000000000000000000, -1.000000000000000000 ) ) ;
#27848=LINE ( 'NONE', #35824, #44968 ) ;
#27857=CARTESIAN_POINT ( 'NONE',  ( 344.0000000000000568, 183.0000000000000284, 349.9999999999998863 ) ) ;
#27861=ADVANCED_FACE ( 'NONE', ( #4622 ), #23355, .T. ) ;
#27863=ORIENTED_EDGE ( 'NONE', *, *, #24019, .T. ) ;
#27869=EDGE_CURVE ( 'NONE', #7708, #19185, #15408, .T. ) ;
#27871=ORIENTED_EDGE ( 'NONE', *, *, #943, .T. ) ;
#27888=CARTESIAN_POINT ( 'NONE',  ( 349.9999999999999432, -184.9999999999999716, 355.9999999999997726 ) ) ;
#27889=FACE_OUTER_BOUND ( 'NONE', #24789, .T. ) ;
#27893=ORIENTED_EDGE ( 'NONE', *, *, #30285, .F. ) ;
#27895=AXIS2_PLACEMENT_3D ( 'NONE', #8267, #7769, #8023 ) ;
#27896=CARTESIAN_POINT ( 'NONE',  ( 185.0000000000000000, -9.999999999999953815, -111.0000000000001563 ) ) ;
#27900=AXIS2_PLACEMENT_3D ( 'NONE', #7347, #23761, #15310 ) ;
#27902=AXIS2_PLACEMENT_3D ( 'NONE', #16127, #35395, #12268 ) ;
#27905=EDGE_LOOP ( 'NONE', ( #23123, #24016, #15549, #11201 ) ) ;
#27908=EDGE_CURVE ( 'NONE', #25084, #37811, #9497, .T. ) ;
#27910=ORIENTED_EDGE ( 'NONE', *, *, #33383, .F. ) ;
#27915=ORIENTED_EDGE ( 'NONE', *, *, #28018, .T. ) ;
#27916=CARTESIAN_POINT ( 'NONE',  ( 339.9999999999999432, 171.9999999999999432, -347.0000000000000568 ) ) ;
#27921=ORIENTED_EDGE ( 'NONE', *, *, #37480, .T. ) ;
#27923=ORIENTED_EDGE ( 'NONE', *, *, #23813, .F. ) ;
#27938=CIRCLE ( 'NONE', #35319, 2.000000000000001776 ) ;
#27941=CARTESIAN_POINT ( 'NONE',  ( 356.0000000000000000, 185.0000000000000284, -360.0000000000002274 ) ) ;
#27944=CARTESIAN_POINT ( 'NONE',  ( 356.0000000000000000, 165.0000000000001705, -340.0000000000002842 ) ) ;
#27961=DIRECTION ( 'NONE',  ( 1.000000000000000000, -4.758098676964956461E-16, -8.975803739141899931E-48 ) ) ;
#27971=VERTEX_POINT ( 'NONE', #28477 ) ;
#27973=CARTESIAN_POINT ( 'NONE',  ( 356.0000000000001137, 183.0000000000000284, 349.9999999999998295 ) ) ;
#27976=( BOUNDED_CURVE ( )  B_SPLINE_CURVE ( 3, ( #1688, #28623, #35852, #43513 ),
 .UNSPECIFIED., .F., .F. ) 
 B_SPLINE_CURVE_WITH_KNOTS ( ( 4, 4 ),
 ( 4.712388980384689674, 6.283185307179586232 ),
 .UNSPECIFIED. ) 
 CURVE ( )  GEOMETRIC_REPRESENTATION_ITEM ( )  RATIONAL_B_SPLINE_CURVE ( ( 1.000000000000000000, 0.8047378541243649375, 0.8047378541243649375, 1.000000000000000000 ) ) 
 REPRESENTATION_ITEM ( '' )  );
#27978=ORIENTED_EDGE ( 'NONE', *, *, #44046, .T. ) ;
#27980=CARTESIAN_POINT ( 'NONE',  ( 169.0000000000000000, -174.9999999999999716, -95.00000000000014211 ) ) ;
#27984=CARTESIAN_POINT ( 'NONE',  ( 358.0000000000000000, 175.0000000000000284, -106.0000000000001990 ) ) ;
#27988=ORIENTED_EDGE ( 'NONE', *, *, #30567, .F. ) ;
#27991=CARTESIAN_POINT ( 'NONE',  ( 355.9999999999999432, -174.9999999999999432, 355.9999999999998295 ) ) ;
#27995=ORIENTED_EDGE ( 'NONE', *, *, #29599, .F. ) ;
#27997=EDGE_CURVE ( 'NONE', #22310, #29971, #26923, .T. ) ;
#28012=EDGE_CURVE ( 'NONE', #49667, #39568, #18353, .T. ) ;
#28018=EDGE_CURVE ( 'NONE', #46031, #11650, #44098, .T. ) ;
#28024=CARTESIAN_POINT ( 'NONE',  ( 167.0000000000000284, 175.0000000000000284, 355.9999999999998863 ) ) ;
#28028=ORIENTED_EDGE ( 'NONE', *, *, #48983, .F. ) ;
#28031=VERTEX_POINT ( 'NONE', #16933 ) ;
#28033=CARTESIAN_POINT ( 'NONE',  ( 181.0000000000000568, -164.9999999999999432, 357.9999999999998863 ) ) ;
#28034=CARTESIAN_POINT ( 'NONE',  ( 183.0000000000000284, -174.9999999999999716, -99.00000000000014211 ) ) ;
#28043=EDGE_CURVE ( 'NONE', #9239, #19835, #25076, .T. ) ;
#28051=EDGE_LOOP ( 'NONE', ( #46594, #28926, #40042, #5340 ) ) ;
#28052=CARTESIAN_POINT ( 'NONE',  ( 358.0000000000000000, 169.0000000000001705, -344.0000000000002842 ) ) ;
#28056=ORIENTED_EDGE ( 'NONE', *, *, #34538, .T. ) ;
#28059=LINE ( 'NONE', #4457, #14655 ) ;
#28065=FACE_OUTER_BOUND ( 'NONE', #41069, .T. ) ;
#28067=CARTESIAN_POINT ( 'NONE',  ( 339.9999999999998863, -168.9999999999999432, 355.9999999999997726 ) ) ;
#28071=VECTOR ( 'NONE', #5245, 1000.000000000000000 ) ;
#28075=CYLINDRICAL_SURFACE ( 'NONE', #35230, 4.000000000000003553 ) ;
#28079=ORIENTED_EDGE ( 'NONE', *, *, #4243, .T. ) ;
#28082=DIRECTION ( 'NONE',  ( 0.000000000000000000, 0.000000000000000000, -1.000000000000000000 ) ) ;
#28094=ORIENTED_EDGE ( 'NONE', *, *, #11496, .F. ) ;
#28095=LINE ( 'NONE', #4489, #32142 ) ;
#28099=AXIS2_PLACEMENT_3D ( 'NONE', #3892, #4154, #4663 ) ;
#28102=CIRCLE ( 'NONE', #9271, 4.000000000000003553 ) ;
#28104=VECTOR ( 'NONE', #4029, 1000.000000000000000 ) ;
#28108=AXIS2_PLACEMENT_3D ( 'NONE', #49181, #18423, #37698 ) ;
#28115=EDGE_LOOP ( 'NONE', ( #44609, #43207, #27710, #40792 ) ) ;
#28123=CARTESIAN_POINT ( 'NONE',  ( 168.9999999999999716, -272.4999999999999432, -341.9999999999999432 ) ) ;
#28125=ORIENTED_EDGE ( 'NONE', *, *, #36709, .T. ) ;
#28126=EDGE_CURVE ( 'NONE', #1207, #18285, #11189, .T. ) ;
#28133=EDGE_CURVE ( 'NONE', #32484, #6330, #19631, .T. ) ;
#28140=PLANE ( 'NONE',  #47724 ) ;
#28143=AXIS2_PLACEMENT_3D ( 'NONE', #28259, #12103, #8008 ) ;
#28150=ORIENTED_EDGE ( 'NONE', *, *, #29289, .T. ) ;
#28158=EDGE_CURVE ( 'NONE', #3658, #16118, #31715, .T. ) ;
#28168=DIRECTION ( 'NONE',  ( 0.000000000000000000, -1.000000000000000000, 0.000000000000000000 ) ) ;
#28172=DIRECTION ( 'NONE',  ( 0.000000000000000000, 1.000000000000000000, 3.186989995019654210E-49 ) ) ;
#28174=AXIS2_PLACEMENT_3D ( 'NONE', #41837, #22588, #34166 ) ;
#28175=VERTEX_POINT ( 'NONE', #8098 ) ;
#28178=DIRECTION ( 'NONE',  ( 0.000000000000000000, 0.000000000000000000, -1.000000000000000000 ) ) ;
#28180=CARTESIAN_POINT ( 'NONE',  ( -5.000000000000000000, -175.0000000000000284, -350.0000000000002274 ) ) ;
#28187=CARTESIAN_POINT ( 'NONE',  ( 357.9999999999998863, -182.1715728752538155, 357.1715728752536734 ) ) ;
#28191=CARTESIAN_POINT ( 'NONE',  ( 169.0000000000000000, -174.9999999999999716, -99.00000000000014211 ) ) ;
#28200=DIRECTION ( 'NONE',  ( -2.958228394578793832E-31, 0.000000000000000000, -1.000000000000000000 ) ) ;
#28207=CYLINDRICAL_SURFACE ( 'NONE', #41754, 2.000000000000001776 ) ;
#28208=VECTOR ( 'NONE', #37394, 1000.000000000000000 ) ;
#28212=DIRECTION ( 'NONE',  ( 0.000000000000000000, 0.000000000000000000, 1.000000000000000000 ) ) ;
#28219=ADVANCED_FACE ( 'NONE', ( #32706 ), #401, .T. ) ;
#28220=EDGE_CURVE ( 'NONE', #45172, #22827, #16802, .T. ) ;
#28232=ORIENTED_EDGE ( 'NONE', *, *, #42774, .T. ) ;
#28235=VECTOR ( 'NONE', #18698, 1000.000000000000000 ) ;
#28245=ORIENTED_EDGE ( 'NONE', *, *, #44390, .F. ) ;
#28248=DIRECTION ( 'NONE',  ( -1.000000000000000000, 1.586032892321652236E-16, 1.586032892321651989E-16 ) ) ;
#28252=EDGE_CURVE ( 'NONE', #15011, #34763, #12935, .T. ) ;
#28256=CARTESIAN_POINT ( 'NONE',  ( -5.000000000000000000, -175.0000000000000284, 350.0000000000002274 ) ) ;
#28258=DIRECTION ( 'NONE',  ( 0.000000000000000000, 0.000000000000000000, -1.000000000000000000 ) ) ;
#28259=CARTESIAN_POINT ( 'NONE',  ( 181.0000000000000000, -268.5000000000000000, -114.9999999999999147 ) ) ;
#28263=DIRECTION ( 'NONE',  ( -0.000000000000000000, -1.000000000000000000, 2.537652627714643577E-15 ) ) ;
#28268=DIRECTION ( 'NONE',  ( 1.000000000000000000, 0.000000000000000000, 0.000000000000000000 ) ) ;
#28270=ORIENTED_EDGE ( 'NONE', *, *, #27801, .F. ) ;
#28278=VECTOR ( 'NONE', #28833, 1000.000000000000000 ) ;
#28284=ORIENTED_EDGE ( 'NONE', *, *, #46065, .T. ) ;
#28285=ORIENTED_EDGE ( 'NONE', *, *, #34749, .F. ) ;
#28286=CARTESIAN_POINT ( 'NONE',  ( -5.000000000000000000, 184.8000000000000114, 359.7999999999997840 ) ) ;
#28289=CARTESIAN_POINT ( 'NONE',  ( 168.9999999999999716, -168.9999999999999432, -350.0000000000001705 ) ) ;
#28291=LINE ( 'NONE', #20334, #39565 ) ;
#28293=DIRECTION ( 'NONE',  ( 1.000000000000000000, 0.000000000000000000, 0.000000000000000000 ) ) ;
#28295=LINE ( 'NONE', #4442, #16533 ) ;
#28312=FACE_BOUND ( 'NONE', #11506, .T. ) ;
#28313=PLANE ( 'NONE',  #42251 ) ;
#28316=VECTOR ( 'NONE', #4323, 1000.000000000000000 ) ;
#28320=EDGE_CURVE ( 'NONE', #30554, #13154, #34764, .T. ) ;
#28336=CARTESIAN_POINT ( 'NONE',  ( 164.9999999999999716, -268.5000000000002842, -114.9999999999999147 ) ) ;
#28341=ORIENTED_EDGE ( 'NONE', *, *, #15123, .F. ) ;
#28342=FACE_OUTER_BOUND ( 'NONE', #36074, .T. ) ;
#28347=ORIENTED_EDGE ( 'NONE', *, *, #41707, .F. ) ;
#28353=CARTESIAN_POINT ( 'NONE',  ( 166.9999999999999716, -184.9999999999999716, -344.0000000000001137 ) ) ;
#28360=DIRECTION ( 'NONE',  ( -1.586032880504786307E-16, 1.654361225106055350E-24, -1.000000000000000000 ) ) ;
#28372=CARTESIAN_POINT ( 'NONE',  ( 167.0000000000000000, 2.775557561562891351E-14, -99.00000000000014211 ) ) ;
#28373=VERTEX_POINT ( 'NONE', #33228 ) ;
#28378=LINE ( 'NONE', #17072, #28579 ) ;
#28383=EDGE_CURVE ( 'NONE', #8172, #36234, #34137, .T. ) ;
#28385=EDGE_CURVE ( 'NONE', #28730, #40964, #13697, .T. ) ;
#28401=ORIENTED_EDGE ( 'NONE', *, *, #23346, .T. ) ;
#28403=CARTESIAN_POINT ( 'NONE',  ( 359.9999999999999432, -174.9999999999999432, 355.9999999999998295 ) ) ;
#28404=LINE ( 'NONE', #39957, #37335 ) ;
#28405=VERTEX_POINT ( 'NONE', #46474 ) ;
#28407=VERTEX_POINT ( 'NONE', #11366 ) ;
#28410=CIRCLE ( 'NONE', #24318, 2.000000000000001776 ) ;
#28416=ORIENTED_EDGE ( 'NONE', *, *, #29778, .F. ) ;
#28418=CARTESIAN_POINT ( 'NONE',  ( 181.0000000000000853, -164.9999999999999432, -115.0000000000001990 ) ) ;
#28419=VERTEX_POINT ( 'NONE', #11630 ) ;
#28421=LINE ( 'NONE', #35632, #20123 ) ;
#28425=CARTESIAN_POINT ( 'NONE',  ( 164.9999999999999716, -256.4999999999999432, -349.9999999999999432 ) ) ;
#28435=VECTOR ( 'NONE', #23554, 1000.000000000000000 ) ;
#28447=CARTESIAN_POINT ( 'NONE',  ( 164.9999999999999716, -81.49999999999997158, -350.0000000000001705 ) ) ;
#28449=EDGE_CURVE ( 'NONE', #17284, #9063, #36605, .T. ) ;
#28452=VECTOR ( 'NONE', #14023, 1000.000000000000000 ) ;
#28456=EDGE_CURVE ( 'NONE', #44740, #45613, #7266, .T. ) ;
#28464=ORIENTED_EDGE ( 'NONE', *, *, #27122, .F. ) ;
#28466=CARTESIAN_POINT ( 'NONE',  ( 181.0000000000000000, 6.000000000000060396, -350.0000000000001705 ) ) ;
#28468=DIRECTION ( 'NONE',  ( -1.000000000000000000, 3.172065784643302499E-16, 1.942330104924128867E-32 ) ) ;
#28471=VERTEX_POINT ( 'NONE', #38842 ) ;
#28477=CARTESIAN_POINT ( 'NONE',  ( 5.551115123125782702E-14, -180.9999999999999716, 357.9999999999997726 ) ) ;
#28479=DIRECTION ( 'NONE',  ( 0.000000000000000000, 2.537652627714642000E-15, 1.000000000000000000 ) ) ;
#28491=PLANE ( 'NONE',  #3622 ) ;
#28493=DIRECTION ( 'NONE',  ( 0.000000000000000000, 0.000000000000000000, 1.000000000000000000 ) ) ;
#28497=CARTESIAN_POINT ( 'NONE',  ( 166.9999999999999716, -268.5000000000000000, -114.9999999999999289 ) ) ;
#28499=EDGE_CURVE ( 'NONE', #26133, #12204, #49629, .T. ) ;
#28501=ORIENTED_EDGE ( 'NONE', *, *, #43669, .F. ) ;
#28513=EDGE_CURVE ( 'NONE', #25177, #45390, #42657, .T. ) ;
#28514=CARTESIAN_POINT ( 'NONE',  ( 356.0000000000000000, -165.0000000000001137, -340.0000000000002842 ) ) ;
#28517=ORIENTED_EDGE ( 'NONE', *, *, #31296, .F. ) ;
#28521=CARTESIAN_POINT ( 'NONE',  ( 356.0000000000001137, 181.0000000000000284, 349.9999999999998863 ) ) ;
#28525=CYLINDRICAL_SURFACE ( 'NONE', #18297, 4.000000000000003553 ) ;
#28527=ORIENTED_EDGE ( 'NONE', *, *, #13, .T. ) ;
#28532=DIRECTION ( 'NONE',  ( -1.586032892321652236E-16, -1.000000000000000000, -6.853681917100419162E-49 ) ) ;
#28533=CARTESIAN_POINT ( 'NONE',  ( 339.9999999999998863, -185.0000000000001421, -349.9999999999998863 ) ) ;
#28535=VERTEX_POINT ( 'NONE', #9046 ) ;
#28539=CARTESIAN_POINT ( 'NONE',  ( 185.0000000000000000, 165.0000000000000000, -344.0000000000001137 ) ) ;
#28544=DIRECTION ( 'NONE',  ( -1.000000000000000000, 0.000000000000000000, 0.000000000000000000 ) ) ;
#28545=DIRECTION ( 'NONE',  ( 1.000000000000000000, -3.172065745548403743E-16, 1.587271980518778491E-16 ) ) ;
#28557=ORIENTED_EDGE ( 'NONE', *, *, #19975, .F. ) ;
#28562=CARTESIAN_POINT ( 'NONE',  ( 0.000000000000000000, -182.9999999999999716, -344.0000000000001705 ) ) ;
#28568=CARTESIAN_POINT ( 'NONE',  ( 356.0000000000000000, 165.0000000000000000, -340.0000000000001137 ) ) ;
#28573=PLANE ( 'NONE',  #6488 ) ;
#28574=ORIENTED_EDGE ( 'NONE', *, *, #39520, .F. ) ;
#28575=CARTESIAN_POINT ( 'NONE',  ( 350.0000000000000000, -180.9999999999999716, -340.0000000000001705 ) ) ;
#28579=VECTOR ( 'NONE', #8867, 1000.000000000000000 ) ;
#28582=LINE ( 'NONE', #8587, #44235 ) ;
#28584=CARTESIAN_POINT ( 'NONE',  ( 181.0000000000000000, -272.4999999999999432, -349.9999999999999432 ) ) ;
#28586=VERTEX_POINT ( 'NONE', #28034 ) ;
#28589=ADVANCED_FACE ( 'NONE', ( #12377 ), #43178, .T. ) ;
#28590=VECTOR ( 'NONE', #22200, 1000.000000000000000 ) ;
#28595=CARTESIAN_POINT ( 'NONE',  ( 350.0000000000000000, 169.0000000000000000, -358.0000000000002274 ) ) ;
#28601=PLANE ( 'NONE',  #27085 ) ;
#28603=ORIENTED_EDGE ( 'NONE', *, *, #23969, .F. ) ;
#28609=DIRECTION ( 'NONE',  ( 6.203854594147707562E-25, -2.067951531382569187E-25, 1.000000000000000000 ) ) ;
#28610=AXIS2_PLACEMENT_3D ( 'NONE', #24427, #36486, #32626 ) ;
#28611=ORIENTED_EDGE ( 'NONE', *, *, #48191, .T. ) ;
#28616=DIRECTION ( 'NONE',  ( -2.874857526315639190E-31, 1.000000000000000000, -2.537652627714642000E-15 ) ) ;
#28618=AXIS2_PLACEMENT_3D ( 'NONE', #42037, #46367, #26135 ) ;
#28619=EDGE_CURVE ( 'NONE', #39109, #5029, #36007, .T. ) ;
#28621=VECTOR ( 'NONE', #48897, 1000.000000000000000 ) ;
#28623=CARTESIAN_POINT ( 'NONE',  ( 342.0000000000000000, -167.8284271247462414, -342.8284271247464972 ) ) ;
#28627=LINE ( 'NONE', #31489, #16347 ) ;
#28640=CARTESIAN_POINT ( 'NONE',  ( 164.9999999999999716, -272.4999999999999432, -344.0000000000001137 ) ) ;
#28644=ADVANCED_FACE ( 'NONE', ( #46983, #19820 ), #39346, .T. ) ;
#28671=ORIENTED_EDGE ( 'NONE', *, *, #32837, .T. ) ;
#28677=PLANE ( 'NONE',  #19851 ) ;
#28679=DIRECTION ( 'NONE',  ( 0.000000000000000000, 1.000000000000000000, 0.000000000000000000 ) ) ;
#28680=DIRECTION ( 'NONE',  ( -0.000000000000000000, 1.000000000000000000, 0.000000000000000000 ) ) ;
#28683=DIRECTION ( 'NONE',  ( 0.000000000000000000, 0.000000000000000000, -1.000000000000000000 ) ) ;
#28687=CARTESIAN_POINT ( 'NONE',  ( 169.0000000000000284, 165.0000000000000000, 343.9999999999998863 ) ) ;
#28688=EDGE_CURVE ( 'NONE', #48047, #35576, #17981, .T. ) ;
#28691=UNCERTAINTY_MEASURE_WITH_UNIT (LENGTH_MEASURE( 1.000000000000000082E-05 ), #22748, 'distance_accuracy_value', 'NONE');
#28696=CIRCLE ( 'NONE', #32007, 4.000000000000003553 ) ;
#28698=( GEOMETRIC_REPRESENTATION_CONTEXT ( 3 ) GLOBAL_UNCERTAINTY_ASSIGNED_CONTEXT ( ( #42772 ) ) GLOBAL_UNIT_ASSIGNED_CONTEXT ( ( #21041, #22296, #46109 ) ) REPRESENTATION_CONTEXT ( 'NONE', 'WORKASPACE' ) );
#28700=CARTESIAN_POINT ( 'NONE',  ( 166.9999999999999716, -180.9999999999999716, -350.0000000000001705 ) ) ;
#28704=ORIENTED_EDGE ( 'NONE', *, *, #18249, .F. ) ;
#28712=VERTEX_POINT ( 'NONE', #25701 ) ;
#28720=DIRECTION ( 'NONE',  ( -1.000000000000000000, 0.000000000000000000, -2.958228394578794270E-31 ) ) ;
#28724=CARTESIAN_POINT ( 'NONE',  ( 168.9999999999999716, -270.4999999999999432, -349.9999999999999432 ) ) ;
#28726=FACE_OUTER_BOUND ( 'NONE', #5921, .T. ) ;
#28730=VERTEX_POINT ( 'NONE', #32909 ) ;
#28735=LINE ( 'NONE', #33597, #584 ) ;
#28736=DIRECTION ( 'NONE',  ( -3.172065784643302499E-16, -1.000000000000000000, 2.537652627714642000E-15 ) ) ;
#28737=VERTEX_POINT ( 'NONE', #40835 ) ;
#28738=ORIENTED_EDGE ( 'NONE', *, *, #41507, .T. ) ;
#28741=VECTOR ( 'NONE', #26722, 1000.000000000000000 ) ;
#28745=FACE_OUTER_BOUND ( 'NONE', #3187, .T. ) ;
#28746=CARTESIAN_POINT ( 'NONE',  ( 0.000000000000000000, 167.0000000000000000, -344.0000000000001705 ) ) ;
#28749=ORIENTED_EDGE ( 'NONE', *, *, #23703, .F. ) ;
#28753=ORIENTED_EDGE ( 'NONE', *, *, #26501, .T. ) ;
#28768=ORIENTED_EDGE ( 'NONE', *, *, #14278, .T. ) ;
#28771=CARTESIAN_POINT ( 'NONE',  ( 168.9999999999999716, -256.5000000000000000, -114.9999999999999574 ) ) ;
#28779=ORIENTED_EDGE ( 'NONE', *, *, #8948, .T. ) ;
#28783=CARTESIAN_POINT ( 'NONE',  ( 166.9999999999999716, -164.9999999999999432, -344.0000000000001137 ) ) ;
#28793=CARTESIAN_POINT ( 'NONE',  ( 168.9999999999999716, -184.9999999999999716, -356.0000000000001705 ) ) ;
#28800=DIRECTION ( 'NONE',  ( -0.000000000000000000, -1.000000000000000000, 2.537652627714643577E-15 ) ) ;
#28801=PLANE ( 'NONE',  #14510 ) ;
#28804=FACE_BOUND ( 'NONE', #25060, .T. ) ;
#28811=LINE ( 'NONE', #43941, #35571 ) ;
#28826=EDGE_CURVE ( 'NONE', #14950, #41788, #26205, .T. ) ;
#28827=DIRECTION ( 'NONE',  ( 0.000000000000000000, -1.000000000000000000, 0.000000000000000000 ) ) ;
#28829=CYLINDRICAL_SURFACE ( 'NONE', #14691, 2.000000000000001776 ) ;
#28830=ORIENTED_EDGE ( 'NONE', *, *, #2693, .F. ) ;
#28832=VECTOR ( 'NONE', #36204, 1000.000000000000000 ) ;
#28833=DIRECTION ( 'NONE',  ( -0.000000000000000000, -1.000000000000000000, -0.000000000000000000 ) ) ;
#28836=EDGE_CURVE ( 'NONE', #5029, #43960, #17708, .T. ) ;
#28840=FACE_OUTER_BOUND ( 'NONE', #34958, .T. ) ;
#28844=LINE ( 'NONE', #13443, #24266 ) ;
#28851=CARTESIAN_POINT ( 'NONE',  ( 181.0000000000000284, -174.9999999999999716, -115.0000000000001563 ) ) ;
#28853=DIRECTION ( 'NONE',  ( 0.000000000000000000, 0.000000000000000000, -1.000000000000000000 ) ) ;
#28857=ORIENTED_EDGE ( 'NONE', *, *, #46352, .T. ) ;
#28863=VECTOR ( 'NONE', #18875, 1000.000000000000000 ) ;
#28871=VECTOR ( 'NONE', #30402, 1000.000000000000000 ) ;
#28874=ORIENTED_EDGE ( 'NONE', *, *, #8016, .T. ) ;
#28876=CARTESIAN_POINT ( 'NONE',  ( 183.0000000000000284, -174.9999999999999716, -99.00000000000014211 ) ) ;
#28878=VECTOR ( 'NONE', #42346, 1000.000000000000000 ) ;
#28887=EDGE_CURVE ( 'NONE', #41339, #38600, #18232, .T. ) ;
#28889=CARTESIAN_POINT ( 'NONE',  ( 168.9999999999999716, 6.000000000000060396, -350.0000000000001705 ) ) ;
#28890=DIRECTION ( 'NONE',  ( -1.000000000000000000, 0.000000000000000000, 0.000000000000000000 ) ) ;
#28891=AXIS2_PLACEMENT_3D ( 'NONE', #35561, #402, #16049 ) ;
#28895=CARTESIAN_POINT ( 'NONE',  ( 343.9999999999999432, -183.0000000000002558, -358.0000000000003411 ) ) ;
#28901=ORIENTED_EDGE ( 'NONE', *, *, #723, .T. ) ;
#28905=VECTOR ( 'NONE', #8455, 1000.000000000000000 ) ;
#28912=ORIENTED_EDGE ( 'NONE', *, *, #46065, .F. ) ;
#28920=PLANE ( 'NONE',  #40933 ) ;
#28925=CARTESIAN_POINT ( 'NONE',  ( 341.9999999999999432, -182.1715728752539860, -357.1715728752541281 ) ) ;
#28926=ORIENTED_EDGE ( 'NONE', *, *, #33383, .T. ) ;
#28931=FACE_BOUND ( 'NONE', #359, .T. ) ;
#28933=LINE ( 'NONE', #13526, #18347 ) ;
#28936=DIRECTION ( 'NONE',  ( 0.000000000000000000, -1.000000000000000000, 2.969158215481698263E-48 ) ) ;
#28938=EDGE_CURVE ( 'NONE', #13304, #11040, #11053, .T. ) ;
#28943=AXIS2_PLACEMENT_3D ( 'NONE', #39819, #12588, #7750 ) ;
#28947=CARTESIAN_POINT ( 'NONE',  ( 358.0000000000000000, 169.0000000000001705, -344.0000000000002842 ) ) ;
#28950=FACE_OUTER_BOUND ( 'NONE', #35418, .T. ) ;
#28951=LINE ( 'NONE', #13041, #22092 ) ;
#28956=DIRECTION ( 'NONE',  ( 1.132880637372608740E-16, 4.718402560806925739E-50, 1.000000000000000000 ) ) ;
#28966=CIRCLE ( 'NONE', #2733, 4.000000000000003553 ) ;
#28967=ORIENTED_EDGE ( 'NONE', *, *, #14993, .T. ) ;
#28973=ORIENTED_EDGE ( 'NONE', *, *, #41692, .F. ) ;
#28976=DIRECTION ( 'NONE',  ( 0.000000000000000000, 1.000000000000000000, 0.000000000000000000 ) ) ;
#28982=ORIENTED_EDGE ( 'NONE', *, *, #33432, .T. ) ;
#28989=FACE_OUTER_BOUND ( 'NONE', #40465, .T. ) ;
#28991=VERTEX_POINT ( 'NONE', #39032 ) ;
#28997=ADVANCED_FACE ( 'NONE', ( #31591 ), #35700, .T. ) ;
#28998=ORIENTED_EDGE ( 'NONE', *, *, #17772, .F. ) ;
#29008=ORIENTED_EDGE ( 'NONE', *, *, #31226, .F. ) ;
#29014=AXIS2_PLACEMENT_3D ( 'NONE', #29718, #13051, #33081 ) ;
#29017=VERTEX_POINT ( 'NONE', #8228 ) ;
#29023=CARTESIAN_POINT ( 'NONE',  ( 339.9999999999999432, -168.9999999999999432, 343.9999999999998295 ) ) ;
#29026=ORIENTED_EDGE ( 'NONE', *, *, #13651, .F. ) ;
#29028=EDGE_CURVE ( 'NONE', #5747, #48314, #20276, .T. ) ;
#29039=DIRECTION ( 'NONE',  ( 0.000000000000000000, 0.000000000000000000, 1.000000000000000000 ) ) ;
#29042=VECTOR ( 'NONE', #10102, 1000.000000000000000 ) ;
#29043=CARTESIAN_POINT ( 'NONE',  ( 356.0000000000000568, -185.0000000000001421, 360.0000000000000000 ) ) ;
#29046=VECTOR ( 'NONE', #38059, 1000.000000000000000 ) ;
#29048=DIRECTION ( 'NONE',  ( 1.000000000000000000, 0.000000000000000000, 7.793956916774525800E-48 ) ) ;
#29050=AXIS2_PLACEMENT_3D ( 'NONE', #5693, #17253, #36520 ) ;
#29063=ORIENTED_EDGE ( 'NONE', *, *, #27717, .F. ) ;
#29064=CARTESIAN_POINT ( 'NONE',  ( 343.9999999999999432, -165.0000000000001137, -340.0000000000002842 ) ) ;
#29068=DIRECTION ( 'NONE',  ( 4.758098676964956461E-16, 1.000000000000000000, 0.000000000000000000 ) ) ;
#29069=EDGE_CURVE ( 'NONE', #38138, #43962, #44850, .T. ) ;
#29070=VECTOR ( 'NONE', #28616, 1000.000000000000000 ) ;
#29080=DIRECTION ( 'NONE',  ( 1.333906992743555050E-23, -1.000000000000000000, 0.000000000000000000 ) ) ;
#29083=FACE_OUTER_BOUND ( 'NONE', #48117, .T. ) ;
#29086=DIRECTION ( 'NONE',  ( 0.000000000000000000, 0.000000000000000000, 1.000000000000000000 ) ) ;
#29090=EDGE_CURVE ( 'NONE', #2228, #46883, #25962, .T. ) ;
#29093=ORIENTED_EDGE ( 'NONE', *, *, #48983, .T. ) ;
#29100=VERTEX_POINT ( 'NONE', #21787 ) ;
#29103=VECTOR ( 'NONE', #47344, 1000.000000000000000 ) ;
#29109=DIRECTION ( 'NONE',  ( -1.000000000000000000, 0.000000000000000000, 0.000000000000000000 ) ) ;
#29111=VECTOR ( 'NONE', #47335, 1000.000000000000000 ) ;
#29112=EDGE_LOOP ( 'NONE', ( #27834, #7847, #12316, #33522 ) ) ;
#29118=ORIENTED_EDGE ( 'NONE', *, *, #47497, .T. ) ;
#29131=DIRECTION ( 'NONE',  ( 1.132880637372608740E-16, 4.718402560806925739E-50, 1.000000000000000000 ) ) ;
#29133=EDGE_CURVE ( 'NONE', #46025, #16830, #28735, .T. ) ;
#29134=ADVANCED_FACE ( 'NONE', ( #41036 ), #37217, .F. ) ;
#29148=CARTESIAN_POINT ( 'NONE',  ( 339.9999999999999432, 181.0000000000000568, -356.0000000000002274 ) ) ;
#29156=MECHANICAL_DESIGN_GEOMETRIC_PRESENTATION_REPRESENTATION('',(#2942),#43103);
#29159=FACE_OUTER_BOUND ( 'NONE', #44147, .T. ) ;
#29161=DIRECTION ( 'NONE',  ( 1.000000000000000000, 0.000000000000000000, -1.860490536778032451E-50 ) ) ;
#29173=ADVANCED_FACE ( 'NONE', ( #37962 ), #11256, .T. ) ;
#29179=AXIS2_PLACEMENT_3D ( 'NONE', #31449, #47043, #46538 ) ;
#29180=ORIENTED_EDGE ( 'NONE', *, *, #2655, .F. ) ;
#29183=DIRECTION ( 'NONE',  ( -1.612977847700450206E-50, 0.000000000000000000, 1.000000000000000000 ) ) ;
#29186=EDGE_LOOP ( 'NONE', ( #28150, #43250, #49821, #20097 ) ) ;
#29187=ORIENTED_EDGE ( 'NONE', *, *, #7173, .T. ) ;
#29189=DIRECTION ( 'NONE',  ( -1.000000000000000000, 0.000000000000000000, -2.958228394578794270E-31 ) ) ;
#29190=ORIENTED_EDGE ( 'NONE', *, *, #34597, .T. ) ;
#29193=AXIS2_PLACEMENT_3D ( 'NONE', #24705, #29048, #9294 ) ;
#29197=DIRECTION ( 'NONE',  ( 0.000000000000000000, 0.000000000000000000, -1.000000000000000000 ) ) ;
#29202=VECTOR ( 'NONE', #31327, 1000.000000000000000 ) ;
#29210=ORIENTED_EDGE ( 'NONE', *, *, #2638, .F. ) ;
#29212=VECTOR ( 'NONE', #32646, 1000.000000000000000 ) ;
#29216=DIRECTION ( 'NONE',  ( 0.000000000000000000, 1.000000000000000000, 6.123233995736766036E-17 ) ) ;
#29219=DIRECTION ( 'NONE',  ( -3.172065784643302499E-16, -1.000000000000000000, 2.537652627714642000E-15 ) ) ;
#29225=CARTESIAN_POINT ( 'NONE',  ( 181.0000000000000000, -5.999999999999950262, -350.0000000000001705 ) ) ;
#29228=LINE ( 'NONE', #37694, #39387 ) ;
#29233=VECTOR ( 'NONE', #12992, 1000.000000000000000 ) ;
#29236=CARTESIAN_POINT ( 'NONE',  ( 0.000000000000000000, 181.0000000000000284, 355.9999999999997726 ) ) ;
#29237=CARTESIAN_POINT ( 'NONE',  ( 181.0000000000000284, -174.9999999999999716, -111.0000000000001563 ) ) ;
#29242=DIRECTION ( 'NONE',  ( 0.000000000000000000, -1.000000000000000000, 0.000000000000000000 ) ) ;
#29255=LINE ( 'NONE', #21811, #28235 ) ;
#29259=VERTEX_POINT ( 'NONE', #42036 ) ;
#29264=DIRECTION ( 'NONE',  ( 0.000000000000000000, -1.000000000000000000, 0.000000000000000000 ) ) ;
#29266=CYLINDRICAL_SURFACE ( 'NONE', #4963, 4.000000000000003553 ) ;
#29284=CARTESIAN_POINT ( 'NONE',  ( 340.0000000000000000, 169.0000000000000284, 359.9999999999998295 ) ) ;
#29287=DIRECTION ( 'NONE',  ( 0.000000000000000000, 1.000000000000000000, 0.000000000000000000 ) ) ;
#29289=EDGE_CURVE ( 'NONE', #32679, #21399, #14330, .T. ) ;
#29290=EDGE_LOOP ( 'NONE', ( #28603, #3192, #18912, #31047, #417, #31, #6970, #14752 ) ) ;
#29294=EDGE_CURVE ( 'NONE', #14457, #43944, #45019, .T. ) ;
#29299=CARTESIAN_POINT ( 'NONE',  ( 340.0000000000000568, 169.0000000000000000, 343.9999999999997726 ) ) ;
#29300=EDGE_CURVE ( 'NONE', #49733, #17553, #9580, .T. ) ;
#29305=CYLINDRICAL_SURFACE ( 'NONE', #31754, 4.000000000000003553 ) ;
#29308=ORIENTED_EDGE ( 'NONE', *, *, #15222, .F. ) ;
#29309=ORIENTED_EDGE ( 'NONE', *, *, #49394, .T. ) ;
#29319=( BOUNDED_CURVE ( )  B_SPLINE_CURVE ( 3, ( #36451, #1290, #40286, #13069 ),
 .UNSPECIFIED., .F., .F. ) 
 B_SPLINE_CURVE_WITH_KNOTS ( ( 4, 4 ),
 ( 1.570796326794896780, 3.141592653589793116 ),
 .UNSPECIFIED. ) 
 CURVE ( )  GEOMETRIC_REPRESENTATION_ITEM ( )  RATIONAL_B_SPLINE_CURVE ( ( 1.000000000000000000, 0.8047378541243650485, 0.8047378541243650485, 1.000000000000000000 ) ) 
 REPRESENTATION_ITEM ( '' )  );
#29322=EDGE_CURVE ( 'NONE', #36125, #46025, #28410, .T. ) ;
#29323=CIRCLE ( 'NONE', #24390, 2.000000000000001776 ) ;
#29325=CARTESIAN_POINT ( 'NONE',  ( 350.0000000000000000, 185.0000000000000284, -356.0000000000002274 ) ) ;
#29327=DIRECTION ( 'NONE',  ( 1.000000000000000000, 0.000000000000000000, 0.000000000000000000 ) ) ;
#29329=CARTESIAN_POINT ( 'NONE',  ( 0.000000000000000000, 169.0000000000000000, -356.0000000000002274 ) ) ;
#29332=CARTESIAN_POINT ( 'NONE',  ( 181.0000000000000000, 175.0000000000000284, -356.0000000000001705 ) ) ;
#29335=ORIENTED_EDGE ( 'NONE', *, *, #16177, .T. ) ;
#29339=CARTESIAN_POINT ( 'NONE',  ( 181.0000000000000000, -7.999999999999952038, -340.0000000000001137 ) ) ;
#29347=CARTESIAN_POINT ( 'NONE',  ( 166.9999999999999716, 175.0000000000000284, -344.0000000000001137 ) ) ;
#29362=VERTEX_POINT ( 'NONE', #15857 ) ;
#29373=LINE ( 'NONE', #44000, #20689 ) ;
#29374=EDGE_LOOP ( 'NONE', ( #12539, #20053, #22057, #37358 ) ) ;
#29378=DIRECTION ( 'NONE',  ( 0.000000000000000000, -3.186989995019654210E-49, -1.000000000000000000 ) ) ;
#29383=DIRECTION ( 'NONE',  ( 0.000000000000000000, -1.000000000000000000, 0.000000000000000000 ) ) ;
#29385=DIRECTION ( 'NONE',  ( 1.132880637372608740E-16, 4.718402560806925739E-50, 1.000000000000000000 ) ) ;
#29386=VECTOR ( 'NONE', #43263, 1000.000000000000000 ) ;
#29387=PLANE ( 'NONE',  #19854 ) ;
#29388=CARTESIAN_POINT ( 'NONE',  ( 181.0000000000000000, -9.999999999999953815, 339.9999999999998295 ) ) ;
#29389=CARTESIAN_POINT ( 'NONE',  ( -5.000000000000000000, 165.2000000000000171, 340.1999999999997044 ) ) ;
#29397=CARTESIAN_POINT ( 'NONE',  ( 181.0000000000000000, -5.999999999999950262, -340.0000000000001137 ) ) ;
#29400=FACE_OUTER_BOUND ( 'NONE', #7624, .T. ) ;
#29403=CARTESIAN_POINT ( 'NONE',  ( 164.9999999999999716, 175.0000000000000284, -356.0000000000001705 ) ) ;
#29405=EDGE_CURVE ( 'NONE', #23455, #48356, #44049, .T. ) ;
#29411=ORIENTED_EDGE ( 'NONE', *, *, #14993, .F. ) ;
#29418=DIRECTION ( 'NONE',  ( -2.874857526315640942E-31, 1.000000000000000000, -2.537652627714643577E-15 ) ) ;
#29428=AXIS2_PLACEMENT_3D ( 'NONE', #7726, #7211, #23366 ) ;
#29429=AXIS2_PLACEMENT_3D ( 'NONE', #41813, #45384, #34145 ) ;
#29430=ADVANCED_FACE ( 'NONE', ( #25575 ), #41216, .F. ) ;
#29433=VECTOR ( 'NONE', #19005, 1000.000000000000000 ) ;
#29439=FACE_OUTER_BOUND ( 'NONE', #38419, .T. ) ;
#29441=CARTESIAN_POINT ( 'NONE',  ( 181.0000000000000000, 8.000000000000062172, 339.9999999999998295 ) ) ;
#29442=LINE ( 'NONE', #17641, #42447 ) ;
#29449=VECTOR ( 'NONE', #38947, 1000.000000000000000 ) ;
#29451=EDGE_CURVE ( 'NONE', #12553, #27291, #20714, .T. ) ;
#29452=AXIS2_PLACEMENT_3D ( 'NONE', #43158, #40818, #40074 ) ;
#29456=CIRCLE ( 'NONE', #17153, 4.000000000000003553 ) ;
#29458=ORIENTED_EDGE ( 'NONE', *, *, #36855, .F. ) ;
#29461=DIRECTION ( 'NONE',  ( -0.000000000000000000, -0.000000000000000000, 1.000000000000000000 ) ) ;
#29463=DIRECTION ( 'NONE',  ( 0.000000000000000000, -1.000000000000000000, 0.000000000000000000 ) ) ;
#29467=VERTEX_POINT ( 'NONE', #5564 ) ;
#29469=CARTESIAN_POINT ( 'NONE',  ( 169.0000000000000284, 175.0000000000000284, 343.9999999999998863 ) ) ;
#29470=VECTOR ( 'NONE', #14177, 1000.000000000000000 ) ;
#29476=DIRECTION ( 'NONE',  ( 6.203854594147707562E-25, -2.067951531382569187E-25, 1.000000000000000000 ) ) ;
#29483=ORIENTED_EDGE ( 'NONE', *, *, #12669, .F. ) ;
#29487=ORIENTED_EDGE ( 'NONE', *, *, #26918, .F. ) ;
#29492=EDGE_LOOP ( 'NONE', ( #36083, #34477, #27777, #12672 ) ) ;
#29502=DIRECTION ( 'NONE',  ( 0.000000000000000000, -1.000000000000000000, 2.969158215481698263E-48 ) ) ;
#29503=VECTOR ( 'NONE', #48182, 1000.000000000000000 ) ;
#29506=VECTOR ( 'NONE', #79, 1000.000000000000000 ) ;
#29519=CARTESIAN_POINT ( 'NONE',  ( 358.0000000000001137, 182.1715728752538155, 357.1715728752536734 ) ) ;
#29521=CARTESIAN_POINT ( 'NONE',  ( 0.000000000000000000, 181.0000000000000284, -344.0000000000001705 ) ) ;
#29522=ORIENTED_EDGE ( 'NONE', *, *, #5845, .F. ) ;
#29538=DIRECTION ( 'NONE',  ( -2.775557561562891351E-16, -0.7071067811865477948, -0.7071067811865473507 ) ) ;
#29545=ADVANCED_FACE ( 'NONE', ( #7342 ), #10426, .F. ) ;
#29546=ORIENTED_EDGE ( 'NONE', *, *, #13705, .T. ) ;
#29556=ADVANCED_FACE ( 'NONE', ( #30695 ), #18862, .T. ) ;
#29564=EDGE_CURVE ( 'NONE', #586, #49298, #2226, .T. ) ;
#29573=LINE ( 'NONE', #17523, #38665 ) ;
#29575=AXIS2_PLACEMENT_3D ( 'NONE', #46521, #11411, #23206 ) ;
#29578=ADVANCED_FACE ( 'NONE', ( #49129 ), #26336, .T. ) ;
#29581=CARTESIAN_POINT ( 'NONE',  ( 355.9999999999999432, -174.9999999999999432, 355.9999999999998295 ) ) ;
#29582=ORIENTED_EDGE ( 'NONE', *, *, #45015, .F. ) ;
#29585=DIRECTION ( 'NONE',  ( -1.000000000000000000, 0.000000000000000000, 0.000000000000000000 ) ) ;
#29594=EDGE_LOOP ( 'NONE', ( #9847, #36172, #38157, #36423 ) ) ;
#29599=EDGE_CURVE ( 'NONE', #26176, #19710, #41473, .T. ) ;
#29602=ORIENTED_EDGE ( 'NONE', *, *, #48355, .F. ) ;
#29609=ADVANCED_FACE ( 'NONE', ( #34287 ), #34044, .F. ) ;
#29615=DIRECTION ( 'NONE',  ( 0.000000000000000000, 0.000000000000000000, 1.000000000000000000 ) ) ;
#29620=VERTEX_POINT ( 'NONE', #10675 ) ;
#29628=CARTESIAN_POINT ( 'NONE',  ( 0.000000000000000000, 169.0000000000000000, 357.9999999999997726 ) ) ;
#29636=ADVANCED_FACE ( 'NONE', ( #15303, #9052 ), #47996, .F. ) ;
#29644=EDGE_CURVE ( 'NONE', #2629, #29259, #34573, .T. ) ;
#29647=ORIENTED_EDGE ( 'NONE', *, *, #30240, .T. ) ;
#29648=DIRECTION ( 'NONE',  ( 0.000000000000000000, -1.000000000000000000, -1.544785076050074834E-48 ) ) ;
#29651=FACE_OUTER_BOUND ( 'NONE', #13447, .T. ) ;
#29653=ORIENTED_EDGE ( 'NONE', *, *, #36982, .T. ) ;
#29662=VERTEX_POINT ( 'NONE', #13140 ) ;
#29671=DIRECTION ( 'NONE',  ( -1.000000000000000000, 0.000000000000000000, -1.612977847700450206E-50 ) ) ;
#29676=EDGE_LOOP ( 'NONE', ( #14456, #33186, #36720, #47968 ) ) ;
#29677=DIRECTION ( 'NONE',  ( -0.000000000000000000, -1.000000000000000000, 2.537652627714643577E-15 ) ) ;
#29678=ADVANCED_FACE ( 'NONE', ( #23756 ), #28801, .F. ) ;
#29688=DIRECTION ( 'NONE',  ( -1.586032892321652236E-16, -1.000000000000000000, -6.853681917100419162E-49 ) ) ;
#29690=CIRCLE ( 'NONE', #32158, 4.000000000000003553 ) ;
#29705=ADVANCED_FACE ( 'NONE', ( #9295 ), #9549, .T. ) ;
#29707=ORIENTED_EDGE ( 'NONE', *, *, #24296, .F. ) ;
#29712=DIRECTION ( 'NONE',  ( -0.000000000000000000, 1.000000000000000000, 0.000000000000000000 ) ) ;
#29718=CARTESIAN_POINT ( 'NONE',  ( 181.0000000000000000, -268.4999999999999432, -349.9999999999999432 ) ) ;
#29722=DIRECTION ( 'NONE',  ( -1.000000000000000000, 0.000000000000000000, 0.000000000000000000 ) ) ;
#29723=VERTEX_POINT ( 'NONE', #32917 ) ;
#29725=DIRECTION ( 'NONE',  ( 0.000000000000000000, -1.000000000000000000, 0.000000000000000000 ) ) ;
#29728=CARTESIAN_POINT ( 'NONE',  ( 164.9999999999999716, -272.4999999999999432, -343.9999999999999432 ) ) ;
#29729=AXIS2_PLACEMENT_3D ( 'NONE', #40101, #4433, #9047 ) ;
#29733=DIRECTION ( 'NONE',  ( 0.000000000000000000, -1.000000000000000000, 0.000000000000000000 ) ) ;
#29740=VERTEX_POINT ( 'NONE', #44666 ) ;
#29752=ORIENTED_EDGE ( 'NONE', *, *, #11084, .T. ) ;
#29753=DIRECTION ( 'NONE',  ( 0.000000000000000000, 0.000000000000000000, -1.000000000000000000 ) ) ;
#29755=CARTESIAN_POINT ( 'NONE',  ( 341.9999999999999432, 174.9999999999996589, -344.0000000000002842 ) ) ;
#29757=CARTESIAN_POINT ( 'NONE',  ( 164.9999999999999716, -268.5000000000000000, -339.9999999999998863 ) ) ;
#29765=DIRECTION ( 'NONE',  ( 0.000000000000000000, -2.537652627714643577E-15, -1.000000000000000000 ) ) ;
#29769=DIRECTION ( 'NONE',  ( 0.000000000000000000, 0.000000000000000000, 1.000000000000000000 ) ) ;
#29771=ADVANCED_FACE ( 'NONE', ( #33421 ), #29305, .T. ) ;
#29772=VERTEX_POINT ( 'NONE', #44910 ) ;
#29773=CARTESIAN_POINT ( 'NONE',  ( 181.0000000000000000, -184.9999999999999716, -350.0000000000001705 ) ) ;
#29776=AXIS2_PLACEMENT_3D ( 'NONE', #28466, #29461, #5090 ) ;
#29778=EDGE_CURVE ( 'NONE', #16880, #45973, #41100, .T. ) ;
#29780=AXIS2_PLACEMENT_3D ( 'NONE', #8872, #44257, #1194 ) ;
#29785=MECHANICAL_DESIGN_GEOMETRIC_PRESENTATION_REPRESENTATION('',(#12560),#32246);
#29790=CARTESIAN_POINT ( 'NONE',  ( 340.0000000000000568, 166.6568542494923975, 341.6568542494921417 ) ) ;
#29791=CARTESIAN_POINT ( 'NONE',  ( 0.000000000000000000, -175.0000000000000284, 350.0000000000002274 ) ) ;
#29809=DIRECTION ( 'NONE',  ( 4.996003610813203446E-16, 1.000000000000000000, 0.000000000000000000 ) ) ;
#29813=AXIS2_PLACEMENT_3D ( 'NONE', #10785, #42580, #30296 ) ;
#29821=DIRECTION ( 'NONE',  ( -1.000000000000000000, 1.586032997072805650E-16, 4.759647537211363479E-16 ) ) ;
#29827=DIRECTION ( 'NONE',  ( -1.000000000000000000, 0.000000000000000000, -7.793956916774525800E-48 ) ) ;
#29839=VERTEX_POINT ( 'NONE', #36431 ) ;
#29852=AXIS2_PLACEMENT_3D ( 'NONE', #11551, #7960, #28212 ) ;
#29859=ORIENTED_EDGE ( 'NONE', *, *, #33199, .F. ) ;
#29862=PLANE ( 'NONE',  #10028 ) ;
#29868=AXIS2_PLACEMENT_3D ( 'NONE', #26479, #41625, #2372 ) ;
#29874=ORIENTED_EDGE ( 'NONE', *, *, #27321, .T. ) ;
#29891=EDGE_CURVE ( 'NONE', #35576, #2845, #1518, .T. ) ;
#29893=CARTESIAN_POINT ( 'NONE',  ( 350.0000000000001137, 181.0000000000000284, 343.9999999999997726 ) ) ;
#29901=ADVANCED_FACE ( 'NONE', ( #17161 ), #13297, .T. ) ;
#29903=AXIS2_PLACEMENT_3D ( 'NONE', #42451, #3717, #42958 ) ;
#29908=DIRECTION ( 'NONE',  ( -2.958228394578793832E-31, 0.000000000000000000, -1.000000000000000000 ) ) ;
#29911=DIRECTION ( 'NONE',  ( 0.000000000000000000, 0.000000000000000000, -1.000000000000000000 ) ) ;
#29916=VECTOR ( 'NONE', #43548, 1000.000000000000000 ) ;
#29918=ORIENTED_EDGE ( 'NONE', *, *, #42103, .T. ) ;
#29924=VECTOR ( 'NONE', #29821, 1000.000000000000000 ) ;
#29927=DIRECTION ( 'NONE',  ( 0.000000000000000000, 2.969158215481698263E-48, -1.000000000000000000 ) ) ;
#29936=CARTESIAN_POINT ( 'NONE',  ( 0.000000000000000000, 169.0000000000000000, -342.0000000000001705 ) ) ;
#29953=CIRCLE ( 'NONE', #49562, 2.000000000000001776 ) ;
#29959=ADVANCED_FACE ( 'NONE', ( #12545 ), #4841, .F. ) ;
#29961=VECTOR ( 'NONE', #29242, 1000.000000000000000 ) ;
#29971=VERTEX_POINT ( 'NONE', #14856 ) ;
#29972=CARTESIAN_POINT ( 'NONE',  ( 168.9999999999999716, -184.9999999999999716, -356.0000000000001705 ) ) ;
#29973=FACE_OUTER_BOUND ( 'NONE', #11203, .T. ) ;
#29974=LINE ( 'NONE', #46078, #22368 ) ;
#29979=ORIENTED_EDGE ( 'NONE', *, *, #18583, .T. ) ;
#29989=VECTOR ( 'NONE', #29385, 1000.000000000000000 ) ;
#29995=STYLED_ITEM('',(#50747),#22914);
#30001=ORIENTED_EDGE ( 'NONE', *, *, #8751, .T. ) ;
#30003=ORIENTED_EDGE ( 'NONE', *, *, #40965, .T. ) ;
#30004=ORIENTED_EDGE ( 'NONE', *, *, #6024, .T. ) ;
#30015=EDGE_LOOP ( 'NONE', ( #38003, #6914, #41156, #48374 ) ) ;
#30018=( NAMED_UNIT ( * ) PLANE_ANGLE_UNIT ( ) SI_UNIT ( $, .RADIAN. ) );
#30019=ADVANCED_FACE ( 'NONE', ( #13825 ), #2545, .F. ) ;
#30026=AXIS2_PLACEMENT_3D ( 'NONE', #20333, #4182, #345 ) ;
#30028=CARTESIAN_POINT ( 'NONE',  ( 342.0000000000000000, -2.999999999999919176, 171.9999999999998295 ) ) ;
#30052=PLANE ( 'NONE',  #29813 ) ;
#30053=CARTESIAN_POINT ( 'NONE',  ( 0.000000000000000000, 184.8000000000000114, 359.7999999999997840 ) ) ;
#30058=LINE ( 'NONE', #30302, #43945 ) ;
#30071=EDGE_CURVE ( 'NONE', #8815, #14722, #2793, .T. ) ;
#30081=ORIENTED_EDGE ( 'NONE', *, *, #38139, .F. ) ;
#30082=VECTOR ( 'NONE', #30627, 1000.000000000000000 ) ;
#30086=FACE_OUTER_BOUND ( 'NONE', #7070, .T. ) ;
#30089=CARTESIAN_POINT ( 'NONE',  ( 359.9999999999999432, -169.0000000000001705, 344.0000000000000000 ) ) ;
#30090=LINE ( 'NONE', #38308, #11692 ) ;
#30092=LINE ( 'NONE', #41122, #19818 ) ;
#30095=DIRECTION ( 'NONE',  ( -1.132880637372608740E-16, -4.718402560806925739E-50, -1.000000000000000000 ) ) ;
#30096=CIRCLE ( 'NONE', #11297, 4.000000000000003553 ) ;
#30105=ORIENTED_EDGE ( 'NONE', *, *, #36352, .F. ) ;
#30106=DIRECTION ( 'NONE',  ( -1.000000000000000000, 0.000000000000000000, -1.612977847700450206E-50 ) ) ;
#30111=FACE_OUTER_BOUND ( 'NONE', #31194, .T. ) ;
#30112=EDGE_LOOP ( 'NONE', ( #46998, #25788, #42136, #15497 ) ) ;
#30117=EDGE_LOOP ( 'NONE', ( #28874, #2764, #24946, #5300, #6601, #33637, #39596, #36313 ) ) ;
#30119=ORIENTED_EDGE ( 'NONE', *, *, #2080, .T. ) ;
#30120=LINE ( 'NONE', #38850, #22575 ) ;
#30129=ORIENTED_EDGE ( 'NONE', *, *, #23028, .T. ) ;
#30134=ORIENTED_EDGE ( 'NONE', *, *, #7173, .F. ) ;
#30135=CARTESIAN_POINT ( 'NONE',  ( 350.0000000000000000, -164.9999999999999432, 343.9999999999997726 ) ) ;
#30137=CARTESIAN_POINT ( 'NONE',  ( 183.0000000000000284, -174.9999999999999716, -111.0000000000001563 ) ) ;
#30143=CIRCLE ( 'NONE', #25232, 4.000000000000003553 ) ;
#30151=ADVANCED_FACE ( 'NONE', ( #27674 ), #23830, .T. ) ;
#30152=VERTEX_POINT ( 'NONE', #8180 ) ;
#30157=CARTESIAN_POINT ( 'NONE',  ( 168.9999999999999716, -93.49999999999998579, -350.0000000000001705 ) ) ;
#30158=FACE_BOUND ( 'NONE', #12174, .T. ) ;
#30162=DIRECTION ( 'NONE',  ( 0.000000000000000000, -1.000000000000000000, -1.544785076050074834E-48 ) ) ;
#30163=ORIENTED_EDGE ( 'NONE', *, *, #29405, .T. ) ;
#30168=ORIENTED_EDGE ( 'NONE', *, *, #10588, .F. ) ;
#30169=ORIENTED_EDGE ( 'NONE', *, *, #34567, .F. ) ;
#30175=DIRECTION ( 'NONE',  ( 0.000000000000000000, 0.000000000000000000, 1.000000000000000000 ) ) ;
#30176=LINE ( 'NONE', #41981, #49871 ) ;
#30184=DIRECTION ( 'NONE',  ( 0.000000000000000000, -2.537652627714643577E-15, -1.000000000000000000 ) ) ;
#30185=FACE_OUTER_BOUND ( 'NONE', #44976, .T. ) ;
#30191=CYLINDRICAL_SURFACE ( 'NONE', #47204, 4.000000000000003553 ) ;
#30192=EDGE_CURVE ( 'NONE', #6937, #11052, #11519, .T. ) ;
#30194=LINE ( 'NONE', #42496, #50190 ) ;
#30197=CLOSED_SHELL ( 'NONE', ( #20860, #19897, #4556, #14867, #50100, #917, #2749, #49607, #17385, #33103, #21764, #36085, #23955, #44661, #13928, #12733, #10558, #50676 ) ) ;
#30200=DIRECTION ( 'NONE',  ( 1.000000000000000000, -4.758098676964957447E-16, -1.586032892321651989E-16 ) ) ;
#30203=DIRECTION ( 'NONE',  ( -1.000000000000000000, -0.000000000000000000, -0.000000000000000000 ) ) ;
#30208=ORIENTED_EDGE ( 'NONE', *, *, #38542, .T. ) ;
#30209=ADVANCED_FACE ( 'NONE', ( #40491, #25094 ), #728, .T. ) ;
#30218=ORIENTED_EDGE ( 'NONE', *, *, #31588, .T. ) ;
#30226=CARTESIAN_POINT ( 'NONE',  ( -5.000000000000000000, 175.0000000000000284, 350.0000000000002274 ) ) ;
#30228=CARTESIAN_POINT ( 'NONE',  ( 181.0000000000000000, -5.999999999999950262, 339.9999999999998295 ) ) ;
#30229=AXIS2_PLACEMENT_3D ( 'NONE', #44620, #32101, #12583 ) ;
#30231=PLANE ( 'NONE',  #1026 ) ;
#30233=AXIS2_PLACEMENT_3D ( 'NONE', #15174, #31083, #19262 ) ;
#30240=EDGE_CURVE ( 'NONE', #36302, #24372, #20774, .T. ) ;
#30245=ORIENTED_EDGE ( 'NONE', *, *, #22812, .T. ) ;
#30246=APPLICATION_CONTEXT ( 'automotive_design' ) ;
#30256=CARTESIAN_POINT ( 'NONE',  ( 356.0000000000001137, 165.0000000000000000, 339.9999999999998295 ) ) ;
#30257=CARTESIAN_POINT ( 'NONE',  ( 343.9999999999994316, 183.0000000000000284, -358.0000000000001705 ) ) ;
#30266=VECTOR ( 'NONE', #31877, 1000.000000000000000 ) ;
#30269=AXIS2_PLACEMENT_3D ( 'NONE', #2381, #45700, #41635 ) ;
#30272=CARTESIAN_POINT ( 'NONE',  ( 339.9999999999998863, -168.9999999999999432, 343.9999999999997726 ) ) ;
#30285=EDGE_CURVE ( 'NONE', #19835, #34493, #20726, .T. ) ;
#30296=DIRECTION ( 'NONE',  ( 0.000000000000000000, 1.000000000000000000, -2.537652627714642000E-15 ) ) ;
#30297=ORIENTED_EDGE ( 'NONE', *, *, #49715, .F. ) ;
#30300=EDGE_LOOP ( 'NONE', ( #45138, #38630, #30582, #4860 ) ) ;
#30302=CARTESIAN_POINT ( 'NONE',  ( 0.000000000000000000, 183.0000000000000284, -356.0000000000002274 ) ) ;
#30304=AXIS2_PLACEMENT_3D ( 'NONE', #29521, #18710, #10023 ) ;
#30305=ORIENTED_EDGE ( 'NONE', *, *, #21182, .T. ) ;
#30312=AXIS2_PLACEMENT_3D ( 'NONE', #11314, #19502, #15417 ) ;
#30334=DIRECTION ( 'NONE',  ( 0.000000000000000000, -1.000000000000000000, 0.000000000000000000 ) ) ;
#30336=DIRECTION ( 'NONE',  ( 0.000000000000000000, 0.000000000000000000, 1.000000000000000000 ) ) ;
#30338=VECTOR ( 'NONE', #11352, 1000.000000000000000 ) ;
#30339=EDGE_CURVE ( 'NONE', #21405, #34478, #45304, .T. ) ;
#30346=ORIENTED_EDGE ( 'NONE', *, *, #47426, .T. ) ;
#30349=LINE ( 'NONE', #26751, #6922 ) ;
#30350=CIRCLE ( 'NONE', #22144, 2.000000000000001776 ) ;
#30354=EDGE_CURVE ( 'NONE', #37052, #23178, #41551, .T. ) ;
#30356=CARTESIAN_POINT ( 'NONE',  ( 0.000000000000000000, -168.9999999999999432, -342.0000000000001705 ) ) ;
#30359=CARTESIAN_POINT ( 'NONE',  ( 166.9999999999999716, -256.4999999999993179, -114.9999999999999574 ) ) ;
#30361=EDGE_CURVE ( 'NONE', #2551, #12862, #30096, .T. ) ;
#30362=EDGE_LOOP ( 'NONE', ( #1011, #43525, #26589, #42132 ) ) ;
#30368=ORIENTED_EDGE ( 'NONE', *, *, #11144, .F. ) ;
#30390=ORIENTED_EDGE ( 'NONE', *, *, #38792, .T. ) ;
#30391=EDGE_CURVE ( 'NONE', #14610, #44239, #46451, .T. ) ;
#30397=EDGE_LOOP ( 'NONE', ( #22651, #27374, #28347, #43745 ) ) ;
#30399=CARTESIAN_POINT ( 'NONE',  ( 166.9999999999999716, 165.0000000000000000, -356.0000000000001705 ) ) ;
#30400=CARTESIAN_POINT ( 'NONE',  ( 185.0000000000000000, -180.9999999999999716, -350.0000000000001705 ) ) ;
#30402=DIRECTION ( 'NONE',  ( -1.586032880504786307E-16, 1.654361225106055350E-24, -1.000000000000000000 ) ) ;
#30405=FACE_OUTER_BOUND ( 'NONE', #40322, .T. ) ;
#30412=CARTESIAN_POINT ( 'NONE',  ( 181.0000000000000000, -79.49999999999995737, -115.0000000000001563 ) ) ;
#30415=DIRECTION ( 'NONE',  ( -1.000000000000000000, 0.000000000000000000, 0.000000000000000000 ) ) ;
#30418=ORIENTED_EDGE ( 'NONE', *, *, #4346, .T. ) ;
#30424=DIRECTION ( 'NONE',  ( -1.860490536778032451E-50, 0.000000000000000000, -1.000000000000000000 ) ) ;
#30430=DIRECTION ( 'NONE',  ( 1.000000000000000000, 0.000000000000000000, 0.000000000000000000 ) ) ;
#30443=ORIENTED_EDGE ( 'NONE', *, *, #41222, .F. ) ;
#30448=CARTESIAN_POINT ( 'NONE',  ( 350.0000000000001137, 183.0000000000000284, 343.9999999999997726 ) ) ;
#30450=DIRECTION ( 'NONE',  ( 1.000000000000000000, 0.000000000000000000, -1.586032892321652482E-16 ) ) ;
#30452=VERTEX_POINT ( 'NONE', #2488 ) ;
#30454=CARTESIAN_POINT ( 'NONE',  ( 344.0000000000000000, -164.9999999999999432, 339.9999999999998295 ) ) ;
#30459=LINE ( 'NONE', #30723, #10949 ) ;
#30460=ORIENTED_EDGE ( 'NONE', *, *, #26775, .T. ) ;
#30474=VERTEX_POINT ( 'NONE', #33803 ) ;
#30477=ORIENTED_EDGE ( 'NONE', *, *, #21907, .T. ) ;
#30492=ORIENTED_EDGE ( 'NONE', *, *, #14284, .F. ) ;
#30494=PLANE ( 'NONE',  #41696 ) ;
#30502=ORIENTED_EDGE ( 'NONE', *, *, #4826, .T. ) ;
#30507=DIRECTION ( 'NONE',  ( -3.364279341222519273E-16, 0.7071067811865474617, -0.7071067811865476838 ) ) ;
#30512=AXIS2_PLACEMENT_3D ( 'NONE', #9308, #6457, #17510 ) ;
#30517=CARTESIAN_POINT ( 'NONE',  ( 350.0000000000000000, -180.9999999999999716, -342.0000000000001705 ) ) ;
#30529=EDGE_LOOP ( 'NONE', ( #44788, #24047, #38919, #46715 ) ) ;
#30539=VECTOR ( 'NONE', #48987, 1000.000000000000000 ) ;
#30540=VERTEX_POINT ( 'NONE', #50407 ) ;
#30541=DIRECTION ( 'NONE',  ( 0.000000000000000000, 2.969158215481698263E-48, -1.000000000000000000 ) ) ;
#30543=EDGE_CURVE ( 'NONE', #48807, #7917, #29323, .T. ) ;
#30547=DIRECTION ( 'NONE',  ( 0.000000000000000000, -1.000000000000000000, 2.537652627714642000E-15 ) ) ;
#30554=VERTEX_POINT ( 'NONE', #8125 ) ;
#30559=ORIENTED_EDGE ( 'NONE', *, *, #4042, .T. ) ;
#30567=EDGE_CURVE ( 'NONE', #40195, #9063, #42485, .T. ) ;
#30570=FACE_OUTER_BOUND ( 'NONE', #40458, .T. ) ;
#30571=CARTESIAN_POINT ( 'NONE',  ( 168.9999999999999716, -164.9999999999999432, -350.0000000000001705 ) ) ;
#30572=CYLINDRICAL_SURFACE ( 'NONE', #24643, 2.000000000000001776 ) ;
#30580=CARTESIAN_POINT ( 'NONE',  ( 169.0000000000000000, 2.775557561562891351E-14, -99.00000000000014211 ) ) ;
#30582=ORIENTED_EDGE ( 'NONE', *, *, #24918, .F. ) ;
#30587=CIRCLE ( 'NONE', #39719, 4.000000000000003553 ) ;
#30588=FACE_OUTER_BOUND ( 'NONE', #11368, .T. ) ;
#30595=VECTOR ( 'NONE', #2818, 1000.000000000000000 ) ;
#30596=ADVANCED_FACE ( 'NONE', ( #5013 ), #9124, .F. ) ;
#30603=CARTESIAN_POINT ( 'NONE',  ( 343.9999999999999432, -185.0000000000001421, 360.0000000000001137 ) ) ;
#30609=ORIENTED_EDGE ( 'NONE', *, *, #13012, .T. ) ;
#30615=ORIENTED_EDGE ( 'NONE', *, *, #43218, .T. ) ;
#30616=VERTEX_POINT ( 'NONE', #20160 ) ;
#30624=CARTESIAN_POINT ( 'NONE',  ( 342.8284271247462698, 167.0000000000000000, 341.9999999999998863 ) ) ;
#30627=DIRECTION ( 'NONE',  ( -1.586032892321652236E-16, -1.000000000000000000, -2.288264760618012091E-48 ) ) ;
#30628=VECTOR ( 'NONE', #27183, 1000.000000000000000 ) ;
#30629=EDGE_LOOP ( 'NONE', ( #50678, #31988, #28079, #14485 ) ) ;
#30630=CARTESIAN_POINT ( 'NONE',  ( 350.0000000000001137, 181.0000000000000284, 355.9999999999997726 ) ) ;
#30632=VECTOR ( 'NONE', #17936, 1000.000000000000000 ) ;
#30653=DIRECTION ( 'NONE',  ( 1.000000000000000000, 0.000000000000000000, 0.000000000000000000 ) ) ;
#30655=CARTESIAN_POINT ( 'NONE',  ( 0.000000000000000000, 181.0000000000000284, 341.9999999999997726 ) ) ;
#30660=CARTESIAN_POINT ( 'NONE',  ( -5.000000000000000000, -184.7999999999999545, 359.7999999999997840 ) ) ;
#30664=VECTOR ( 'NONE', #25069, 1000.000000000000000 ) ;
#30665=FACE_OUTER_BOUND ( 'NONE', #16178, .T. ) ;
#30666=AXIS2_PLACEMENT_3D ( 'NONE', #5755, #36839, #29615 ) ;
#30667=CARTESIAN_POINT ( 'NONE',  ( 167.0000000000000284, 175.0000000000000284, 355.9999999999998863 ) ) ;
#30669=VECTOR ( 'NONE', #12237, 1000.000000000000000 ) ;
#30676=EDGE_LOOP ( 'NONE', ( #5153, #46016, #15571, #39408 ) ) ;
#30678=EDGE_LOOP ( 'NONE', ( #10869, #36050, #43095, #45747, #49617, #48978, #9511, #17688 ) ) ;
#30679=LINE ( 'NONE', #7073, #11145 ) ;
#30682=AXIS2_PLACEMENT_3D ( 'NONE', #40855, #5702, #10062 ) ;
#30684=ORIENTED_EDGE ( 'NONE', *, *, #8028, .F. ) ;
#30692=LINE ( 'NONE', #27090, #10364 ) ;
#30695=FACE_OUTER_BOUND ( 'NONE', #8593, .T. ) ;
#30696=ADVANCED_FACE ( 'NONE', ( #40178 ), #17322, .F. ) ;
#30699=AXIS2_PLACEMENT_3D ( 'NONE', #47494, #14072, #13133 ) ;
#30700=ORIENTED_EDGE ( 'NONE', *, *, #42110, .F. ) ;
#30703=DIRECTION ( 'NONE',  ( 0.000000000000000000, -0.000000000000000000, 1.000000000000000000 ) ) ;
#30707=ORIENTED_EDGE ( 'NONE', *, *, #11067, .F. ) ;
#30716=CARTESIAN_POINT ( 'NONE',  ( 344.0000000000000000, -169.0000000000001137, -349.9999999999998863 ) ) ;
#30718=DIRECTION ( 'NONE',  ( 0.000000000000000000, 1.000000000000000000, -2.537652627714643577E-15 ) ) ;
#30723=CARTESIAN_POINT ( 'NONE',  ( 355.9999999999998295, -165.0000000000001137, -110.0000000000002132 ) ) ;
#30735=CARTESIAN_POINT ( 'NONE',  ( 349.9999999999999432, -180.9999999999999716, 343.9999999999997726 ) ) ;
#30736=DIRECTION ( 'NONE',  ( -1.000000000000000000, 4.996003610813203446E-16, 7.930164450086814785E-16 ) ) ;
#30742=VECTOR ( 'NONE', #22183, 1000.000000000000000 ) ;
#30746=VERTEX_POINT ( 'NONE', #49581 ) ;
#30747=CARTESIAN_POINT ( 'NONE',  ( 360.0000000000000000, -165.0000000000001137, -94.00000000000019895 ) ) ;
#30751=ORIENTED_EDGE ( 'NONE', *, *, #16465, .F. ) ;
#30756=ORIENTED_EDGE ( 'NONE', *, *, #4186, .T. ) ;
#30764=AXIS2_PLACEMENT_3D ( 'NONE', #12099, #27245, #39559 ) ;
#30785=LINE ( 'NONE', #19207, #50226 ) ;
#30789=DIRECTION ( 'NONE',  ( -1.586032892321651989E-16, -1.194346094642793337E-32, -1.000000000000000000 ) ) ;
#30791=CARTESIAN_POINT ( 'NONE',  ( 355.9999999999999432, -183.0000000000001421, 358.0000000000001705 ) ) ;
#30792=DIRECTION ( 'NONE',  ( 0.000000000000000000, -1.000000000000000000, -3.186989995019654210E-49 ) ) ;
#30793=ORIENTED_EDGE ( 'NONE', *, *, #37131, .F. ) ;
#30800=PLANE ( 'NONE',  #7424 ) ;
#30809=CARTESIAN_POINT ( 'NONE',  ( 168.9999999999999716, -77.49999999999997158, -350.0000000000001705 ) ) ;
#30812=LINE ( 'NONE', #3334, #43920 ) ;
#30817=AXIS2_PLACEMENT_3D ( 'NONE', #21644, #36822, #41141 ) ;
#30820=ORIENTED_EDGE ( 'NONE', *, *, #7027, .T. ) ;
#30827=ORIENTED_EDGE ( 'NONE', *, *, #189, .T. ) ;
#30833=VECTOR ( 'NONE', #46424, 1000.000000000000000 ) ;
#30843=ORIENTED_EDGE ( 'NONE', *, *, #14058, .F. ) ;
#30845=ADVANCED_FACE ( 'NONE', ( #13470 ), #9873, .T. ) ;
#30853=DIRECTION ( 'NONE',  ( 0.000000000000000000, 5.664403186863042467E-17, 1.000000000000000000 ) ) ;
#30855=ADVANCED_FACE ( 'NONE', ( #45245 ), #10125, .T. ) ;
#30858=VECTOR ( 'NONE', #9287, 1000.000000000000000 ) ;
#30860=DIRECTION ( 'NONE',  ( -1.000000000000000000, 0.000000000000000000, 0.000000000000000000 ) ) ;
#30861=ORIENTED_EDGE ( 'NONE', *, *, #13656, .T. ) ;
#30862=CARTESIAN_POINT ( 'NONE',  ( 341.6568542494922553, 165.0000000000001705, -340.0000000000002842 ) ) ;
#30867=EDGE_CURVE ( 'NONE', #13154, #38075, #3946, .T. ) ;
#30868=LINE ( 'NONE', #46458, #47626 ) ;
#30877=CARTESIAN_POINT ( 'NONE',  ( 181.0000000000000568, 165.0000000000000000, 341.9999999999998863 ) ) ;
#30879=CARTESIAN_POINT ( 'NONE',  ( 181.0000000000000000, 175.0000000000000284, -340.0000000000001137 ) ) ;
#30881=CARTESIAN_POINT ( 'NONE',  ( 342.0000000000000568, 169.0000000000000000, 349.9999999999998863 ) ) ;
#30886=DIRECTION ( 'NONE',  ( 1.000000000000000000, -4.758098676964957447E-16, 2.958228394578795584E-31 ) ) ;
#30891=ORIENTED_EDGE ( 'NONE', *, *, #31009, .T. ) ;
#30896=CIRCLE ( 'NONE', #22666, 2.000000000000001776 ) ;
#30900=EDGE_LOOP ( 'NONE', ( #13117, #26769, #30954, #15385 ) ) ;
#30908=ORIENTED_EDGE ( 'NONE', *, *, #19035, .F. ) ;
#30911=ADVANCED_FACE ( 'NONE', ( #28312, #11910 ), #43949, .F. ) ;
#30913=ORIENTED_EDGE ( 'NONE', *, *, #14284, .T. ) ;
#30942=EDGE_LOOP ( 'NONE', ( #22933, #41847, #3268, #36742, #42402, #31897, #14087, #11136 ) ) ;
#30954=ORIENTED_EDGE ( 'NONE', *, *, #32505, .F. ) ;
#30955=CARTESIAN_POINT ( 'NONE',  ( 166.9999999999999716, -174.9999999999999716, -344.0000000000001137 ) ) ;
#30956=CARTESIAN_POINT ( 'NONE',  ( 339.9999999999999432, -164.9999999999999432, -356.0000000000002274 ) ) ;
#30960=CARTESIAN_POINT ( 'NONE',  ( 167.0000000000000000, -174.9999999999999716, -111.0000000000001563 ) ) ;
#30966=LINE ( 'NONE', #16064, #5221 ) ;
#30971=LINE ( 'NONE', #4268, #42726 ) ;
#30972=DIRECTION ( 'NONE',  ( 0.000000000000000000, 0.000000000000000000, 1.000000000000000000 ) ) ;
#30978=PLANE ( 'NONE',  #19103 ) ;
#30986=CARTESIAN_POINT ( 'NONE',  ( 344.0000000000001705, 167.0000000000000000, -342.0000000000001137 ) ) ;
#30988=VERTEX_POINT ( 'NONE', #23707 ) ;
#30989=EDGE_CURVE ( 'NONE', #36488, #30988, #19844, .T. ) ;
#31009=EDGE_CURVE ( 'NONE', #44375, #30554, #6464, .T. ) ;
#31014=LINE ( 'NONE', #31523, #22584 ) ;
#31027=CARTESIAN_POINT ( 'NONE',  ( 181.0000000000000000, -81.49999999999997158, -350.0000000000001705 ) ) ;
#31039=DIRECTION ( 'NONE',  ( -1.000000000000000000, 0.000000000000000000, -7.793956916774525800E-48 ) ) ;
#31041=CARTESIAN_POINT ( 'NONE',  ( 181.0000000000000000, -164.9999999999999432, 359.9999999999997726 ) ) ;
#31045=LINE ( 'NONE', #43834, #11530 ) ;
#31047=ORIENTED_EDGE ( 'NONE', *, *, #37602, .F. ) ;
#31052=DIRECTION ( 'NONE',  ( 1.132880637372608740E-16, 4.718402560806925739E-50, 1.000000000000000000 ) ) ;
#31053=DIRECTION ( 'NONE',  ( -1.612977847700450206E-50, 0.000000000000000000, -1.000000000000000000 ) ) ;
#31064=CARTESIAN_POINT ( 'NONE',  ( 356.0000000000000568, -183.0000000000001421, 358.0000000000001705 ) ) ;
#31068=CARTESIAN_POINT ( 'NONE',  ( 357.9999999999999432, 181.0000000000002558, -356.0000000000003411 ) ) ;
#31069=ORIENTED_EDGE ( 'NONE', *, *, #29090, .T. ) ;
#31074=CARTESIAN_POINT ( 'NONE',  ( 185.0000000000000000, -93.49999999999998579, -115.0000000000001563 ) ) ;
#31075=ORIENTED_EDGE ( 'NONE', *, *, #44953, .T. ) ;
#31083=DIRECTION ( 'NONE',  ( 1.000000000000000000, 0.000000000000000000, 2.958228394578794270E-31 ) ) ;
#31089=VERTEX_POINT ( 'NONE', #44932 ) ;
#31098=DIRECTION ( 'NONE',  ( 0.000000000000000000, 0.000000000000000000, 1.000000000000000000 ) ) ;
#31109=VECTOR ( 'NONE', #28720, 1000.000000000000000 ) ;
#31116=ORIENTED_EDGE ( 'NONE', *, *, #33825, .T. ) ;
#31119=UNCERTAINTY_MEASURE_WITH_UNIT (LENGTH_MEASURE( 1.000000000000000082E-05 ), #19591, 'distance_accuracy_value', 'NONE');
#31125=EDGE_LOOP ( 'NONE', ( #48244, #20921, #30134, #47113 ) ) ;
#31128=VECTOR ( 'NONE', #50620, 1000.000000000000000 ) ;
#31131=CYLINDRICAL_SURFACE ( 'NONE', #19206, 2.000000000000001776 ) ;
#31132=CARTESIAN_POINT ( 'NONE',  ( 181.0000000000000000, -168.9999999999999432, -340.0000000000001137 ) ) ;
#31133=CARTESIAN_POINT ( 'NONE',  ( 342.0000000000000568, 167.8284271247462129, 342.8284271247459856 ) ) ;
#31142=EDGE_CURVE ( 'NONE', #21789, #7928, #5460, .T. ) ;
#31143=DIRECTION ( 'NONE',  ( 1.000000000000000000, 0.000000000000000000, 0.000000000000000000 ) ) ;
#31154=AXIS2_PLACEMENT_3D ( 'NONE', #8902, #48361, #13500 ) ;
#31166=ORIENTED_EDGE ( 'NONE', *, *, #8134, .T. ) ;
#31174=DIRECTION ( 'NONE',  ( -1.000000000000000000, 0.000000000000000000, -1.612977847700450206E-50 ) ) ;
#31175=ORIENTED_EDGE ( 'NONE', *, *, #16465, .T. ) ;
#31184=LINE ( 'NONE', #19866, #47452 ) ;
#31185=DIRECTION ( 'NONE',  ( 0.000000000000000000, 1.000000000000000000, 0.000000000000000000 ) ) ;
#31191=DIRECTION ( 'NONE',  ( -1.612977847700450206E-50, 0.000000000000000000, -1.000000000000000000 ) ) ;
#31192=AXIS2_PLACEMENT_3D ( 'NONE', #29469, #21508, #41022 ) ;
#31193=CIRCLE ( 'NONE', #49150, 2.000000000000001776 ) ;
#31194=EDGE_LOOP ( 'NONE', ( #9309, #15860, #28749, #22163 ) ) ;
#31198=ORIENTED_EDGE ( 'NONE', *, *, #7409, .T. ) ;
#31200=VECTOR ( 'NONE', #41315, 1000.000000000000000 ) ;
#31203=CIRCLE ( 'NONE', #33651, 4.000000000000003553 ) ;
#31210=VERTEX_POINT ( 'NONE', #18761 ) ;
#31214=UNCERTAINTY_MEASURE_WITH_UNIT (LENGTH_MEASURE( 1.000000000000000082E-05 ), #46703, 'distance_accuracy_value', 'NONE');
#31221=ORIENTED_EDGE ( 'NONE', *, *, #11097, .T. ) ;
#31222=ADVANCED_FACE ( 'NONE', ( #23839, #39749 ), #34442, .T. ) ;
#31226=EDGE_CURVE ( 'NONE', #29259, #46163, #7231, .T. ) ;
#31228=EDGE_LOOP ( 'NONE', ( #45102, #5457, #12707, #38184 ) ) ;
#31230=DIRECTION ( 'NONE',  ( 1.000000000000000000, 0.000000000000000000, 0.000000000000000000 ) ) ;
#31233=DIRECTION ( 'NONE',  ( -1.586032892321652236E-16, -1.000000000000000000, -2.288264760618012091E-48 ) ) ;
#31243=ADVANCED_FACE ( 'NONE', ( #30086 ), #12276, .T. ) ;
#31248=LINE ( 'NONE', #46838, #29449 ) ;
#31255=DIRECTION ( 'NONE',  ( 0.000000000000000000, -1.000000000000000000, -1.544785076050074834E-48 ) ) ;
#31256=CARTESIAN_POINT ( 'NONE',  ( 350.0000000000001137, 183.0000000000000284, 343.9999999999997726 ) ) ;
#31260=ADVANCED_FACE ( 'NONE', ( #9436 ), #25101, .F. ) ;
#31261=VECTOR ( 'NONE', #18956, 1000.000000000000000 ) ;
#31268=ORIENTED_EDGE ( 'NONE', *, *, #43538, .T. ) ;
#31269=DIRECTION ( 'NONE',  ( -7.793956916774524585E-48, 0.000000000000000000, -1.000000000000000000 ) ) ;
#31278=VECTOR ( 'NONE', #32684, 1000.000000000000000 ) ;
#31282=DIRECTION ( 'NONE',  ( 0.000000000000000000, 1.000000000000000000, 0.000000000000000000 ) ) ;
#31287=LINE ( 'NONE', #16627, #17333 ) ;
#31293=CARTESIAN_POINT ( 'NONE',  ( 169.0000000000000000, -180.9999999999999716, -115.0000000000001279 ) ) ;
#31296=EDGE_CURVE ( 'NONE', #32935, #27742, #40025, .T. ) ;
#31301=ORIENTED_EDGE ( 'NONE', *, *, #47216, .T. ) ;
#31305=CARTESIAN_POINT ( 'NONE',  ( 0.000000000000000000, 185.0000000000000284, 343.9999999999997726 ) ) ;
#31310=ORIENTED_EDGE ( 'NONE', *, *, #24201, .F. ) ;
#31311=AXIS2_PLACEMENT_3D ( 'NONE', #29329, #37553, #21365 ) ;
#31316=ORIENTED_EDGE ( 'NONE', *, *, #43479, .F. ) ;
#31318=ORIENTED_EDGE ( 'NONE', *, *, #24892, .F. ) ;
#31327=DIRECTION ( 'NONE',  ( 4.758098676964956461E-16, 0.000000000000000000, 1.000000000000000000 ) ) ;
#31329=DIRECTION ( 'NONE',  ( 1.000000000000000000, 0.000000000000000000, 0.000000000000000000 ) ) ;
#31332=LINE ( 'NONE', #27973, #2393 ) ;
#31337=LINE ( 'NONE', #46927, #43138 ) ;
#31340=DIRECTION ( 'NONE',  ( 0.000000000000000000, -2.265761274745217480E-16, 1.000000000000000000 ) ) ;
#31345=VECTOR ( 'NONE', #24386, 1000.000000000000000 ) ;
#31358=CARTESIAN_POINT ( 'NONE',  ( 181.0000000000000000, -93.49999999999997158, -115.0000000000001563 ) ) ;
#31361=VECTOR ( 'NONE', #9718, 1000.000000000000000 ) ;
#31362=CARTESIAN_POINT ( 'NONE',  ( 0.000000000000000000, -184.7999999999999545, -359.8000000000002387 ) ) ;
#31365=ORIENTED_EDGE ( 'NONE', *, *, #9099, .T. ) ;
#31370=CARTESIAN_POINT ( 'NONE',  ( 339.9999999999998863, 174.9999999999996305, -356.0000000000003411 ) ) ;
#31371=EDGE_LOOP ( 'NONE', ( #23740, #21364, #40021, #14997 ) ) ;
#31373=AXIS2_PLACEMENT_3D ( 'NONE', #3939, #15740, #17006 ) ;
#31378=AXIS2_PLACEMENT_3D ( 'NONE', #3835, #46896, #20494 ) ;
#31381=CARTESIAN_POINT ( 'NONE',  ( 339.9999999999998863, -182.9999999999999716, 355.9999999999997726 ) ) ;
#31387=ORIENTED_EDGE ( 'NONE', *, *, #36278, .T. ) ;
#31390=ADVANCED_FACE ( 'NONE', ( #9941, #49401 ), #14800, .T. ) ;
#31391=EDGE_LOOP ( 'NONE', ( #28973, #43900, #44152, #18250 ) ) ;
#31395=DIRECTION ( 'NONE',  ( -1.000000000000000000, -0.000000000000000000, -0.000000000000000000 ) ) ;
#31397=DIRECTION ( 'NONE',  ( 0.000000000000000000, 0.000000000000000000, -1.000000000000000000 ) ) ;
#31404=VECTOR ( 'NONE', #36168, 1000.000000000000000 ) ;
#31406=CARTESIAN_POINT ( 'NONE',  ( 5.551115123125782702E-14, -180.9999999999999716, 359.9999999999997726 ) ) ;
#31412=ORIENTED_EDGE ( 'NONE', *, *, #11084, .F. ) ;
#31414=EDGE_LOOP ( 'NONE', ( #46209, #9167, #34224, #15482, #39379, #17314, #21205, #34670 ) ) ;
#31415=CARTESIAN_POINT ( 'NONE',  ( 360.0000000000000000, 181.0000000000000284, -356.0000000000001705 ) ) ;
#31418=CIRCLE ( 'NONE', #22380, 4.000000000000003553 ) ;
#31419=CARTESIAN_POINT ( 'NONE',  ( 356.0000000000000000, -167.0000000000001137, 341.9999999999999432 ) ) ;
#31424=CARTESIAN_POINT ( 'NONE',  ( 181.0000000000000284, -174.9999999999999716, -113.0000000000001563 ) ) ;
#31436=VECTOR ( 'NONE', #7461, 1000.000000000000000 ) ;
#31437=DIRECTION ( 'NONE',  ( -1.586032892321652236E-16, -1.000000000000000000, -6.853681917100419162E-49 ) ) ;
#31439=VECTOR ( 'NONE', #6407, 1000.000000000000000 ) ;
#31449=CARTESIAN_POINT ( 'NONE',  ( 181.0000000000000000, -5.999999999999950262, 339.9999999999998295 ) ) ;
#31456=AXIS2_PLACEMENT_3D ( 'NONE', #22674, #35262, #14982 ) ;
#31458=FACE_OUTER_BOUND ( 'NONE', #30300, .T. ) ;
#31459=FACE_OUTER_BOUND ( 'NONE', #23804, .T. ) ;
#31476=VECTOR ( 'NONE', #47100, 1000.000000000000000 ) ;
#31478=VERTEX_POINT ( 'NONE', #40993 ) ;
#31486=PLANE ( 'NONE',  #27164 ) ;
#31489=CARTESIAN_POINT ( 'NONE',  ( 358.0000000000000000, 175.0000000000000284, -106.0000000000001990 ) ) ;
#31491=DIRECTION ( 'NONE',  ( -1.612977847700450206E-50, 0.000000000000000000, -1.000000000000000000 ) ) ;
#31494=DIRECTION ( 'NONE',  ( 0.000000000000000000, -1.000000000000000000, -4.687818848539279227E-49 ) ) ;
#31495=CIRCLE ( 'NONE', #14252, 2.000000000000001776 ) ;
#31502=DIRECTION ( 'NONE',  ( 1.000000000000000000, 0.000000000000000000, 2.958228394578794708E-31 ) ) ;
#31506=VERTEX_POINT ( 'NONE', #18635 ) ;
#31507=CARTESIAN_POINT ( 'NONE',  ( 349.9999999999999432, -180.9999999999999716, 355.9999999999997726 ) ) ;
#31508=EDGE_CURVE ( 'NONE', #3587, #37149, #29442, .T. ) ;
#31509=EDGE_CURVE ( 'NONE', #586, #43206, #13778, .T. ) ;
#31514=AXIS2_PLACEMENT_3D ( 'NONE', #21650, #3146, #45473 ) ;
#31523=CARTESIAN_POINT ( 'NONE',  ( 344.0000000000000000, 165.0000000000000000, -90.00000000000018474 ) ) ;
#31537=CARTESIAN_POINT ( 'NONE',  ( 169.0000000000000284, 165.0000000000000000, 355.9999999999998863 ) ) ;
#31542=EDGE_CURVE ( 'NONE', #19831, #26993, #16077, .T. ) ;
#31547=LINE ( 'NONE', #3551, #25826 ) ;
#31552=CARTESIAN_POINT ( 'NONE',  ( 344.0000000000000568, 167.0000000000000000, 349.9999999999998863 ) ) ;
#31553=VECTOR ( 'NONE', #215, 1000.000000000000000 ) ;
#31555=DIRECTION ( 'NONE',  ( -0.000000000000000000, -0.000000000000000000, 1.000000000000000000 ) ) ;
#31556=EDGE_LOOP ( 'NONE', ( #49425, #27547, #31075, #13454 ) ) ;
#31558=DIRECTION ( 'NONE',  ( 1.000000000000000000, 0.000000000000000000, 2.958228394578794270E-31 ) ) ;
#31565=EDGE_LOOP ( 'NONE', ( #18443, #13796, #48916, #42240 ) ) ;
#31578=LINE ( 'NONE', #12065, #26998 ) ;
#31580=AXIS2_PLACEMENT_3D ( 'NONE', #16699, #21557, #48465 ) ;
#31582=CARTESIAN_POINT ( 'NONE',  ( 360.0000000000001137, 181.0000000000000284, 355.9999999999998295 ) ) ;
#31586=EDGE_CURVE ( 'NONE', #21707, #33352, #50583, .T. ) ;
#31587=CARTESIAN_POINT ( 'NONE',  ( 181.0000000000000000, -252.4999999999999432, -349.9999999999999432 ) ) ;
#31588=EDGE_CURVE ( 'NONE', #16652, #35927, #15567, .T. ) ;
#31589=CYLINDRICAL_SURFACE ( 'NONE', #39549, 4.000000000000003553 ) ;
#31591=FACE_OUTER_BOUND ( 'NONE', #35704, .T. ) ;
#31621=AXIS2_PLACEMENT_3D ( 'NONE', #27991, #11592, #38554 ) ;
#31623=CARTESIAN_POINT ( 'NONE',  ( 181.0000000000000000, 175.0000000000000284, -360.0000000000001705 ) ) ;
#31626=CARTESIAN_POINT ( 'NONE',  ( 344.0000000000000568, 167.0000000000000000, 349.9999999999998863 ) ) ;
#31628=DIRECTION ( 'NONE',  ( -0.000000000000000000, -0.000000000000000000, 1.000000000000000000 ) ) ;
#31636=VERTEX_POINT ( 'NONE', #47073 ) ;
#31638=EDGE_CURVE ( 'NONE', #16880, #42585, #47331, .T. ) ;
#31642=VERTEX_POINT ( 'NONE', #34566 ) ;
#31644=CARTESIAN_POINT ( 'NONE',  ( 356.0000000000000000, 165.0000000000000000, -110.0000000000002132 ) ) ;
#31659=CARTESIAN_POINT ( 'NONE',  ( 168.9999999999999716, -166.9999999999999432, -340.0000000000001137 ) ) ;
#31660=VERTEX_POINT ( 'NONE', #24292 ) ;
#31670=CARTESIAN_POINT ( 'NONE',  ( 343.9999999999999432, -183.0000000000001421, -358.0000000000003411 ) ) ;
#31677=DIRECTION ( 'NONE',  ( 1.586032892321651989E-16, 1.194346094642793337E-32, 1.000000000000000000 ) ) ;
#31683=LINE ( 'NONE', #24728, #25613 ) ;
#31685=ORIENTED_EDGE ( 'NONE', *, *, #28456, .F. ) ;
#31698=AXIS2_PLACEMENT_3D ( 'NONE', #12568, #42853, #16185 ) ;
#31701=AXIS2_PLACEMENT_3D ( 'NONE', #8865, #5520, #48827 ) ;
#31708=VECTOR ( 'NONE', #47102, 1000.000000000000000 ) ;
#31711=VERTEX_POINT ( 'NONE', #24032 ) ;
#31713=CARTESIAN_POINT ( 'NONE',  ( 168.9999999999999716, -252.4999999999999432, -339.9999999999998863 ) ) ;
#31715=LINE ( 'NONE', #4491, #12799 ) ;
#31718=VERTEX_POINT ( 'NONE', #40694 ) ;
#31726=ORIENTED_EDGE ( 'NONE', *, *, #22820, .F. ) ;
#31735=ORIENTED_EDGE ( 'NONE', *, *, #3526, .F. ) ;
#31745=AXIS2_PLACEMENT_3D ( 'NONE', #12140, #46477, #8548 ) ;
#31747=LINE ( 'NONE', #185, #946 ) ;
#31754=AXIS2_PLACEMENT_3D ( 'NONE', #2347, #17989, #1855 ) ;
#31756=ORIENTED_EDGE ( 'NONE', *, *, #4619, .T. ) ;
#31757=DIRECTION ( 'NONE',  ( -0.000000000000000000, -0.000000000000000000, 1.000000000000000000 ) ) ;
#31759=CARTESIAN_POINT ( 'NONE',  ( 350.0000000000000000, 169.0000000000000000, -340.0000000000001705 ) ) ;
#31760=ORIENTED_EDGE ( 'NONE', *, *, #24303, .T. ) ;
#31761=LINE ( 'NONE', #47346, #30669 ) ;
#31763=ORIENTED_EDGE ( 'NONE', *, *, #46859, .F. ) ;
#31767=CARTESIAN_POINT ( 'NONE',  ( 350.0000000000001137, 185.0000000000000284, 343.9999999999997726 ) ) ;
#31768=CARTESIAN_POINT ( 'NONE',  ( 344.0000000000000000, 165.0000000000001990, -340.0000000000002842 ) ) ;
#31778=CARTESIAN_POINT ( 'NONE',  ( 359.9999999999998295, -183.3431457505077731, 358.3431457505076310 ) ) ;
#31781=EDGE_LOOP ( 'NONE', ( #45360, #11741, #12981, #38719 ) ) ;
#31784=EDGE_CURVE ( 'NONE', #16304, #32679, #27976, .T. ) ;
#31788=DIRECTION ( 'NONE',  ( -0.000000000000000000, -1.000000000000000000, 2.537652627714643577E-15 ) ) ;
#31801=CARTESIAN_POINT ( 'NONE',  ( 0.000000000000000000, 0.000000000000000000, 0.000000000000000000 ) ) ;
#31812=VERTEX_POINT ( 'NONE', #18320 ) ;
#31816=EDGE_LOOP ( 'NONE', ( #6944, #34295, #3119, #39048 ) ) ;
#31819=CARTESIAN_POINT ( 'NONE',  ( 164.9999999999999716, -174.9999999999999716, -344.0000000000001137 ) ) ;
#31822=EDGE_CURVE ( 'NONE', #49726, #20342, #37369, .T. ) ;
#31844=LINE ( 'NONE', #43359, #40696 ) ;
#31851=EDGE_LOOP ( 'NONE', ( #2717, #22793, #43861, #19990 ) ) ;
#31857=EDGE_CURVE ( 'NONE', #4748, #15011, #47362, .T. ) ;
#31861=EDGE_CURVE ( 'NONE', #7906, #18739, #40848, .T. ) ;
#31863=AXIS2_PLACEMENT_3D ( 'NONE', #2615, #21622, #10077 ) ;
#31868=CARTESIAN_POINT ( 'NONE',  ( 168.9999999999999716, -7.999999999999952038, -340.0000000000001137 ) ) ;
#31869=EDGE_CURVE ( 'NONE', #41575, #2449, #21422, .T. ) ;
#31870=PLANE ( 'NONE',  #42518 ) ;
#31872=CLOSED_SHELL ( 'NONE', ( #13829, #35360, #10809, #2990, #18281, #15983, #20971, #43386, #46780, #40301, #48121, #22702, #38447, #49897, #27295, #31260, #8895, #10185 ) ) ;
#31877=DIRECTION ( 'NONE',  ( 1.132880637372608740E-16, 4.718402560806925739E-50, 1.000000000000000000 ) ) ;
#31879=FACE_OUTER_BOUND ( 'NONE', #36043, .T. ) ;
#31881=DIRECTION ( 'NONE',  ( 0.000000000000000000, 6.123233995736766036E-17, -1.000000000000000000 ) ) ;
#31883=EDGE_LOOP ( 'NONE', ( #49513, #37091, #27729, #46122 ) ) ;
#31887=VERTEX_POINT ( 'NONE', #34510 ) ;
#31890=CARTESIAN_POINT ( 'NONE',  ( 5.551115123125782702E-14, -184.9999999999999716, 355.9999999999997726 ) ) ;
#31894=EDGE_LOOP ( 'NONE', ( #8019, #42586, #42268, #37800, #41207, #45098, #39684, #363 ) ) ;
#31897=ORIENTED_EDGE ( 'NONE', *, *, #31142, .F. ) ;
#31898=DIRECTION ( 'NONE',  ( 0.000000000000000000, 0.000000000000000000, 1.000000000000000000 ) ) ;
#31902=DIRECTION ( 'NONE',  ( 1.000000000000000000, 0.000000000000000000, 0.000000000000000000 ) ) ;
#31907=CIRCLE ( 'NONE', #23690, 4.000000000000003553 ) ;
#31910=LINE ( 'NONE', #44181, #45967 ) ;
#31911=ORIENTED_EDGE ( 'NONE', *, *, #41692, .T. ) ;
#31912=ORIENTED_EDGE ( 'NONE', *, *, #2457, .F. ) ;
#31914=LINE ( 'NONE', #7543, #12385 ) ;
#31921=PLANE ( 'NONE',  #6156 ) ;
#31923=CARTESIAN_POINT ( 'NONE',  ( 0.000000000000000000, 0.000000000000000000, 0.000000000000000000 ) ) ;
#31929=CARTESIAN_POINT ( 'NONE',  ( 356.0000000000006253, 167.0000000000000000, 341.9999999999998295 ) ) ;
#31930=FACE_OUTER_BOUND ( 'NONE', #42363, .T. ) ;
#31931=ORIENTED_EDGE ( 'NONE', *, *, #39555, .T. ) ;
#31943=LINE ( 'NONE', #27058, #23755 ) ;
#31948=CYLINDRICAL_SURFACE ( 'NONE', #7421, 2.000000000000001776 ) ;
#31956=ORIENTED_EDGE ( 'NONE', *, *, #50609, .T. ) ;
#31959=CARTESIAN_POINT ( 'NONE',  ( -5.000000000000000000, 184.8000000000000114, -359.8000000000002387 ) ) ;
#31960=CYLINDRICAL_SURFACE ( 'NONE', #49312, 4.000000000000003553 ) ;
#31962=ORIENTED_EDGE ( 'NONE', *, *, #17243, .F. ) ;
#31964=EDGE_CURVE ( 'NONE', #19831, #38131, #15002, .T. ) ;
#31976=ORIENTED_EDGE ( 'NONE', *, *, #9089, .F. ) ;
#31977=ORIENTED_EDGE ( 'NONE', *, *, #2946, .T. ) ;
#31985=ADVANCED_FACE ( 'NONE', ( #35038 ), #49830, .F. ) ;
#31986=EDGE_CURVE ( 'NONE', #24656, #29740, #11156, .T. ) ;
#31988=ORIENTED_EDGE ( 'NONE', *, *, #514, .T. ) ;
#32001=ORIENTED_EDGE ( 'NONE', *, *, #43679, .T. ) ;
#32007=AXIS2_PLACEMENT_3D ( 'NONE', #32033, #47624, #28178 ) ;
#32010=ORIENTED_EDGE ( 'NONE', *, *, #17428, .T. ) ;
#32021=ORIENTED_EDGE ( 'NONE', *, *, #5123, .T. ) ;
#32024=CARTESIAN_POINT ( 'NONE',  ( 344.0000000000000000, -165.0000000000001137, -94.00000000000019895 ) ) ;
#32029=DIRECTION ( 'NONE',  ( 0.000000000000000000, 0.000000000000000000, -1.000000000000000000 ) ) ;
#32033=CARTESIAN_POINT ( 'NONE',  ( 168.9999999999999716, -272.5000000000000000, -110.9999999999999005 ) ) ;
#32035=DIRECTION ( 'NONE',  ( -0.000000000000000000, 1.000000000000000000, 0.000000000000000000 ) ) ;
#32036=ORIENTED_EDGE ( 'NONE', *, *, #23253, .F. ) ;
#32037=VECTOR ( 'NONE', #9904, 1000.000000000000000 ) ;
#32044=DIRECTION ( 'NONE',  ( 1.000000000000000000, 0.000000000000000000, 0.000000000000000000 ) ) ;
#32045=CARTESIAN_POINT ( 'NONE',  ( 166.9999999999999716, -184.9999999999999716, -356.0000000000014211 ) ) ;
#32052=CYLINDRICAL_SURFACE ( 'NONE', #18268, 4.000000000000003553 ) ;
#32059=ORIENTED_EDGE ( 'NONE', *, *, #35406, .T. ) ;
#32061=VERTEX_POINT ( 'NONE', #36036 ) ;
#32069=VECTOR ( 'NONE', #42148, 1000.000000000000000 ) ;
#32074=FACE_BOUND ( 'NONE', #9762, .T. ) ;
#32081=CARTESIAN_POINT ( 'NONE',  ( 356.0000000000000000, -169.0000000000001137, -349.9999999999999432 ) ) ;
#32083=CARTESIAN_POINT ( 'NONE',  ( 181.0000000000000568, 175.0000000000000284, 355.9999999999998863 ) ) ;
#32087=FACE_OUTER_BOUND ( 'NONE', #22088, .T. ) ;
#32092=DIRECTION ( 'NONE',  ( -1.110223024625156171E-16, 0.7071067811865474617, -0.7071067811865474617 ) ) ;
#32095=DIRECTION ( 'NONE',  ( 0.000000000000000000, 2.265761274745217480E-16, -1.000000000000000000 ) ) ;
#32096=CIRCLE ( 'NONE', #1766, 2.000000000000001776 ) ;
#32101=DIRECTION ( 'NONE',  ( 1.000000000000000000, -3.172065745548403743E-16, 1.587271980518778491E-16 ) ) ;
#32105=DIRECTION ( 'NONE',  ( -4.758098676964957447E-16, -1.000000000000000000, 7.143884938411937192E-48 ) ) ;
#32106=DIRECTION ( 'NONE',  ( 1.000000000000000000, 0.000000000000000000, 0.000000000000000000 ) ) ;
#32107=ORIENTED_EDGE ( 'NONE', *, *, #47123, .F. ) ;
#32109=EDGE_CURVE ( 'NONE', #46256, #16880, #7262, .T. ) ;
#32110=CARTESIAN_POINT ( 'NONE',  ( 340.0000000000000568, 177.9999999999999432, -3.000000000000003109 ) ) ;
#32123=PLANE ( 'NONE',  #17339 ) ;
#32124=VERTEX_POINT ( 'NONE', #35801 ) ;
#32125=DIRECTION ( 'NONE',  ( 1.000000000000000000, 0.000000000000000000, 0.000000000000000000 ) ) ;
#32128=CARTESIAN_POINT ( 'NONE',  ( 181.0000000000000000, -272.4999999999999432, -359.9999999999999432 ) ) ;
#32129=DIRECTION ( 'NONE',  ( -1.000000000000000000, 4.105366553918459587E-48, 1.586032880504786307E-16 ) ) ;
#32131=DIRECTION ( 'NONE',  ( 1.000000000000000000, 0.000000000000000000, 0.000000000000000000 ) ) ;
#32132=AXIS2_PLACEMENT_3D ( 'NONE', #31537, #35143, #727 ) ;
#32138=CIRCLE ( 'NONE', #1127, 4.000000000000003553 ) ;
#32142=VECTOR ( 'NONE', #43979, 1000.000000000000000 ) ;
#32143=FACE_OUTER_BOUND ( 'NONE', #13200, .T. ) ;
#32149=EDGE_CURVE ( 'NONE', #29100, #14588, #36296, .T. ) ;
#32155=CARTESIAN_POINT ( 'NONE',  ( 169.0000000000000000, -174.9999999999999716, -115.0000000000001563 ) ) ;
#32156=CARTESIAN_POINT ( 'NONE',  ( 0.000000000000000000, 175.0000000000000284, 353.7500000000001705 ) ) ;
#32158=AXIS2_PLACEMENT_3D ( 'NONE', #20647, #8604, #28853 ) ;
#32163=CARTESIAN_POINT ( 'NONE',  ( 342.0000000000000000, 165.0000000000000000, -94.00000000000019895 ) ) ;
#32173=LINE ( 'NONE', #9071, #15142 ) ;
#32179=DIRECTION ( 'NONE',  ( 1.333906992743555050E-23, -1.000000000000000000, 0.000000000000000000 ) ) ;
#32182=VECTOR ( 'NONE', #9320, 1000.000000000000000 ) ;
#32183=CARTESIAN_POINT ( 'NONE',  ( 356.0000000000000000, 165.0000000000001705, -340.0000000000002842 ) ) ;
#32190=DIRECTION ( 'NONE',  ( 1.860490536778032451E-50, 0.000000000000000000, -1.000000000000000000 ) ) ;
#32193=CARTESIAN_POINT ( 'NONE',  ( 356.0000000000006253, 167.0000000000000000, -342.0000000000001137 ) ) ;
#32195=AXIS2_PLACEMENT_3D ( 'NONE', #25191, #9290, #2339 ) ;
#32197=VERTEX_POINT ( 'NONE', #41629 ) ;
#32201=EDGE_CURVE ( 'NONE', #30616, #10238, #21988, .T. ) ;
#32204=CARTESIAN_POINT ( 'NONE',  ( 181.0000000000000284, -168.9999999999999432, -115.0000000000001847 ) ) ;
#32212=ORIENTED_EDGE ( 'NONE', *, *, #10456, .F. ) ;
#32214=STYLED_ITEM('',(#50747),#39303);
#32223=EDGE_CURVE ( 'NONE', #22898, #18727, #9711, .T. ) ;
#32234=CARTESIAN_POINT ( 'NONE',  ( 181.0000000000000568, -164.9999999999999432, 341.9999999999998863 ) ) ;
#32246=( GEOMETRIC_REPRESENTATION_CONTEXT ( 3 ) GLOBAL_UNCERTAINTY_ASSIGNED_CONTEXT ( ( #11619 ) ) GLOBAL_UNIT_ASSIGNED_CONTEXT ( ( #8724, #35925, #20752 ) ) REPRESENTATION_CONTEXT ( 'NONE', 'WORKASPACE' ) );
#32249=VECTOR ( 'NONE', #11280, 1000.000000000000000 ) ;
#32258=ORIENTED_EDGE ( 'NONE', *, *, #9110, .T. ) ;
#32259=VERTEX_POINT ( 'NONE', #36799 ) ;
#32262=ADVANCED_FACE ( 'NONE', ( #13906 ), #21366, .T. ) ;
#32267=LINE ( 'NONE', #40467, #33126 ) ;
#32292=VECTOR ( 'NONE', #40263, 1000.000000000000000 ) ;
#32294=AXIS2_PLACEMENT_3D ( 'NONE', #33875, #26158, #2799 ) ;
#32302=DIRECTION ( 'NONE',  ( -1.000000000000000000, 0.000000000000000000, 0.000000000000000000 ) ) ;
#32303=UNCERTAINTY_MEASURE_WITH_UNIT (LENGTH_MEASURE( 1.000000000000000082E-05 ), #49817, 'distance_accuracy_value', 'NONE');
#32308=EDGE_CURVE ( 'NONE', #48932, #11192, #7755, .T. ) ;
#32313=ORIENTED_EDGE ( 'NONE', *, *, #43679, .F. ) ;
#32317=ORIENTED_EDGE ( 'NONE', *, *, #13519, .F. ) ;
#32322=DIRECTION ( 'NONE',  ( -0.000000000000000000, -0.000000000000000000, 1.000000000000000000 ) ) ;
#32326=( BOUNDED_CURVE ( )  B_SPLINE_CURVE ( 3, ( #2038, #9724, #33598, #40785 ),
 .UNSPECIFIED., .F., .F. ) 
 B_SPLINE_CURVE_WITH_KNOTS ( ( 4, 4 ),
 ( 3.141592653589793560, 4.712388980384689674 ),
 .UNSPECIFIED. ) 
 CURVE ( )  GEOMETRIC_REPRESENTATION_ITEM ( )  RATIONAL_B_SPLINE_CURVE ( ( 1.000000000000000000, 0.8047378541243650485, 0.8047378541243650485, 1.000000000000000000 ) ) 
 REPRESENTATION_ITEM ( '' )  );
#32327=EDGE_LOOP ( 'NONE', ( #8662, #6502, #29411, #6759 ) ) ;
#32328=DIRECTION ( 'NONE',  ( 0.000000000000000000, -1.000000000000000000, 0.000000000000000000 ) ) ;
#32336=FACE_OUTER_BOUND ( 'NONE', #46907, .T. ) ;
#32341=AXIS2_PLACEMENT_3D ( 'NONE', #6028, #21681, #21423 ) ;
#32349=CARTESIAN_POINT ( 'NONE',  ( 340.0000000000000568, 185.0000000000000284, 349.9999999999997726 ) ) ;
#32355=CIRCLE ( 'NONE', #41351, 2.000000000000001776 ) ;
#32356=ORIENTED_EDGE ( 'NONE', *, *, #3795, .T. ) ;
#32358=DIRECTION ( 'NONE',  ( 1.587271980518778491E-16, -5.169878828456422968E-26, -1.000000000000000000 ) ) ;
#32359=LINE ( 'NONE', #35964, #11125 ) ;
#32377=LINE ( 'NONE', #17893, #49229 ) ;
#32389=AXIS2_PLACEMENT_3D ( 'NONE', #33488, #45740, #33246 ) ;
#32395=CYLINDRICAL_SURFACE ( 'NONE', #37683, 2.000000000000001776 ) ;
#32396=EDGE_CURVE ( 'NONE', #31718, #8840, #27251, .T. ) ;
#32401=PLANE ( 'NONE',  #35630 ) ;
#32404=AXIS2_PLACEMENT_3D ( 'NONE', #48482, #13862, #40586 ) ;
#32405=ORIENTED_EDGE ( 'NONE', *, *, #33096, .T. ) ;
#32407=ORIENTED_EDGE ( 'NONE', *, *, #17612, .T. ) ;
#32412=CARTESIAN_POINT ( 'NONE',  ( 169.0000000000000000, -174.9999999999999716, -99.00000000000014211 ) ) ;
#32416=EDGE_LOOP ( 'NONE', ( #3821, #32600, #26418, #44041 ) ) ;
#32419=EDGE_CURVE ( 'NONE', #34763, #34025, #14678, .T. ) ;
#32425=CIRCLE ( 'NONE', #26664, 4.000000000000003553 ) ;
#32426=DIRECTION ( 'NONE',  ( -1.000000000000000000, -0.000000000000000000, -0.000000000000000000 ) ) ;
#32436=ADVANCED_FACE ( 'NONE', ( #23648 ), #31870, .T. ) ;
#32439=EDGE_LOOP ( 'NONE', ( #11322, #16356, #21541, #1731, #6124, #30105, #17230, #18866 ) ) ;
#32444=DIRECTION ( 'NONE',  ( 1.132880637372608740E-16, 4.718402560806925739E-50, 1.000000000000000000 ) ) ;
#32451=DIRECTION ( 'NONE',  ( 1.000000000000000000, 0.000000000000000000, -1.586032892321652482E-16 ) ) ;
#32457=DIRECTION ( 'NONE',  ( 0.000000000000000000, 1.000000000000000000, 7.004339610132985974E-48 ) ) ;
#32464=CARTESIAN_POINT ( 'NONE',  ( 0.000000000000000000, 185.0000000000000284, -356.0000000000002274 ) ) ;
#32466=DIRECTION ( 'NONE',  ( 3.172065745548403743E-16, 1.000000000000000000, 0.000000000000000000 ) ) ;
#32468=VECTOR ( 'NONE', #39294, 1000.000000000000000 ) ;
#32471=EDGE_CURVE ( 'NONE', #47169, #50656, #35469, .T. ) ;
#32481=( NAMED_UNIT ( * ) SI_UNIT ( $, .STERADIAN. ) SOLID_ANGLE_UNIT ( ) );
#32484=VERTEX_POINT ( 'NONE', #816 ) ;
#32485=EDGE_CURVE ( 'NONE', #13307, #25458, #16458, .T. ) ;
#32489=AXIS2_PLACEMENT_3D ( 'NONE', #18289, #1659, #32973 ) ;
#32497=ORIENTED_EDGE ( 'NONE', *, *, #25378, .T. ) ;
#32505=EDGE_CURVE ( 'NONE', #49828, #24745, #13581, .T. ) ;
#32507=EDGE_CURVE ( 'NONE', #14529, #19026, #36223, .T. ) ;
#32523=ORIENTED_EDGE ( 'NONE', *, *, #49942, .T. ) ;
#32532=CARTESIAN_POINT ( 'NONE',  ( 344.0000000000000000, -166.9999999999999716, 341.9999999999998295 ) ) ;
#32536=CARTESIAN_POINT ( 'NONE',  ( 341.9999999999999432, 181.0000000000000568, -356.0000000000002274 ) ) ;
#32542=ORIENTED_EDGE ( 'NONE', *, *, #376, .F. ) ;
#32545=LINE ( 'NONE', #32791, #41418 ) ;
#32547=AXIS2_PLACEMENT_3D ( 'NONE', #44587, #28479, #40035 ) ;
#32557=EDGE_CURVE ( 'NONE', #31711, #49297, #19558, .T. ) ;
#32558=EDGE_CURVE ( 'NONE', #31642, #15166, #37738, .T. ) ;
#32572=PLANE ( 'NONE',  #34415 ) ;
#32573=( BOUNDED_CURVE ( )  B_SPLINE_CURVE ( 3, ( #15965, #8782, #24430, #25173 ),
 .UNSPECIFIED., .F., .F. ) 
 B_SPLINE_CURVE_WITH_KNOTS ( ( 4, 4 ),
 ( 3.141592653589793116, 4.712388980384689674 ),
 .UNSPECIFIED. ) 
 CURVE ( )  GEOMETRIC_REPRESENTATION_ITEM ( )  RATIONAL_B_SPLINE_CURVE ( ( 1.000000000000000000, 0.8047378541243649375, 0.8047378541243649375, 1.000000000000000000 ) ) 
 REPRESENTATION_ITEM ( '' )  );
#32582=ORIENTED_EDGE ( 'NONE', *, *, #17340, .T. ) ;
#32591=PLANE ( 'NONE',  #1044 ) ;
#32592=EDGE_LOOP ( 'NONE', ( #2219, #41088, #11049, #46942 ) ) ;
#32595=CARTESIAN_POINT ( 'NONE',  ( 169.0000000000000000, -174.9999999999999716, -113.0000000000001563 ) ) ;
#32598=CARTESIAN_POINT ( 'NONE',  ( 360.0000000000000000, -169.0000000000001137, -349.9999999999999432 ) ) ;
#32599=CARTESIAN_POINT ( 'NONE',  ( 166.9999999999999716, -5.999999999999950262, 339.9999999999998295 ) ) ;
#32600=ORIENTED_EDGE ( 'NONE', *, *, #23346, .F. ) ;
#32601=EDGE_CURVE ( 'NONE', #29839, #34606, #9503, .T. ) ;
#32611=DIRECTION ( 'NONE',  ( 0.000000000000000000, -1.000000000000000000, 2.969158215481698263E-48 ) ) ;
#32616=CARTESIAN_POINT ( 'NONE',  ( 359.9999999999999432, -181.0000000000001421, -349.9999999999998863 ) ) ;
#32624=VECTOR ( 'NONE', #31233, 1000.000000000000000 ) ;
#32626=DIRECTION ( 'NONE',  ( 1.586032892321652236E-16, 1.000000000000000000, 2.288264760618012091E-48 ) ) ;
#32639=CARTESIAN_POINT ( 'NONE',  ( 342.0000000000000568, 181.0000000000000284, 355.9999999999998863 ) ) ;
#32645=CARTESIAN_POINT ( 'NONE',  ( 168.9999999999999716, -270.4999999999999432, -339.9999999999998863 ) ) ;
#32646=DIRECTION ( 'NONE',  ( 0.000000000000000000, -0.000000000000000000, 1.000000000000000000 ) ) ;
#32663=CARTESIAN_POINT ( 'NONE',  ( 341.9999999999999432, 167.8284271247463835, -342.8284271247465540 ) ) ;
#32664=ORIENTED_EDGE ( 'NONE', *, *, #3585, .T. ) ;
#32665=CARTESIAN_POINT ( 'NONE',  ( 5.551115123125782702E-14, -180.9999999999999716, 341.9999999999997726 ) ) ;
#32667=CARTESIAN_POINT ( 'NONE',  ( 183.0000000000000000, -268.5000000000002842, -114.9999999999999147 ) ) ;
#32672=CARTESIAN_POINT ( 'NONE',  ( 344.0000000000000000, -165.0000000000001137, 340.0000000000000568 ) ) ;
#32678=LINE ( 'NONE', #380, #14202 ) ;
#32679=VERTEX_POINT ( 'NONE', #23330 ) ;
#32680=DIRECTION ( 'NONE',  ( 0.000000000000000000, -5.664403186863042467E-17, -1.000000000000000000 ) ) ;
#32681=ORIENTED_EDGE ( 'NONE', *, *, #10709, .F. ) ;
#32683=DIRECTION ( 'NONE',  ( 1.000000000000000000, -3.172065799423185948E-16, 1.587271980518778491E-16 ) ) ;
#32684=DIRECTION ( 'NONE',  ( 3.172065745548403743E-16, 1.000000000000000000, 0.000000000000000000 ) ) ;
#32685=AXIS2_PLACEMENT_3D ( 'NONE', #36092, #16320, #35847 ) ;
#32690=FACE_BOUND ( 'NONE', #23188, .T. ) ;
#32691=VECTOR ( 'NONE', #40622, 1000.000000000000000 ) ;
#32696=VECTOR ( 'NONE', #8753, 1000.000000000000000 ) ;
#32702=ORIENTED_EDGE ( 'NONE', *, *, #33113, .T. ) ;
#32706=FACE_OUTER_BOUND ( 'NONE', #15337, .T. ) ;
#32710=ORIENTED_EDGE ( 'NONE', *, *, #18925, .F. ) ;
#32721=VERTEX_POINT ( 'NONE', #43583 ) ;
#32733=CARTESIAN_POINT ( 'NONE',  ( 169.0000000000000000, -174.9999999999999716, -115.0000000000001563 ) ) ;
#32735=CARTESIAN_POINT ( 'NONE',  ( 181.0000000000000000, -180.9999999999999716, -340.0000000000001137 ) ) ;
#32737=CARTESIAN_POINT ( 'NONE',  ( 355.9999999999999432, -185.0000000000002558, -360.0000000000003411 ) ) ;
#32739=CIRCLE ( 'NONE', #3227, 4.000000000000003553 ) ;
#32745=LINE ( 'NONE', #40947, #8156 ) ;
#32756=FACE_OUTER_BOUND ( 'NONE', #33385, .T. ) ;
#32760=CARTESIAN_POINT ( 'NONE',  ( 357.1715728752537871, 183.0000000000000853, 357.9999999999998295 ) ) ;
#32761=VECTOR ( 'NONE', #3837, 1000.000000000000000 ) ;
#32764=ORIENTED_EDGE ( 'NONE', *, *, #15993, .T. ) ;
#32766=DIRECTION ( 'NONE',  ( -0.000000000000000000, -0.000000000000000000, 1.000000000000000000 ) ) ;
#32784=ORIENTED_EDGE ( 'NONE', *, *, #44055, .F. ) ;
#32791=CARTESIAN_POINT ( 'NONE',  ( 355.9999999999999432, 174.9999999999996305, -360.0000000000003411 ) ) ;
#32792=ORIENTED_EDGE ( 'NONE', *, *, #41794, .T. ) ;
#32797=CARTESIAN_POINT ( 'NONE',  ( 343.9999999999999432, -183.0000000000001421, -349.9999999999998863 ) ) ;
#32809=AXIS2_PLACEMENT_3D ( 'NONE', #12715, #42998, #42733 ) ;
#32812=CIRCLE ( 'NONE', #7429, 2.000000000000001776 ) ;
#32814=VECTOR ( 'NONE', #39547, 1000.000000000000000 ) ;
#32817=PLANE ( 'NONE',  #44637 ) ;
#32818=DIRECTION ( 'NONE',  ( 1.000000000000000000, 0.000000000000000000, 0.000000000000000000 ) ) ;
#32826=LINE ( 'NONE', #1271, #31404 ) ;
#32829=ORIENTED_EDGE ( 'NONE', *, *, #32109, .F. ) ;
#32832=VERTEX_POINT ( 'NONE', #31305 ) ;
#32834=CYLINDRICAL_SURFACE ( 'NONE', #44202, 3.749999999999975575 ) ;
#32837=EDGE_CURVE ( 'NONE', #17816, #43954, #47395, .T. ) ;
#32841=LINE ( 'NONE', #33093, #31361 ) ;
#32842=DIRECTION ( 'NONE',  ( 2.958228394578793832E-31, 0.000000000000000000, 1.000000000000000000 ) ) ;
#32843=ORIENTED_EDGE ( 'NONE', *, *, #31509, .F. ) ;
#32863=ADVANCED_FACE ( 'NONE', ( #48399 ), #20741, .T. ) ;
#32868=EDGE_CURVE ( 'NONE', #38709, #40720, #44559, .T. ) ;
#32873=DIRECTION ( 'NONE',  ( -1.000000000000000000, 5.326388832052271710E-25, -1.587271980518778491E-16 ) ) ;
#32876=LINE ( 'NONE', #17211, #31439 ) ;
#32882=VECTOR ( 'NONE', #8596, 1000.000000000000000 ) ;
#32887=ORIENTED_EDGE ( 'NONE', *, *, #23419, .F. ) ;
#32893=EDGE_LOOP ( 'NONE', ( #25901, #17691, #2328, #15498 ) ) ;
#32905=CARTESIAN_POINT ( 'NONE',  ( 356.0000000000000568, 185.0000000000001137, 359.9999999999998295 ) ) ;
#32909=CARTESIAN_POINT ( 'NONE',  ( 181.0000000000000000, -7.999999999999952038, -340.0000000000001137 ) ) ;
#32915=DIRECTION ( 'NONE',  ( 0.000000000000000000, 1.000000000000000000, 7.004339610132985974E-48 ) ) ;
#32916=ORIENTED_EDGE ( 'NONE', *, *, #5750, .T. ) ;
#32917=CARTESIAN_POINT ( 'NONE',  ( 339.9999999999999432, -169.0000000000001137, -344.0000000000002842 ) ) ;
#32928=EDGE_CURVE ( 'NONE', #41902, #46801, #1260, .T. ) ;
#32932=VECTOR ( 'NONE', #13682, 1000.000000000000000 ) ;
#32933=ORIENTED_EDGE ( 'NONE', *, *, #36517, .F. ) ;
#32935=VERTEX_POINT ( 'NONE', #21244 ) ;
#32948=DIRECTION ( 'NONE',  ( -1.000000000000000000, 0.000000000000000000, 1.586032892321651989E-16 ) ) ;
#32958=EDGE_CURVE ( 'NONE', #16715, #34606, #17397, .T. ) ;
#32963=CARTESIAN_POINT ( 'NONE',  ( 360.0000000000000000, -169.0000000000000568, -344.0000000000002842 ) ) ;
#32973=DIRECTION ( 'NONE',  ( 0.000000000000000000, -1.000000000000000000, 3.469446951953611033E-15 ) ) ;
#32974=CARTESIAN_POINT ( 'NONE',  ( 169.0000000000000284, 175.0000000000000284, 359.9999999999998863 ) ) ;
#32975=ORIENTED_EDGE ( 'NONE', *, *, #14234, .T. ) ;
#32982=ORIENTED_EDGE ( 'NONE', *, *, #26302, .F. ) ;
#32987=ORIENTED_EDGE ( 'NONE', *, *, #40948, .T. ) ;
#32988=ORIENTED_EDGE ( 'NONE', *, *, #47491, .T. ) ;
#33008=AXIS2_PLACEMENT_3D ( 'NONE', #11120, #31395, #49805 ) ;
#33018=CARTESIAN_POINT ( 'NONE',  ( 350.0000000000000000, 181.0000000000000284, -358.0000000000002274 ) ) ;
#33023=ORIENTED_EDGE ( 'NONE', *, *, #36838, .F. ) ;
#33034=CARTESIAN_POINT ( 'NONE',  ( 168.9999999999999716, -252.5000000000000000, -114.9999999999999574 ) ) ;
#33037=ORIENTED_EDGE ( 'NONE', *, *, #9816, .T. ) ;
#33041=EDGE_LOOP ( 'NONE', ( #36314, #27809, #37934, #33023 ) ) ;
#33056=ADVANCED_FACE ( 'NONE', ( #34784 ), #15759, .F. ) ;
#33061=DIRECTION ( 'NONE',  ( 2.168404344971008627E-19, -0.7071067811865474617, -0.7071067811865475727 ) ) ;
#33065=EDGE_CURVE ( 'NONE', #34472, #1515, #43366, .T. ) ;
#33066=DIRECTION ( 'NONE',  ( 1.000000000000000000, 0.000000000000000000, 0.000000000000000000 ) ) ;
#33074=ADVANCED_FACE ( 'NONE', ( #30665 ), #38881, .T. ) ;
#33076=LINE ( 'NONE', #49670, #42870 ) ;
#33080=VERTEX_POINT ( 'NONE', #126 ) ;
#33081=DIRECTION ( 'NONE',  ( 0.000000000000000000, -1.000000000000000000, 0.000000000000000000 ) ) ;
#33084=FACE_OUTER_BOUND ( 'NONE', #6514, .T. ) ;
#33091=CARTESIAN_POINT ( 'NONE',  ( 342.0000000000000568, 177.9999999999999432, -3.000000000000002665 ) ) ;
#33092=VECTOR ( 'NONE', #5584, 1000.000000000000000 ) ;
#33093=CARTESIAN_POINT ( 'NONE',  ( 355.9999999999999432, -185.0000000000001421, -360.0000000000003411 ) ) ;
#33096=EDGE_CURVE ( 'NONE', #48718, #6330, #29456, .T. ) ;
#33098=AXIS2_PLACEMENT_3D ( 'NONE', #19226, #30541, #26429 ) ;
#33103=ADVANCED_FACE ( 'NONE', ( #43462 ), #36803, .F. ) ;
#33105=DIRECTION ( 'NONE',  ( 0.000000000000000000, 0.000000000000000000, -1.000000000000000000 ) ) ;
#33108=VERTEX_POINT ( 'NONE', #16530 ) ;
#33112=ORIENTED_EDGE ( 'NONE', *, *, #43776, .T. ) ;
#33113=EDGE_CURVE ( 'NONE', #13147, #38490, #25135, .T. ) ;
#33116=CARTESIAN_POINT ( 'NONE',  ( 355.9999999999999432, 174.9999999999996589, -358.0000000000003411 ) ) ;
#33117=AXIS2_PLACEMENT_3D ( 'NONE', #26031, #17567, #33738 ) ;
#33119=DIRECTION ( 'NONE',  ( -1.000000000000000000, 0.000000000000000000, 0.000000000000000000 ) ) ;
#33125=LINE ( 'NONE', #5141, #9469 ) ;
#33126=VECTOR ( 'NONE', #20441, 1000.000000000000000 ) ;
#33127=ADVANCED_FACE ( 'NONE', ( #36042 ), #28829, .F. ) ;
#33139=ORIENTED_EDGE ( 'NONE', *, *, #17045, .F. ) ;
#33140=CARTESIAN_POINT ( 'NONE',  ( 358.3431457505075741, -185.0000000000000000, 359.9999999999997726 ) ) ;
#33141=ADVANCED_FACE ( 'NONE', ( #47778 ), #28573, .T. ) ;
#33152=EDGE_CURVE ( 'NONE', #12938, #37443, #47535, .T. ) ;
#33158=LINE ( 'NONE', #28533, #20934 ) ;
#33162=LINE ( 'NONE', #17242, #30858 ) ;
#33164=ADVANCED_FACE ( 'NONE', ( #39895 ), #16777, .F. ) ;
#33168=CARTESIAN_POINT ( 'NONE',  ( 341.9999999999999432, -181.0000000000001421, 356.0000000000000568 ) ) ;
#33169=AXIS2_PLACEMENT_3D ( 'NONE', #5352, #9200, #48656 ) ;
#33172=AXIS2_PLACEMENT_3D ( 'NONE', #9297, #48996, #36775 ) ;
#33178=EDGE_LOOP ( 'NONE', ( #37189, #12643, #18059, #43236 ) ) ;
#33184=ORIENTED_EDGE ( 'NONE', *, *, #34048, .F. ) ;
#33186=ORIENTED_EDGE ( 'NONE', *, *, #23253, .T. ) ;
#33191=DIRECTION ( 'NONE',  ( 0.000000000000000000, 0.000000000000000000, 1.000000000000000000 ) ) ;
#33195=ORIENTED_EDGE ( 'NONE', *, *, #49981, .T. ) ;
#33197=DIRECTION ( 'NONE',  ( 3.172065745548403743E-16, 1.000000000000000000, 0.000000000000000000 ) ) ;
#33199=EDGE_CURVE ( 'NONE', #44740, #41339, #41725, .T. ) ;
#33200=FACE_BOUND ( 'NONE', #18783, .T. ) ;
#33202=ORIENTED_EDGE ( 'NONE', *, *, #47726, .F. ) ;
#33203=AXIS2_PLACEMENT_3D ( 'NONE', #18609, #21969, #30430 ) ;
#33216=CARTESIAN_POINT ( 'NONE',  ( 358.0000000000000000, 169.0000000000000000, -344.0000000000001137 ) ) ;
#33224=ORIENTED_EDGE ( 'NONE', *, *, #2361, .F. ) ;
#33227=DIRECTION ( 'NONE',  ( 0.000000000000000000, 5.664403186863042467E-17, 1.000000000000000000 ) ) ;
#33228=CARTESIAN_POINT ( 'NONE',  ( 167.0000000000000000, -174.9999999999999716, -111.0000000000001563 ) ) ;
#33230=AXIS2_PLACEMENT_3D ( 'NONE', #43518, #4532, #36103 ) ;
#33238=ORIENTED_EDGE ( 'NONE', *, *, #49753, .T. ) ;
#33239=DIRECTION ( 'NONE',  ( 0.000000000000000000, 1.000000000000000000, 0.000000000000000000 ) ) ;
#33241=CARTESIAN_POINT ( 'NONE',  ( 360.0000000000000000, -169.0000000000001137, -344.0000000000003411 ) ) ;
#33246=DIRECTION ( 'NONE',  ( 0.000000000000000000, 0.000000000000000000, 1.000000000000000000 ) ) ;
#33247=LINE ( 'NONE', #48824, #10834 ) ;
#33248=EDGE_LOOP ( 'NONE', ( #28738, #29582, #37133, #9594 ) ) ;
#33249=DIRECTION ( 'NONE',  ( 3.172065745548403743E-16, 1.000000000000000000, 0.000000000000000000 ) ) ;
#33252=DIRECTION ( 'NONE',  ( 1.000000000000000000, 0.000000000000000000, 0.000000000000000000 ) ) ;
#33253=LINE ( 'NONE', #36610, #29070 ) ;
#33260=CARTESIAN_POINT ( 'NONE',  ( 356.0000000000000568, 165.0000000000000000, -90.00000000000018474 ) ) ;
#33265=AXIS2_PLACEMENT_3D ( 'NONE', #1811, #17454, #36739 ) ;
#33273=ADVANCED_FACE ( 'NONE', ( #6733 ), #6244, .T. ) ;
#33275=LINE ( 'NONE', #37127, #21729 ) ;
#33276=ORIENTED_EDGE ( 'NONE', *, *, #18103, .T. ) ;
#33279=AXIS2_PLACEMENT_3D ( 'NONE', #15815, #19910, #15566 ) ;
#33280=DIRECTION ( 'NONE',  ( 0.000000000000000000, -1.000000000000000000, -3.186989995019654210E-49 ) ) ;
#33292=VERTEX_POINT ( 'NONE', #44705 ) ;
#33301=DIRECTION ( 'NONE',  ( 0.000000000000000000, 0.000000000000000000, -1.000000000000000000 ) ) ;
#33303=ADVANCED_FACE ( 'NONE', ( #9582 ), #48791, .T. ) ;
#33316=CARTESIAN_POINT ( 'NONE',  ( 350.0000000000000000, -174.9999999999999432, -350.0000000000001705 ) ) ;
#33318=LINE ( 'NONE', #25350, #41005 ) ;
#33322=AXIS2_PLACEMENT_3D ( 'NONE', #39170, #7096, #26844 ) ;
#33325=DIRECTION ( 'NONE',  ( -1.000000000000000000, 0.000000000000000000, -7.793956916774525800E-48 ) ) ;
#33327=DIRECTION ( 'NONE',  ( 1.333906992743555050E-23, -1.000000000000000000, 0.000000000000000000 ) ) ;
#33339=ADVANCED_FACE ( 'NONE', ( #18023 ), #44944, .T. ) ;
#33342=DIRECTION ( 'NONE',  ( 1.000000000000000000, 0.000000000000000000, 7.793956916774525800E-48 ) ) ;
#33350=ORIENTED_EDGE ( 'NONE', *, *, #3053, .F. ) ;
#33352=VERTEX_POINT ( 'NONE', #46454 ) ;
#33359=DIRECTION ( 'NONE',  ( 1.860490536778032451E-50, 0.000000000000000000, -1.000000000000000000 ) ) ;
#33366=EDGE_LOOP ( 'NONE', ( #9650, #91, #14600, #12667 ) ) ;
#33367=DIRECTION ( 'NONE',  ( -1.000000000000000000, 0.000000000000000000, 0.000000000000000000 ) ) ;
#33379=CARTESIAN_POINT ( 'NONE',  ( 181.0000000000000000, 165.0000000000000000, -358.0000000000001705 ) ) ;
#33383=EDGE_CURVE ( 'NONE', #48420, #21503, #10835, .T. ) ;
#33385=EDGE_LOOP ( 'NONE', ( #42532, #34220, #16819, #46054 ) ) ;
#33391=EDGE_LOOP ( 'NONE', ( #48099, #13556 ) ) ;
#33396=( BOUNDED_CURVE ( )  B_SPLINE_CURVE ( 3, ( #1428, #24774, #40423, #5512 ),
 .UNSPECIFIED., .F., .F. ) 
 B_SPLINE_CURVE_WITH_KNOTS ( ( 4, 4 ),
 ( 1.570796326794889897, 3.141592653589793560 ),
 .UNSPECIFIED. ) 
 CURVE ( )  GEOMETRIC_REPRESENTATION_ITEM ( )  RATIONAL_B_SPLINE_CURVE ( ( 1.000000000000000000, 0.8047378541243632721, 0.8047378541243632721, 1.000000000000000000 ) ) 
 REPRESENTATION_ITEM ( '' )  );
#33399=EDGE_CURVE ( 'NONE', #34606, #15667, #13870, .T. ) ;
#33403=CARTESIAN_POINT ( 'NONE',  ( 0.000000000000000000, 181.0000000000000284, -356.0000000000002274 ) ) ;
#33405=CARTESIAN_POINT ( 'NONE',  ( 340.0000000000000568, 181.0000000000000284, 341.9999999999997726 ) ) ;
#33406=LINE ( 'NONE', #48976, #34095 ) ;
#33411=ORIENTED_EDGE ( 'NONE', *, *, #25960, .F. ) ;
#33419=ORIENTED_EDGE ( 'NONE', *, *, #9816, .F. ) ;
#33421=FACE_OUTER_BOUND ( 'NONE', #50646, .T. ) ;
#33426=EDGE_CURVE ( 'NONE', #38075, #28407, #49649, .T. ) ;
#33428=ORIENTED_EDGE ( 'NONE', *, *, #13718, .T. ) ;
#33432=EDGE_CURVE ( 'NONE', #47246, #8581, #32745, .T. ) ;
#33434=ORIENTED_EDGE ( 'NONE', *, *, #35748, .T. ) ;
#33435=CARTESIAN_POINT ( 'NONE',  ( -5.000000000000000000, 175.0000000000000284, -353.7500000000001705 ) ) ;
#33439=DIRECTION ( 'NONE',  ( 1.000000000000000000, 0.000000000000000000, 0.000000000000000000 ) ) ;
#33444=ORIENTED_EDGE ( 'NONE', *, *, #4979, .T. ) ;
#33454=LINE ( 'NONE', #17534, #28278 ) ;
#33463=VERTEX_POINT ( 'NONE', #33507 ) ;
#33466=VECTOR ( 'NONE', #36791, 1000.000000000000000 ) ;
#33467=ORIENTED_EDGE ( 'NONE', *, *, #27182, .T. ) ;
#33472=DIRECTION ( 'NONE',  ( 0.000000000000000000, 0.000000000000000000, 1.000000000000000000 ) ) ;
#33476=DIRECTION ( 'NONE',  ( 0.000000000000000000, 0.000000000000000000, 1.000000000000000000 ) ) ;
#33477=DIRECTION ( 'NONE',  ( 1.654361225106055350E-24, 1.654361225106055350E-24, -1.000000000000000000 ) ) ;
#33480=ORIENTED_EDGE ( 'NONE', *, *, #48132, .T. ) ;
#33488=CARTESIAN_POINT ( 'NONE',  ( 349.9999999999999432, -168.9999999999999432, 355.9999999999997726 ) ) ;
#33491=EDGE_CURVE ( 'NONE', #11298, #1975, #5719, .T. ) ;
#33492=PLANE ( 'NONE',  #16849 ) ;
#33499=DIRECTION ( 'NONE',  ( -1.000000000000000000, 0.000000000000000000, 0.000000000000000000 ) ) ;
#33500=DIRECTION ( 'NONE',  ( -0.000000000000000000, -0.000000000000000000, 1.000000000000000000 ) ) ;
#33503=CYLINDRICAL_SURFACE ( 'NONE', #46323, 4.000000000000003553 ) ;
#33506=DIRECTION ( 'NONE',  ( 0.000000000000000000, -1.000000000000000000, 3.469446951953611033E-15 ) ) ;
#33507=CARTESIAN_POINT ( 'NONE',  ( 181.0000000000000000, -272.5000000000000000, -114.9999999999999147 ) ) ;
#33508=ORIENTED_EDGE ( 'NONE', *, *, #50350, .T. ) ;
#33517=CARTESIAN_POINT ( 'NONE',  ( 164.9999999999999716, -268.4999999999999432, -349.9999999999999432 ) ) ;
#33519=ORIENTED_EDGE ( 'NONE', *, *, #28938, .T. ) ;
#33521=CARTESIAN_POINT ( 'NONE',  ( 341.9999999999999432, 182.1715728752539007, -357.1715728752538439 ) ) ;
#33522=ORIENTED_EDGE ( 'NONE', *, *, #16404, .T. ) ;
#33531=ADVANCED_FACE ( 'NONE', ( #30405 ), #7307, .T. ) ;
#33534=EDGE_CURVE ( 'NONE', #10975, #12244, #40963, .T. ) ;
#33540=VECTOR ( 'NONE', #20293, 1000.000000000000000 ) ;
#33541=CIRCLE ( 'NONE', #14663, 4.000000000000003553 ) ;
#33551=VECTOR ( 'NONE', #8029, 1000.000000000000000 ) ;
#33567=ORIENTED_EDGE ( 'NONE', *, *, #24918, .T. ) ;
#33569=VECTOR ( 'NONE', #24484, 1000.000000000000000 ) ;
#33576=DIRECTION ( 'NONE',  ( 0.000000000000000000, 2.537652627714642000E-15, 1.000000000000000000 ) ) ;
#33579=ORIENTED_EDGE ( 'NONE', *, *, #48951, .F. ) ;
#33582=CARTESIAN_POINT ( 'NONE',  ( 350.0000000000000000, -168.9999999999999432, -344.0000000000001705 ) ) ;
#33584=ORIENTED_EDGE ( 'NONE', *, *, #36847, .T. ) ;
#33587=ORIENTED_EDGE ( 'NONE', *, *, #39388, .F. ) ;
#33591=CARTESIAN_POINT ( 'NONE',  ( 344.0000000000000000, 167.0000000000000000, -342.0000000000001137 ) ) ;
#33593=FACE_OUTER_BOUND ( 'NONE', #44354, .T. ) ;
#33597=CARTESIAN_POINT ( 'NONE',  ( 166.9999999999999716, 165.0000000000000000, -344.0000000000001137 ) ) ;
#33598=CARTESIAN_POINT ( 'NONE',  ( 339.9999999999999432, 166.6568542494923406, -341.6568542494925396 ) ) ;
#33600=ORIENTED_EDGE ( 'NONE', *, *, #43491, .F. ) ;
#33606=AXIS2_PLACEMENT_3D ( 'NONE', #37745, #17724, #14109 ) ;
#33610=VECTOR ( 'NONE', #32683, 1000.000000000000000 ) ;
#33614=FACE_OUTER_BOUND ( 'NONE', #16467, .T. ) ;
#33616=EDGE_CURVE ( 'NONE', #19710, #34629, #41950, .T. ) ;
#33617=AXIS2_PLACEMENT_3D ( 'NONE', #18368, #45796, #1978 ) ;
#33618=AXIS2_PLACEMENT_3D ( 'NONE', #47629, #31788, #5064 ) ;
#33626=DIRECTION ( 'NONE',  ( 0.000000000000000000, 0.000000000000000000, -1.000000000000000000 ) ) ;
#33637=ORIENTED_EDGE ( 'NONE', *, *, #41222, .T. ) ;
#33641=AXIS2_PLACEMENT_3D ( 'NONE', #47540, #39636, #4233 ) ;
#33643=ORIENTED_EDGE ( 'NONE', *, *, #11230, .F. ) ;
#33651=AXIS2_PLACEMENT_3D ( 'NONE', #35736, #6169, #45132 ) ;
#33654=EDGE_LOOP ( 'NONE', ( #7153, #5813, #5912, #17703 ) ) ;
#33656=CARTESIAN_POINT ( 'NONE',  ( 358.0000000000000000, -182.1715728752539007, -357.1715728752540713 ) ) ;
#33669=ORIENTED_EDGE ( 'NONE', *, *, #4979, .F. ) ;
#33670=ORIENTED_EDGE ( 'NONE', *, *, #42192, .F. ) ;
#33674=LINE ( 'NONE', #37040, #42937 ) ;
#33678=DIRECTION ( 'NONE',  ( -1.000000000000000000, 0.000000000000000000, 0.000000000000000000 ) ) ;
#33683=LINE ( 'NONE', #14670, #46599 ) ;
#33687=CARTESIAN_POINT ( 'NONE',  ( 181.0000000000000853, -164.9999999999999432, -340.0000000000001137 ) ) ;
#33690=FACE_OUTER_BOUND ( 'NONE', #33366, .T. ) ;
#33692=VECTOR ( 'NONE', #439, 1000.000000000000000 ) ;
#33697=VERTEX_POINT ( 'NONE', #38625 ) ;
#33703=ORIENTED_EDGE ( 'NONE', *, *, #15993, .F. ) ;
#33704=ADVANCED_FACE ( 'NONE', ( #22446 ), #38118, .T. ) ;
#33705=EDGE_CURVE ( 'NONE', #16909, #21703, #31943, .T. ) ;
#33708=ORIENTED_EDGE ( 'NONE', *, *, #27646, .T. ) ;
#33723=DIRECTION ( 'NONE',  ( -1.000000000000000000, 0.000000000000000000, -2.958228394578794270E-31 ) ) ;
#33726=ORIENTED_EDGE ( 'NONE', *, *, #15825, .F. ) ;
#33727=VECTOR ( 'NONE', #19825, 1000.000000000000000 ) ;
#33728=VECTOR ( 'NONE', #25616, 1000.000000000000000 ) ;
#33732=DIRECTION ( 'NONE',  ( 0.000000000000000000, 0.000000000000000000, -1.000000000000000000 ) ) ;
#33733=EDGE_CURVE ( 'NONE', #41468, #35739, #43713, .T. ) ;
#33738=DIRECTION ( 'NONE',  ( 1.000000000000000000, 0.000000000000000000, 0.000000000000000000 ) ) ;
#33740=EDGE_LOOP ( 'NONE', ( #22861, #42776, #22348, #29309, #5948, #50325, #38472, #46845 ) ) ;
#33752=VECTOR ( 'NONE', #45881, 1000.000000000000000 ) ;
#33768=CARTESIAN_POINT ( 'NONE',  ( 0.000000000000000000, -175.0000000000000284, -353.7500000000001705 ) ) ;
#33773=VERTEX_POINT ( 'NONE', #39391 ) ;
#33785=ADVANCED_FACE ( 'NONE', ( #39138 ), #28075, .T. ) ;
#33786=DIRECTION ( 'NONE',  ( -4.996003610813203446E-16, -1.000000000000000000, 0.000000000000000000 ) ) ;
#33788=CARTESIAN_POINT ( 'NONE',  ( 0.000000000000000000, -175.0000000000000284, 346.2500000000002274 ) ) ;
#33789=ORIENTED_EDGE ( 'NONE', *, *, #4829, .T. ) ;
#33792=VECTOR ( 'NONE', #11568, 1000.000000000000000 ) ;
#33793=CARTESIAN_POINT ( 'NONE',  ( 339.9999999999999432, -180.9999999999999716, -356.0000000000002274 ) ) ;
#33794=LINE ( 'NONE', #15306, #22175 ) ;
#33797=DIRECTION ( 'NONE',  ( -1.586032892321652236E-16, -1.000000000000000000, -2.288264760618012091E-48 ) ) ;
#33799=CARTESIAN_POINT ( 'NONE',  ( 357.9999999999999432, -181.0000000000000853, 355.9999999999999432 ) ) ;
#33803=CARTESIAN_POINT ( 'NONE',  ( 360.0000000000000000, -168.9999999999999432, 343.9999999999998295 ) ) ;
#33804=DIRECTION ( 'NONE',  ( 0.000000000000000000, 0.000000000000000000, -1.000000000000000000 ) ) ;
#33807=ORIENTED_EDGE ( 'NONE', *, *, #36590, .F. ) ;
#33808=DIRECTION ( 'NONE',  ( 1.000000000000000000, -7.930164457481157120E-16, 1.587271980518778491E-16 ) ) ;
#33809=AXIS2_PLACEMENT_3D ( 'NONE', #8973, #44844, #21024 ) ;
#33815=VECTOR ( 'NONE', #31282, 1000.000000000000000 ) ;
#33820=CARTESIAN_POINT ( 'NONE',  ( 358.0000000000001137, 169.0000000000000000, 343.9999999999998295 ) ) ;
#33825=EDGE_CURVE ( 'NONE', #24412, #15793, #40641, .T. ) ;
#33828=ORIENTED_EDGE ( 'NONE', *, *, #28252, .T. ) ;
#33834=EDGE_CURVE ( 'NONE', #13231, #10537, #4971, .T. ) ;
#33838=ORIENTED_EDGE ( 'NONE', *, *, #37795, .T. ) ;
#33840=CYLINDRICAL_SURFACE ( 'NONE', #1698, 2.000000000000001776 ) ;
#33843=CARTESIAN_POINT ( 'NONE',  ( 340.0000000000000568, 181.0000000000000284, 343.9999999999997726 ) ) ;
#33846=FACE_OUTER_BOUND ( 'NONE', #23908, .T. ) ;
#33847=ADVANCED_FACE ( 'NONE', ( #9828 ), #25484, .F. ) ;
#33848=DIRECTION ( 'NONE',  ( -0.000000000000000000, -1.000000000000000000, 2.537652627714643577E-15 ) ) ;
#33849=ORIENTED_EDGE ( 'NONE', *, *, #35606, .T. ) ;
#33853=EDGE_LOOP ( 'NONE', ( #21283, #15295, #39457, #42066 ) ) ;
#33855=CARTESIAN_POINT ( 'NONE',  ( 339.9999999999999432, -164.9999999999999432, -344.0000000000001705 ) ) ;
#33856=ORIENTED_EDGE ( 'NONE', *, *, #1225, .T. ) ;
#33863=AXIS2_PLACEMENT_3D ( 'NONE', #48153, #21756, #2251 ) ;
#33865=CARTESIAN_POINT ( 'NONE',  ( 166.9999999999999716, -272.4999999999999432, -355.9999999999999432 ) ) ;
#33868=VECTOR ( 'NONE', #2196, 1000.000000000000000 ) ;
#33875=CARTESIAN_POINT ( 'NONE',  ( 355.9999999999999432, -174.9999999999999432, 359.9999999999998295 ) ) ;
#33885=ORIENTED_EDGE ( 'NONE', *, *, #27489, .T. ) ;
#33891=AXIS2_PLACEMENT_3D ( 'NONE', #20296, #28258, #43889 ) ;
#33892=CARTESIAN_POINT ( 'NONE',  ( 168.9999999999999716, -81.49999999999997158, -340.0000000000001137 ) ) ;
#33898=ORIENTED_EDGE ( 'NONE', *, *, #43098, .F. ) ;
#33902=DIRECTION ( 'NONE',  ( -1.586032892321652236E-16, -1.000000000000000000, -6.853681917100419162E-49 ) ) ;
#33913=ORIENTED_EDGE ( 'NONE', *, *, #45883, .F. ) ;
#33917=DIRECTION ( 'NONE',  ( 0.000000000000000000, 0.000000000000000000, -1.000000000000000000 ) ) ;
#33924=AXIS2_PLACEMENT_3D ( 'NONE', #6005, #25261, #21157 ) ;
#33927=AXIS2_PLACEMENT_3D ( 'NONE', #203, #15840, #31502 ) ;
#33932=DIRECTION ( 'NONE',  ( 0.000000000000000000, -2.537652627714643577E-15, -1.000000000000000000 ) ) ;
#33935=CARTESIAN_POINT ( 'NONE',  ( 185.0000000000000000, -174.9999999999999716, -356.0000000000001705 ) ) ;
#33937=ORIENTED_EDGE ( 'NONE', *, *, #45529, .F. ) ;
#33938=DIRECTION ( 'NONE',  ( -1.000000000000000000, 0.000000000000000000, 0.000000000000000000 ) ) ;
#33941=CARTESIAN_POINT ( 'NONE',  ( 167.0000000000000000, -174.9999999999999716, -99.00000000000014211 ) ) ;
#33944=ORIENTED_EDGE ( 'NONE', *, *, #10521, .F. ) ;
#33978=AXIS2_PLACEMENT_3D ( 'NONE', #33935, #13902, #21883 ) ;
#33980=ORIENTED_EDGE ( 'NONE', *, *, #13144, .F. ) ;
#33985=CARTESIAN_POINT ( 'NONE',  ( 358.0000000000000000, -168.9999999999999432, 343.9999999999998295 ) ) ;
#33989=FACE_OUTER_BOUND ( 'NONE', #4184, .T. ) ;
#33994=DIRECTION ( 'NONE',  ( 0.000000000000000000, 6.123233995736766036E-17, -1.000000000000000000 ) ) ;
#34000=ORIENTED_EDGE ( 'NONE', *, *, #30391, .T. ) ;
#34005=CARTESIAN_POINT ( 'NONE',  ( 357.9999999999999432, -181.0000000000000853, 355.9999999999999432 ) ) ;
#34019=VECTOR ( 'NONE', #32948, 1000.000000000000000 ) ;
#34021=DIRECTION ( 'NONE',  ( -1.586032892321652236E-16, -1.194346094642792789E-32, -1.000000000000000000 ) ) ;
#34025=VERTEX_POINT ( 'NONE', #14946 ) ;
#34044=CYLINDRICAL_SURFACE ( 'NONE', #1390, 2.000000000000001776 ) ;
#34045=CYLINDRICAL_SURFACE ( 'NONE', #9961, 4.000000000000003553 ) ;
#34046=CARTESIAN_POINT ( 'NONE',  ( 350.0000000000000000, 181.0000000000000284, -340.0000000000001705 ) ) ;
#34048=EDGE_CURVE ( 'NONE', #14610, #34262, #26251, .T. ) ;
#34052=CARTESIAN_POINT ( 'NONE',  ( 358.0000000000000568, -182.1715728752539292, 357.1715728752538439 ) ) ;
#34056=EDGE_CURVE ( 'NONE', #26176, #35933, #11095, .T. ) ;
#34057=AXIS2_PLACEMENT_3D ( 'NONE', #30881, #15457, #46214 ) ;
#34062=CIRCLE ( 'NONE', #18470, 2.000000000000001776 ) ;
#34064=EDGE_CURVE ( 'NONE', #35344, #42209, #21324, .T. ) ;
#34068=AXIS2_PLACEMENT_3D ( 'NONE', #48517, #21615, #18254 ) ;
#34071=LINE ( 'NONE', #13276, #5839 ) ;
#34073=DIRECTION ( 'NONE',  ( 0.000000000000000000, 2.537652627714642000E-15, 1.000000000000000000 ) ) ;
#34079=VECTOR ( 'NONE', #19624, 1000.000000000000000 ) ;
#34083=LINE ( 'NONE', #45076, #10624 ) ;
#34086=DIRECTION ( 'NONE',  ( -1.122149248522496843E-16, 0.7071067811865476838, 0.7071067811865474617 ) ) ;
#34094=DIRECTION ( 'NONE',  ( 0.000000000000000000, 0.000000000000000000, 1.000000000000000000 ) ) ;
#34095=VECTOR ( 'NONE', #10534, 1000.000000000000000 ) ;
#34096=EDGE_LOOP ( 'NONE', ( #40638, #38660 ) ) ;
#34098=CARTESIAN_POINT ( 'NONE',  ( 343.9999999999997158, -165.0000000000001137, -90.00000000000018474 ) ) ;
#34111=VECTOR ( 'NONE', #18561, 1000.000000000000000 ) ;
#34113=ORIENTED_EDGE ( 'NONE', *, *, #45832, .F. ) ;
#34114=DIRECTION ( 'NONE',  ( -1.000000000000000000, 1.586032997072805650E-16, 4.759647537211363479E-16 ) ) ;
#34115=FACE_OUTER_BOUND ( 'NONE', #14988, .T. ) ;
#34117=AXIS2_PLACEMENT_3D ( 'NONE', #36509, #12878, #1345 ) ;
#34121=CARTESIAN_POINT ( 'NONE',  ( 181.0000000000000000, -184.9999999999999716, -115.0000000000001279 ) ) ;
#34122=ADVANCED_FACE ( 'NONE', ( #31879 ), #34721, .F. ) ;
#34137=CIRCLE ( 'NONE', #32489, 4.000000000000003553 ) ;
#34142=VERTEX_POINT ( 'NONE', #43160 ) ;
#34144=CARTESIAN_POINT ( 'NONE',  ( 168.9999999999999716, 10.00000000000006395, -350.0000000000001705 ) ) ;
#34145=DIRECTION ( 'NONE',  ( 0.000000000000000000, 1.000000000000000000, 0.000000000000000000 ) ) ;
#34160=ORIENTED_EDGE ( 'NONE', *, *, #41343, .T. ) ;
#34161=( LENGTH_UNIT ( ) NAMED_UNIT ( * ) SI_UNIT ( .MILLI., .METRE. ) );
#34163=CYLINDRICAL_SURFACE ( 'NONE', #23692, 2.000000000000001776 ) ;
#34165=LINE ( 'NONE', #14636, #27034 ) ;
#34166=DIRECTION ( 'NONE',  ( -1.612977847700450206E-50, 0.000000000000000000, -1.000000000000000000 ) ) ;
#34170=ORIENTED_EDGE ( 'NONE', *, *, #50642, .T. ) ;
#34172=ADVANCED_FACE ( 'NONE', ( #43644 ), #46710, .T. ) ;
#34182=LINE ( 'NONE', #46933, #28741 ) ;
#34197=CARTESIAN_POINT ( 'NONE',  ( 0.000000000000000000, -166.9999999999999432, -344.0000000000001705 ) ) ;
#34198=CARTESIAN_POINT ( 'NONE',  ( 358.3431457505076310, -165.0000000000001137, 339.9999999999998863 ) ) ;
#34199=DIRECTION ( 'NONE',  ( -2.220446049250312588E-16, -0.7071067811865475727, -0.7071067811865474617 ) ) ;
#34201=EDGE_CURVE ( 'NONE', #7115, #43423, #12603, .T. ) ;
#34206=EDGE_LOOP ( 'NONE', ( #13007, #13707, #1583, #17427, #19065, #15028, #15379, #12257 ) ) ;
#34218=FACE_OUTER_BOUND ( 'NONE', #11726, .T. ) ;
#34219=ORIENTED_EDGE ( 'NONE', *, *, #4477, .F. ) ;
#34220=ORIENTED_EDGE ( 'NONE', *, *, #49342, .F. ) ;
#34221=CARTESIAN_POINT ( 'NONE',  ( 181.0000000000000000, -9.999999999999953815, -350.0000000000001705 ) ) ;
#34224=ORIENTED_EDGE ( 'NONE', *, *, #16854, .T. ) ;
#34230=PLANE ( 'NONE',  #49686 ) ;
#34237=ORIENTED_EDGE ( 'NONE', *, *, #24464, .T. ) ;
#34238=CARTESIAN_POINT ( 'NONE',  ( 341.6568542494924259, 185.0000000000000284, 359.9999999999998295 ) ) ;
#34239=DIRECTION ( 'NONE',  ( -1.586032892321652236E-16, -1.000000000000000000, -6.853681917100419162E-49 ) ) ;
#34251=EDGE_CURVE ( 'NONE', #17870, #47520, #22170, .T. ) ;
#34253=AXIS2_PLACEMENT_3D ( 'NONE', #21935, #2674, #3168 ) ;
#34257=DIRECTION ( 'NONE',  ( 1.000000000000000000, 0.000000000000000000, 0.000000000000000000 ) ) ;
#34258=CARTESIAN_POINT ( 'NONE',  ( 339.9999999999999432, 181.0000000000000568, -356.0000000000002274 ) ) ;
#34262=VERTEX_POINT ( 'NONE', #44148 ) ;
#34266=CARTESIAN_POINT ( 'NONE',  ( 165.0000000000000000, -174.9999999999999716, -99.00000000000014211 ) ) ;
#34276=ORIENTED_EDGE ( 'NONE', *, *, #34251, .F. ) ;
#34278=DIRECTION ( 'NONE',  ( 0.000000000000000000, 0.000000000000000000, -1.000000000000000000 ) ) ;
#34282=ORIENTED_EDGE ( 'NONE', *, *, #48841, .T. ) ;
#34283=DIRECTION ( 'NONE',  ( 1.132880637372608740E-16, 4.718402560806925739E-50, 1.000000000000000000 ) ) ;
#34286=ORIENTED_EDGE ( 'NONE', *, *, #27801, .T. ) ;
#34287=FACE_OUTER_BOUND ( 'NONE', #50217, .T. ) ;
#34295=ORIENTED_EDGE ( 'NONE', *, *, #176, .T. ) ;
#34304=DIRECTION ( 'NONE',  ( -1.000000000000000000, 0.000000000000000000, -2.958228394578794270E-31 ) ) ;
#34309=CLOSED_SHELL ( 'NONE', ( #43204, #44086, #17489, #15473, #40081, #12807, #29556, #44704, #888, #7372, #25044, #45928, #45876, #36274, #212, #16926, #27861, #47758 ) ) ;
#34324=DIRECTION ( 'NONE',  ( -1.000000000000000000, 0.000000000000000000, -2.958228394578794270E-31 ) ) ;
#34331=ORIENTED_EDGE ( 'NONE', *, *, #49690, .F. ) ;
#34342=CIRCLE ( 'NONE', #29428, 2.000000000000001776 ) ;
#34346=LINE ( 'NONE', #7143, #18555 ) ;
#34347=VECTOR ( 'NONE', #33367, 1000.000000000000000 ) ;
#34350=DIRECTION ( 'NONE',  ( 1.000000000000000000, 0.000000000000000000, 0.000000000000000000 ) ) ;
#34353=VECTOR ( 'NONE', #43482, 1000.000000000000000 ) ;
#34370=DIRECTION ( 'NONE',  ( -7.793956916774525800E-48, 0.000000000000000000, -1.000000000000000000 ) ) ;
#34371=LINE ( 'NONE', #38728, #35778 ) ;
#34374=AXIS2_PLACEMENT_3D ( 'NONE', #50291, #50545, #19289 ) ;
#34375=DIRECTION ( 'NONE',  ( 0.000000000000000000, 1.580451535867971417E-48, -1.000000000000000000 ) ) ;
#34406=DIRECTION ( 'NONE',  ( 1.000000000000000000, 0.000000000000000000, -1.586032892321652482E-16 ) ) ;
#34410=EDGE_CURVE ( 'NONE', #7540, #23937, #48964, .T. ) ;
#34412=DIRECTION ( 'NONE',  ( 0.000000000000000000, 1.000000000000000000, 0.000000000000000000 ) ) ;
#34415=AXIS2_PLACEMENT_3D ( 'NONE', #13292, #40761, #21253 ) ;
#34417=( BOUNDED_CURVE ( )  B_SPLINE_CURVE ( 3, ( #38982, #46112, #6909, #26662 ),
 .UNSPECIFIED., .F., .F. ) 
 B_SPLINE_CURVE_WITH_KNOTS ( ( 4, 4 ),
 ( 4.712388980384689674, 6.283185307179586232 ),
 .UNSPECIFIED. ) 
 CURVE ( )  GEOMETRIC_REPRESENTATION_ITEM ( )  RATIONAL_B_SPLINE_CURVE ( ( 1.000000000000000000, 0.8047378541243649375, 0.8047378541243649375, 1.000000000000000000 ) ) 
 REPRESENTATION_ITEM ( '' )  );
#34418=AXIS2_PLACEMENT_3D ( 'NONE', #20937, #1450, #28890 ) ;
#34420=CARTESIAN_POINT ( 'NONE',  ( 350.0000000000001137, 165.0000000000000000, 359.9999999999997726 ) ) ;
#34421=FACE_OUTER_BOUND ( 'NONE', #28051, .T. ) ;
#34432=VECTOR ( 'NONE', #28532, 1000.000000000000000 ) ;
#34434=ORIENTED_EDGE ( 'NONE', *, *, #43166, .F. ) ;
#34438=LINE ( 'NONE', #38036, #49320 ) ;
#34442=PLANE ( 'NONE',  #6383 ) ;
#34443=DIRECTION ( 'NONE',  ( 0.000000000000000000, 1.000000000000000000, 6.123233995736766036E-17 ) ) ;
#34444=CARTESIAN_POINT ( 'NONE',  ( -5.000000000000000000, -165.1999999999999602, 359.7999999999997840 ) ) ;
#34447=VERTEX_POINT ( 'NONE', #14377 ) ;
#34449=DIRECTION ( 'NONE',  ( 3.363195139050033768E-16, 0.7071067811865474617, 0.7071067811865475727 ) ) ;
#34450=CARTESIAN_POINT ( 'NONE',  ( 181.0000000000000000, -9.999999999999953815, -340.0000000000001137 ) ) ;
#34460=VECTOR ( 'NONE', #33359, 1000.000000000000000 ) ;
#34463=ORIENTED_EDGE ( 'NONE', *, *, #6058, .F. ) ;
#34469=LINE ( 'NONE', #11356, #35727 ) ;
#34471=EDGE_CURVE ( 'NONE', #21503, #29362, #16287, .T. ) ;
#34472=VERTEX_POINT ( 'NONE', #45892 ) ;
#34473=CARTESIAN_POINT ( 'NONE',  ( 344.0000000000000000, 175.0000000000000284, -108.0000000000002132 ) ) ;
#34477=ORIENTED_EDGE ( 'NONE', *, *, #49385, .F. ) ;
#34478=VERTEX_POINT ( 'NONE', #23338 ) ;
#34483=DIRECTION ( 'NONE',  ( -1.000000000000000000, 0.000000000000000000, 0.000000000000000000 ) ) ;
#34484=EDGE_CURVE ( 'NONE', #26083, #11650, #12056, .T. ) ;
#34492=EDGE_LOOP ( 'NONE', ( #2728, #29063, #30700, #4417 ) ) ;
#34493=VERTEX_POINT ( 'NONE', #39010 ) ;
#34497=VECTOR ( 'NONE', #17218, 1000.000000000000000 ) ;
#34498=VERTEX_POINT ( 'NONE', #11550 ) ;
#34502=DIRECTION ( 'NONE',  ( 0.000000000000000000, -2.537652627714643577E-15, -1.000000000000000000 ) ) ;
#34508=ADVANCED_FACE ( 'NONE', ( #43089 ), #30800, .T. ) ;
#34510=CARTESIAN_POINT ( 'NONE',  ( 344.0000000000000000, -164.9999999999999432, 339.9999999999998295 ) ) ;
#34512=ADVANCED_FACE ( 'NONE', ( #27199 ), #27701, .F. ) ;
#34519=FACE_OUTER_BOUND ( 'NONE', #17592, .T. ) ;
#34528=ORIENTED_EDGE ( 'NONE', *, *, #27717, .T. ) ;
#34532=VERTEX_POINT ( 'NONE', #35168 ) ;
#34533=DIRECTION ( 'NONE',  ( 0.000000000000000000, 0.000000000000000000, 1.000000000000000000 ) ) ;
#34538=EDGE_CURVE ( 'NONE', #32124, #25314, #15643, .T. ) ;
#34544=CARTESIAN_POINT ( 'NONE',  ( 350.0000000000000000, 183.0000000000000284, -356.0000000000002274 ) ) ;
#34548=ORIENTED_EDGE ( 'NONE', *, *, #47578, .T. ) ;
#34551=VECTOR ( 'NONE', #11376, 1000.000000000000000 ) ;
#34561=ORIENTED_EDGE ( 'NONE', *, *, #35958, .F. ) ;
#34562=DIRECTION ( 'NONE',  ( 6.203854594147707562E-25, -2.067951531382569187E-25, 1.000000000000000000 ) ) ;
#34564=CARTESIAN_POINT ( 'NONE',  ( 359.9999999999999432, 177.9999999999999716, -353.0000000000000568 ) ) ;
#34566=CARTESIAN_POINT ( 'NONE',  ( 359.9999999999999432, -181.0000000000001421, 356.0000000000000000 ) ) ;
#34567=EDGE_CURVE ( 'NONE', #26389, #43828, #46651, .T. ) ;
#34570=CARTESIAN_POINT ( 'NONE',  ( 341.9999999999999432, -169.0000000000001705, 344.0000000000000568 ) ) ;
#34573=( BOUNDED_CURVE ( )  B_SPLINE_CURVE ( 3, ( #38910, #27094, #47052, #44176 ),
 .UNSPECIFIED., .F., .F. ) 
 B_SPLINE_CURVE_WITH_KNOTS ( ( 4, 4 ),
 ( 2.784193070085688408E-13, 1.570796326794910991 ),
 .UNSPECIFIED. ) 
 CURVE ( )  GEOMETRIC_REPRESENTATION_ITEM ( )  RATIONAL_B_SPLINE_CURVE ( ( 1.000000000000000000, 0.8047378541244272210, 0.8047378541244272210, 1.000000000000000000 ) ) 
 REPRESENTATION_ITEM ( '' )  );
#34578=FACE_OUTER_BOUND ( 'NONE', #18000, .T. ) ;
#34591=DIRECTION ( 'NONE',  ( 1.333906992743555050E-23, -1.000000000000000000, 0.000000000000000000 ) ) ;
#34596=EDGE_LOOP ( 'NONE', ( #24550, #30001, #43273, #46241 ) ) ;
#34597=EDGE_CURVE ( 'NONE', #43608, #39344, #31193, .T. ) ;
#34606=VERTEX_POINT ( 'NONE', #23080 ) ;
#34612=DIRECTION ( 'NONE',  ( 0.000000000000000000, -1.000000000000000000, 0.000000000000000000 ) ) ;
#34613=ORIENTED_EDGE ( 'NONE', *, *, #1102, .F. ) ;
#34629=VERTEX_POINT ( 'NONE', #9199 ) ;
#34639=LINE ( 'NONE', #34144, #31261 ) ;
#34643=CARTESIAN_POINT ( 'NONE',  ( 0.000000000000000000, -168.9999999999999432, -358.0000000000002274 ) ) ;
#34647=ORIENTED_EDGE ( 'NONE', *, *, #37547, .F. ) ;
#34649=ORIENTED_EDGE ( 'NONE', *, *, #35914, .F. ) ;
#34650=CARTESIAN_POINT ( 'NONE',  ( 350.0000000000001137, 169.0000000000000000, 343.9999999999997726 ) ) ;
#34660=LINE ( 'NONE', #30809, #31436 ) ;
#34666=EDGE_CURVE ( 'NONE', #16118, #21503, #13044, .T. ) ;
#34667=VECTOR ( 'NONE', #2241, 1000.000000000000000 ) ;
#34670=ORIENTED_EDGE ( 'NONE', *, *, #41343, .F. ) ;
#34675=ORIENTED_EDGE ( 'NONE', *, *, #30361, .F. ) ;
#34678=CYLINDRICAL_SURFACE ( 'NONE', #10556, 2.000000000000001776 ) ;
#34683=ORIENTED_EDGE ( 'NONE', *, *, #39052, .T. ) ;
#34687=DIRECTION ( 'NONE',  ( 1.000000000000000000, 0.000000000000000000, 0.000000000000000000 ) ) ;
#34705=CARTESIAN_POINT ( 'NONE',  ( 181.0000000000000000, -164.9999999999999432, -358.0000000000001705 ) ) ;
#34707=ADVANCED_FACE ( 'NONE', ( #6359, #29973 ), #2512, .T. ) ;
#34710=ADVANCED_FACE ( 'NONE', ( #25868 ), #22265, .T. ) ;
#34712=DIRECTION ( 'NONE',  ( 1.333906992743555050E-23, -1.000000000000000000, 0.000000000000000000 ) ) ;
#34721=CYLINDRICAL_SURFACE ( 'NONE', #874, 2.000000000000001776 ) ;
#34722=CARTESIAN_POINT ( 'NONE',  ( 355.9999999999998863, -183.0000000000002274, -358.0000000000003411 ) ) ;
#34724=ORIENTED_EDGE ( 'NONE', *, *, #31296, .T. ) ;
#34730=ORIENTED_EDGE ( 'NONE', *, *, #48979, .F. ) ;
#34735=ORIENTED_EDGE ( 'NONE', *, *, #19553, .F. ) ;
#34736=ORIENTED_EDGE ( 'NONE', *, *, #17964, .T. ) ;
#34737=CARTESIAN_POINT ( 'NONE',  ( 167.0000000000000000, -174.9999999999999716, -99.00000000000014211 ) ) ;
#34738=CARTESIAN_POINT ( 'NONE',  ( 168.9999999999999716, -272.5000000000000000, -98.99999999999990052 ) ) ;
#34746=CARTESIAN_POINT ( 'NONE',  ( 344.0000000000000000, 175.0000000000000284, -110.0000000000002132 ) ) ;
#34749=EDGE_CURVE ( 'NONE', #34922, #25186, #45822, .T. ) ;
#34753=CARTESIAN_POINT ( 'NONE',  ( 168.9999999999999716, -180.9999999999999716, -350.0000000000001705 ) ) ;
#34761=ORIENTED_EDGE ( 'NONE', *, *, #8038, .F. ) ;
#34762=LINE ( 'NONE', #38353, #16821 ) ;
#34763=VERTEX_POINT ( 'NONE', #37190 ) ;
#34764=LINE ( 'NONE', #16011, #3729 ) ;
#34775=DIRECTION ( 'NONE',  ( 0.000000000000000000, 0.000000000000000000, 1.000000000000000000 ) ) ;
#34780=ADVANCED_FACE ( 'NONE', ( #20373 ), #11479, .F. ) ;
#34782=AXIS2_PLACEMENT_3D ( 'NONE', #775, #278, #27466 ) ;
#34784=FACE_OUTER_BOUND ( 'NONE', #15289, .T. ) ;
#34786=AXIS2_PLACEMENT_3D ( 'NONE', #43090, #4610, #31053 ) ;
#34795=ORIENTED_EDGE ( 'NONE', *, *, #11097, .F. ) ;
#34800=VERTEX_POINT ( 'NONE', #43967 ) ;
#34801=ORIENTED_EDGE ( 'NONE', *, *, #1438, .T. ) ;
#34802=DIRECTION ( 'NONE',  ( 0.000000000000000000, 1.000000000000000000, 7.004339610132985974E-48 ) ) ;
#34804=CARTESIAN_POINT ( 'NONE',  ( 340.0000000000000000, 175.0000000000000284, -94.00000000000019895 ) ) ;
#34808=ORIENTED_EDGE ( 'NONE', *, *, #17840, .F. ) ;
#34810=CARTESIAN_POINT ( 'NONE',  ( 340.0000000000000568, 169.0000000000000000, 339.9999999999997726 ) ) ;
#34812=VERTEX_POINT ( 'NONE', #26874 ) ;
#34816=AXIS2_PLACEMENT_3D ( 'NONE', #28793, #41274, #31898 ) ;
#34818=VERTEX_POINT ( 'NONE', #42269 ) ;
#34829=LINE ( 'NONE', #15048, #22855 ) ;
#34833=CARTESIAN_POINT ( 'NONE',  ( 181.0000000000000000, 6.000000000000060396, 339.9999999999998295 ) ) ;
#34847=CIRCLE ( 'NONE', #46254, 4.000000000000003553 ) ;
#34848=ORIENTED_EDGE ( 'NONE', *, *, #15788, .F. ) ;
#34853=ORIENTED_EDGE ( 'NONE', *, *, #7992, .F. ) ;
#34854=CARTESIAN_POINT ( 'NONE',  ( 185.0000000000000000, -5.999999999999950262, -340.0000000000001137 ) ) ;
#34856=ORIENTED_EDGE ( 'NONE', *, *, #24300, .T. ) ;
#34859=VERTEX_POINT ( 'NONE', #10968 ) ;
#34860=FACE_OUTER_BOUND ( 'NONE', #37887, .T. ) ;
#34867=DIRECTION ( 'NONE',  ( -1.000000000000000000, 0.000000000000000000, -1.612977847700450206E-50 ) ) ;
#34869=VECTOR ( 'NONE', #23984, 1000.000000000000000 ) ;
#34870=ORIENTED_EDGE ( 'NONE', *, *, #28012, .F. ) ;
#34877=AXIS2_PLACEMENT_3D ( 'NONE', #27043, #42681, #38866 ) ;
#34887=FACE_OUTER_BOUND ( 'NONE', #25866, .T. ) ;
#34894=ORIENTED_EDGE ( 'NONE', *, *, #41074, .T. ) ;
#34895=CARTESIAN_POINT ( 'NONE',  ( 344.0000000000000000, 165.0000000000000000, -94.00000000000019895 ) ) ;
#34905=CARTESIAN_POINT ( 'NONE',  ( 168.9999999999999716, -164.9999999999999432, -340.0000000000001137 ) ) ;
#34907=CARTESIAN_POINT ( 'NONE',  ( 168.9999999999999716, -174.9999999999999716, -358.0000000000001705 ) ) ;
#34909=LINE ( 'NONE', #39007, #11436 ) ;
#34910=VECTOR ( 'NONE', #42466, 1000.000000000000000 ) ;
#34911=EDGE_LOOP ( 'NONE', ( #19054, #4236, #44779, #26651 ) ) ;
#34912=CARTESIAN_POINT ( 'NONE',  ( 343.9999999999998863, -165.0000000000001137, -92.00000000000019895 ) ) ;
#34913=DIRECTION ( 'NONE',  ( 0.000000000000000000, -1.000000000000000000, 0.000000000000000000 ) ) ;
#34914=EDGE_CURVE ( 'NONE', #22581, #46047, #31248, .T. ) ;
#34922=VERTEX_POINT ( 'NONE', #13434 ) ;
#34923=CARTESIAN_POINT ( 'NONE',  ( 339.9999999999999432, -168.9999999999999432, -344.0000000000001705 ) ) ;
#34939=ORIENTED_EDGE ( 'NONE', *, *, #19663, .T. ) ;
#34941=CARTESIAN_POINT ( 'NONE',  ( 181.0000000000000000, -97.49999999999997158, -115.0000000000001563 ) ) ;
#34942=ORIENTED_EDGE ( 'NONE', *, *, #5509, .T. ) ;
#34944=DIRECTION ( 'NONE',  ( 0.000000000000000000, 1.000000000000000000, 6.123233995736766036E-17 ) ) ;
#34954=( LENGTH_UNIT ( ) NAMED_UNIT ( * ) SI_UNIT ( .MILLI., .METRE. ) );
#34956=ORIENTED_EDGE ( 'NONE', *, *, #15224, .T. ) ;
#34958=EDGE_LOOP ( 'NONE', ( #6102, #4633, #7660, #21404, #45181, #40823, #17257, #32764 ) ) ;
#34960=DIRECTION ( 'NONE',  ( 0.000000000000000000, -1.000000000000000000, 2.537652627714643577E-15 ) ) ;
#34965=( NAMED_UNIT ( * ) PLANE_ANGLE_UNIT ( ) SI_UNIT ( $, .RADIAN. ) );
#34976=CIRCLE ( 'NONE', #34117, 4.000000000000003553 ) ;
#34979=PLANE ( 'NONE',  #34374 ) ;
#34984=CARTESIAN_POINT ( 'NONE',  ( 168.9999999999999716, 6.000000000000060396, -340.0000000000001137 ) ) ;
#34989=ORIENTED_EDGE ( 'NONE', *, *, #9665, .T. ) ;
#34990=CYLINDRICAL_SURFACE ( 'NONE', #43478, 4.000000000000003553 ) ;
#34995=VERTEX_POINT ( 'NONE', #1146 ) ;
#34996=DIRECTION ( 'NONE',  ( 0.000000000000000000, 1.000000000000000000, 0.000000000000000000 ) ) ;
#35002=ORIENTED_EDGE ( 'NONE', *, *, #31964, .T. ) ;
#35005=CARTESIAN_POINT ( 'NONE',  ( 0.000000000000000000, -180.9999999999999716, -340.0000000000001705 ) ) ;
#35007=CARTESIAN_POINT ( 'NONE',  ( 339.9999999999999432, 169.0000000000000000, -356.0000000000002274 ) ) ;
#35011=DIRECTION ( 'NONE',  ( 1.000000000000000000, 0.000000000000000000, 0.000000000000000000 ) ) ;
#35017=ORIENTED_EDGE ( 'NONE', *, *, #12340, .F. ) ;
#35019=( NAMED_UNIT ( * ) PLANE_ANGLE_UNIT ( ) SI_UNIT ( $, .RADIAN. ) );
#35025=ORIENTED_EDGE ( 'NONE', *, *, #19952, .T. ) ;
#35026=DIRECTION ( 'NONE',  ( 1.000000000000000000, 0.000000000000000000, 0.000000000000000000 ) ) ;
#35027=FACE_BOUND ( 'NONE', #286, .T. ) ;
#35029=DIRECTION ( 'NONE',  ( 1.000000000000000000, 0.000000000000000000, -1.586032892321651989E-16 ) ) ;
#35031=EDGE_CURVE ( 'NONE', #23937, #13514, #1702, .T. ) ;
#35038=FACE_OUTER_BOUND ( 'NONE', #47577, .T. ) ;
#35041=DIRECTION ( 'NONE',  ( 1.000000000000000000, 0.000000000000000000, 0.000000000000000000 ) ) ;
#35044=EDGE_CURVE ( 'NONE', #913, #32935, #22393, .T. ) ;
#35049=CARTESIAN_POINT ( 'NONE',  ( 340.0000000000000568, 169.0000000000000000, 341.9999999999997726 ) ) ;
#35051=CARTESIAN_POINT ( 'NONE',  ( 356.0000000000001137, 183.0000000000000284, 357.9999999999998295 ) ) ;
#35059=VECTOR ( 'NONE', #46315, 1000.000000000000000 ) ;
#35067=ORIENTED_EDGE ( 'NONE', *, *, #22515, .F. ) ;
#35075=CARTESIAN_POINT ( 'NONE',  ( 344.0000000000000000, 175.0000000000000284, -106.0000000000001990 ) ) ;
#35081=DIRECTION ( 'NONE',  ( 1.333906992743555050E-23, -1.000000000000000000, 0.000000000000000000 ) ) ;
#35101=ORIENTED_EDGE ( 'NONE', *, *, #49014, .T. ) ;
#35103=CARTESIAN_POINT ( 'NONE',  ( 350.0000000000000000, -164.9999999999999432, -356.0000000000002274 ) ) ;
#35109=VERTEX_POINT ( 'NONE', #32128 ) ;
#35113=ORIENTED_EDGE ( 'NONE', *, *, #25661, .F. ) ;
#35118=ADVANCED_FACE ( 'NONE', ( #39585 ), #34990, .T. ) ;
#35130=VECTOR ( 'NONE', #42437, 1000.000000000000000 ) ;
#35132=CARTESIAN_POINT ( 'NONE',  ( 344.0000000000000568, 165.0000000000000000, 349.9999999999998295 ) ) ;
#35136=CARTESIAN_POINT ( 'NONE',  ( 0.000000000000000000, -168.9999999999999432, -356.0000000000002274 ) ) ;
#35137=EDGE_CURVE ( 'NONE', #14362, #38591, #8280, .T. ) ;
#35139=EDGE_LOOP ( 'NONE', ( #31685, #3511, #31221, #30346 ) ) ;
#35143=DIRECTION ( 'NONE',  ( 0.000000000000000000, 1.000000000000000000, 1.544785076050074834E-48 ) ) ;
#35146=LINE ( 'NONE', #11523, #11823 ) ;
#35151=DIRECTION ( 'NONE',  ( -1.000000000000000000, 0.000000000000000000, -2.958228394578794270E-31 ) ) ;
#35161=ORIENTED_EDGE ( 'NONE', *, *, #35044, .T. ) ;
#35166=ORIENTED_EDGE ( 'NONE', *, *, #49394, .F. ) ;
#35168=CARTESIAN_POINT ( 'NONE',  ( 358.0000000000000000, -168.9999999999999432, 343.9999999999998295 ) ) ;
#35170=ORIENTED_EDGE ( 'NONE', *, *, #48539, .T. ) ;
#35172=CLOSED_SHELL ( 'NONE', ( #46829, #50030, #25242, #19088, #14224, #23466, #15357, #30019 ) ) ;
#35189=DIRECTION ( 'NONE',  ( 1.000000000000000000, 0.000000000000000000, -0.000000000000000000 ) ) ;
#35194=DIRECTION ( 'NONE',  ( -1.586032892321652236E-16, -1.000000000000000000, -2.288264760618012091E-48 ) ) ;
#35201=AXIS2_PLACEMENT_3D ( 'NONE', #46425, #50002, #42849 ) ;
#35205=ORIENTED_EDGE ( 'NONE', *, *, #813, .T. ) ;
#35207=CIRCLE ( 'NONE', #13054, 4.000000000000003553 ) ;
#35209=CYLINDRICAL_SURFACE ( 'NONE', #31621, 4.000000000000003553 ) ;
#35211=CARTESIAN_POINT ( 'NONE',  ( 4.999999999999999112, 175.0000000000000284, -346.2500000000002274 ) ) ;
#35216=LINE ( 'NONE', #11854, #7803 ) ;
#35217=VERTEX_POINT ( 'NONE', #3655 ) ;
#35218=( NAMED_UNIT ( * ) PLANE_ANGLE_UNIT ( ) SI_UNIT ( $, .RADIAN. ) );
#35219=ORIENTED_EDGE ( 'NONE', *, *, #17977, .F. ) ;
#35222=ORIENTED_EDGE ( 'NONE', *, *, #32557, .T. ) ;
#35229=CIRCLE ( 'NONE', #49901, 4.000000000000003553 ) ;
#35230=AXIS2_PLACEMENT_3D ( 'NONE', #128, #47537, #12417 ) ;
#35233=ORIENTED_EDGE ( 'NONE', *, *, #31869, .T. ) ;
#35243=EDGE_LOOP ( 'NONE', ( #50472, #25697, #45618, #45915 ) ) ;
#35244=FACE_OUTER_BOUND ( 'NONE', #24675, .T. ) ;
#35251=EDGE_CURVE ( 'NONE', #50485, #34472, #42897, .T. ) ;
#35253=EDGE_CURVE ( 'NONE', #32679, #14457, #4172, .T. ) ;
#35254=CARTESIAN_POINT ( 'NONE',  ( 342.0000000000000568, 169.0000000000000000, 343.9999999999998863 ) ) ;
#35262=DIRECTION ( 'NONE',  ( 0.000000000000000000, -1.000000000000000000, -1.544785076050074834E-48 ) ) ;
#35263=EDGE_CURVE ( 'NONE', #6656, #24412, #11035, .T. ) ;
#35265=DIRECTION ( 'NONE',  ( 1.000000000000000000, -1.586032892321652236E-16, -9.711650524620651178E-33 ) ) ;
#35271=PLANE ( 'NONE',  #48210 ) ;
#35272=DIRECTION ( 'NONE',  ( -1.110223024625156171E-16, 0.7071067811865474617, -0.7071067811865474617 ) ) ;
#35276=FACE_OUTER_BOUND ( 'NONE', #50060, .T. ) ;
#35278=ORIENTED_EDGE ( 'NONE', *, *, #29294, .F. ) ;
#35280=CIRCLE ( 'NONE', #4128, 2.000000000000001776 ) ;
#35281=CIRCLE ( 'NONE', #40377, 4.000000000000003553 ) ;
#35294=EDGE_CURVE ( 'NONE', #30988, #32259, #15650, .T. ) ;
#35295=CYLINDRICAL_SURFACE ( 'NONE', #38608, 2.000000000000001776 ) ;
#35300=ORIENTED_EDGE ( 'NONE', *, *, #10867, .F. ) ;
#35304=CARTESIAN_POINT ( 'NONE',  ( 0.000000000000000000, 181.0000000000000284, 343.9999999999997726 ) ) ;
#35312=DIRECTION ( 'NONE',  ( -1.000000000000000000, -0.000000000000000000, -0.000000000000000000 ) ) ;
#35315=VERTEX_POINT ( 'NONE', #16722 ) ;
#35317=ORIENTED_EDGE ( 'NONE', *, *, #29133, .F. ) ;
#35319=AXIS2_PLACEMENT_3D ( 'NONE', #37001, #9262, #16701 ) ;
#35331=UNCERTAINTY_MEASURE_WITH_UNIT (LENGTH_MEASURE( 1.000000000000000082E-05 ), #46966, 'distance_accuracy_value', 'NONE');
#35337=VERTEX_POINT ( 'NONE', #5170 ) ;
#35344=VERTEX_POINT ( 'NONE', #1338 ) ;
#35345=DIRECTION ( 'NONE',  ( 1.000000000000000000, 0.000000000000000000, 0.000000000000000000 ) ) ;
#35349=AXIS2_PLACEMENT_3D ( 'NONE', #41905, #30886, #6751 ) ;
#35353=ORIENTED_EDGE ( 'NONE', *, *, #43560, .T. ) ;
#35355=EDGE_CURVE ( 'NONE', #26029, #22310, #48478, .T. ) ;
#35360=ADVANCED_FACE ( 'NONE', ( #42336 ), #26434, .F. ) ;
#35362=PLANE ( 'NONE',  #5975 ) ;
#35365=CARTESIAN_POINT ( 'NONE',  ( 181.0000000000000000, -5.999999999999950262, -340.0000000000001137 ) ) ;
#35369=PLANE ( 'NONE',  #33927 ) ;
#35374=EDGE_LOOP ( 'NONE', ( #43197, #44535, #38575, #30081 ) ) ;
#35376=DIRECTION ( 'NONE',  ( 1.000000000000000000, 0.000000000000000000, 0.000000000000000000 ) ) ;
#35377=LINE ( 'NONE', #24065, #31476 ) ;
#35381=LINE ( 'NONE', #27916, #29916 ) ;
#35382=FACE_OUTER_BOUND ( 'NONE', #11987, .T. ) ;
#35383=DIRECTION ( 'NONE',  ( -0.000000000000000000, -0.000000000000000000, 1.000000000000000000 ) ) ;
#35386=DIRECTION ( 'NONE',  ( -1.000000000000000000, 0.000000000000000000, 0.000000000000000000 ) ) ;
#35395=DIRECTION ( 'NONE',  ( 0.000000000000000000, -1.000000000000000000, 0.000000000000000000 ) ) ;
#35406=EDGE_CURVE ( 'NONE', #44300, #42814, #2574, .T. ) ;
#35408=DIRECTION ( 'NONE',  ( 1.000000000000000000, 0.000000000000000000, 0.000000000000000000 ) ) ;
#35411=AXIS2_PLACEMENT_3D ( 'NONE', #35716, #11579, #1043 ) ;
#35418=EDGE_LOOP ( 'NONE', ( #41591, #5111, #21830, #24756 ) ) ;
#35423=ORIENTED_EDGE ( 'NONE', *, *, #33426, .T. ) ;
#35434=CARTESIAN_POINT ( 'NONE',  ( 181.0000000000000000, -272.5000000000000000, -114.9999999999999147 ) ) ;
#35439=DIRECTION ( 'NONE',  ( 1.000000000000000000, 0.000000000000000000, 0.000000000000000000 ) ) ;
#35440=ORIENTED_EDGE ( 'NONE', *, *, #19340, .T. ) ;
#35447=CARTESIAN_POINT ( 'NONE',  ( 0.000000000000000000, -166.9999999999999432, -356.0000000000002274 ) ) ;
#35449=VECTOR ( 'NONE', #15508, 1000.000000000000000 ) ;
#35450=EDGE_CURVE ( 'NONE', #13304, #43357, #34165, .T. ) ;
#35453=CARTESIAN_POINT ( 'NONE',  ( 5.551115123125782702E-14, -182.9999999999999716, 355.9999999999997726 ) ) ;
#35455=AXIS2_PLACEMENT_3D ( 'NONE', #9721, #40283, #25139 ) ;
#35466=ORIENTED_EDGE ( 'NONE', *, *, #32419, .T. ) ;
#35467=CARTESIAN_POINT ( 'NONE',  ( 341.6568542494921417, -185.0000000000000568, 359.9999999999998295 ) ) ;
#35469=LINE ( 'NONE', #35734, #4833 ) ;
#35474=ORIENTED_EDGE ( 'NONE', *, *, #15577, .F. ) ;
#35480=FACE_OUTER_BOUND ( 'NONE', #45737, .T. ) ;
#35486=CARTESIAN_POINT ( 'NONE',  ( 358.3431457505075741, 185.0000000000001990, -360.0000000000003411 ) ) ;
#35488=CARTESIAN_POINT ( 'NONE',  ( 181.0000000000000000, -168.9999999999999432, -350.0000000000001705 ) ) ;
#35489=DIRECTION ( 'NONE',  ( 0.000000000000000000, 0.000000000000000000, 1.000000000000000000 ) ) ;
#35491=LINE ( 'NONE', #24441, #40608 ) ;
#35493=VERTEX_POINT ( 'NONE', #25691 ) ;
#35494=VERTEX_POINT ( 'NONE', #10784 ) ;
#35500=LINE ( 'NONE', #47991, #42827 ) ;
#35510=AXIS2_PLACEMENT_3D ( 'NONE', #5292, #42898, #26059 ) ;
#35514=( NAMED_UNIT ( * ) PLANE_ANGLE_UNIT ( ) SI_UNIT ( $, .RADIAN. ) );
#35515=CIRCLE ( 'NONE', #15016, 2.000000000000001776 ) ;
#35520=ORIENTED_EDGE ( 'NONE', *, *, #32507, .T. ) ;
#35527=PLANE ( 'NONE',  #47844 ) ;
#35536=( NAMED_UNIT ( * ) PLANE_ANGLE_UNIT ( ) SI_UNIT ( $, .RADIAN. ) );
#35540=CARTESIAN_POINT ( 'NONE',  ( 355.9999999999999432, 185.0000000000002274, -360.0000000000003411 ) ) ;
#35544=CIRCLE ( 'NONE', #42911, 4.000000000000003553 ) ;
#35556=ORIENTED_EDGE ( 'NONE', *, *, #44962, .T. ) ;
#35559=CARTESIAN_POINT ( 'NONE',  ( 340.0000000000000568, 183.0000000000000284, 343.9999999999997726 ) ) ;
#35561=CARTESIAN_POINT ( 'NONE',  ( 340.0000000000000568, 169.0000000000000000, 349.9999999999998295 ) ) ;
#35569=EDGE_LOOP ( 'NONE', ( #8969, #47163, #34894, #13181 ) ) ;
#35571=VECTOR ( 'NONE', #17005, 1000.000000000000000 ) ;
#35576=VERTEX_POINT ( 'NONE', #39524 ) ;
#35577=FACE_OUTER_BOUND ( 'NONE', #26263, .T. ) ;
#35586=DIRECTION ( 'NONE',  ( 1.000000000000000000, 0.000000000000000000, 0.000000000000000000 ) ) ;
#35592=ORIENTED_EDGE ( 'NONE', *, *, #12669, .T. ) ;
#35594=FACE_OUTER_BOUND ( 'NONE', #35243, .T. ) ;
#35605=LINE ( 'NONE', #4026, #33692 ) ;
#35606=EDGE_CURVE ( 'NONE', #3991, #25566, #26199, .T. ) ;
#35608=LINE ( 'NONE', #8646, #28104 ) ;
#35609=AXIS2_PLACEMENT_3D ( 'NONE', #23576, #12033, #12520 ) ;
#35619=CARTESIAN_POINT ( 'NONE',  ( 181.0000000000000000, -164.9999999999999432, 343.9999999999998863 ) ) ;
#35625=EDGE_CURVE ( 'NONE', #48047, #18735, #31578, .T. ) ;
#35630=AXIS2_PLACEMENT_3D ( 'NONE', #1609, #1358, #20590 ) ;
#35631=CARTESIAN_POINT ( 'NONE',  ( 164.9999999999999716, 165.0000000000000000, -344.0000000000001137 ) ) ;
#35632=CARTESIAN_POINT ( 'NONE',  ( 344.0000000000000000, 174.9999999999996874, -342.0000000000002842 ) ) ;
#35649=ORIENTED_EDGE ( 'NONE', *, *, #49062, .T. ) ;
#35664=LINE ( 'NONE', #31552, #11860 ) ;
#35691=FACE_OUTER_BOUND ( 'NONE', #37830, .T. ) ;
#35696=VECTOR ( 'NONE', #22124, 1000.000000000000000 ) ;
#35700=CYLINDRICAL_SURFACE ( 'NONE', #21813, 4.000000000000003553 ) ;
#35704=EDGE_LOOP ( 'NONE', ( #19696, #18642, #11263, #35786 ) ) ;
#35705=CARTESIAN_POINT ( 'NONE',  ( 164.9999999999999716, 6.000000000000060396, -350.0000000000001705 ) ) ;
#35706=ADVANCED_FACE ( 'NONE', ( #8729 ), #48667, .T. ) ;
#35708=CARTESIAN_POINT ( 'NONE',  ( 340.0000000000000568, 169.0000000000000284, 343.9999999999998295 ) ) ;
#35709=EDGE_LOOP ( 'NONE', ( #27893, #25105, #48373, #32582 ) ) ;
#35712=EDGE_CURVE ( 'NONE', #21405, #7855, #20509, .T. ) ;
#35716=CARTESIAN_POINT ( 'NONE',  ( 344.0000000000000000, 174.9999999999996589, -340.0000000000002842 ) ) ;
#35727=VECTOR ( 'NONE', #38327, 1000.000000000000000 ) ;
#35728=CARTESIAN_POINT ( 'NONE',  ( 183.0000000000000000, 165.0000000000000000, -344.0000000000001137 ) ) ;
#35729=AXIS2_PLACEMENT_3D ( 'NONE', #11688, #10671, #3467 ) ;
#35734=CARTESIAN_POINT ( 'NONE',  ( 168.9999999999999716, -97.49999999999998579, -350.0000000000001705 ) ) ;
#35736=CARTESIAN_POINT ( 'NONE',  ( 356.0000000000000000, 165.0000000000000000, -106.0000000000001990 ) ) ;
#35739=VERTEX_POINT ( 'NONE', #20756 ) ;
#35746=VECTOR ( 'NONE', #35345, 1000.000000000000000 ) ;
#35748=EDGE_CURVE ( 'NONE', #49664, #3886, #15539, .T. ) ;
#35751=CARTESIAN_POINT ( 'NONE',  ( 0.000000000000000000, 181.0000000000000284, -360.0000000000002274 ) ) ;
#35753=DIRECTION ( 'NONE',  ( 1.132880637372608740E-16, 4.718402560806925739E-50, 1.000000000000000000 ) ) ;
#35756=CARTESIAN_POINT ( 'NONE',  ( 168.9999999999999716, -168.9999999999999432, -350.0000000000001705 ) ) ;
#35757=ORIENTED_EDGE ( 'NONE', *, *, #24268, .T. ) ;
#35763=ADVANCED_FACE ( 'NONE', ( #24867 ), #32834, .F. ) ;
#35764=CARTESIAN_POINT ( 'NONE',  ( 5.551115123125782702E-14, -180.9999999999999716, 343.9999999999997726 ) ) ;
#35769=ORIENTED_EDGE ( 'NONE', *, *, #7571, .F. ) ;
#35776=ORIENTED_EDGE ( 'NONE', *, *, #37506, .T. ) ;
#35778=VECTOR ( 'NONE', #7428, 1000.000000000000000 ) ;
#35783=CARTESIAN_POINT ( 'NONE',  ( 165.0000000000000000, 2.775557561562891351E-14, -99.00000000000014211 ) ) ;
#35784=ORIENTED_EDGE ( 'NONE', *, *, #5509, .F. ) ;
#35786=ORIENTED_EDGE ( 'NONE', *, *, #3598, .F. ) ;
#35788=CARTESIAN_POINT ( 'NONE',  ( 181.0000000000000000, -93.49999999999998579, -340.0000000000001137 ) ) ;
#35789=ORIENTED_EDGE ( 'NONE', *, *, #38139, .T. ) ;
#35793=CARTESIAN_POINT ( 'NONE',  ( 168.9999999999999716, -164.9999999999999432, 343.9999999999998863 ) ) ;
#35795=FACE_OUTER_BOUND ( 'NONE', #41662, .T. ) ;
#35801=CARTESIAN_POINT ( 'NONE',  ( 164.9999999999999716, -180.9999999999999716, -340.0000000000001137 ) ) ;
#35803=DIRECTION ( 'NONE',  ( 0.000000000000000000, 3.186989995019654210E-49, 1.000000000000000000 ) ) ;
#35805=VECTOR ( 'NONE', #30703, 1000.000000000000000 ) ;
#35807=EDGE_LOOP ( 'NONE', ( #34795, #41669, #43662, #32258 ) ) ;
#35816=CARTESIAN_POINT ( 'NONE',  ( 181.0000000000000000, -254.5000000000000000, -114.9999999999999574 ) ) ;
#35818=ORIENTED_EDGE ( 'NONE', *, *, #9089, .T. ) ;
#35822=EDGE_LOOP ( 'NONE', ( #24496, #19338, #29008, #3708 ) ) ;
#35824=CARTESIAN_POINT ( 'NONE',  ( 181.0000000000000000, -272.4999999999999432, -357.9999999999999432 ) ) ;
#35826=CARTESIAN_POINT ( 'NONE',  ( 0.000000000000000000, 165.0000000000000000, 355.9999999999997726 ) ) ;
#35829=EDGE_LOOP ( 'NONE', ( #34000, #28232, #23661, #476, #28125, #22402, #19449, #26002 ) ) ;
#35835=EDGE_LOOP ( 'NONE', ( #9351, #40769, #5385, #8418, #19487, #16096, #35317, #47573 ) ) ;
#35837=CARTESIAN_POINT ( 'NONE',  ( 185.0000000000000284, -9.999999999999953815, -111.0000000000001563 ) ) ;
#35844=VERTEX_POINT ( 'NONE', #46087 ) ;
#35847=DIRECTION ( 'NONE',  ( 1.860490536778032451E-50, 0.000000000000000000, -1.000000000000000000 ) ) ;
#35852=CARTESIAN_POINT ( 'NONE',  ( 342.8284271247461561, -167.0000000000001137, -342.0000000000002842 ) ) ;
#35859=AXIS2_PLACEMENT_3D ( 'NONE', #20499, #36169, #6908 ) ;
#35869=DIRECTION ( 'NONE',  ( 0.000000000000000000, 0.000000000000000000, -1.000000000000000000 ) ) ;
#35873=CARTESIAN_POINT ( 'NONE',  ( 185.0000000000000000, 175.0000000000000284, -344.0000000000001137 ) ) ;
#35876=LINE ( 'NONE', #32532, #19417 ) ;
#35877=ORIENTED_EDGE ( 'NONE', *, *, #17092, .T. ) ;
#35882=ADVANCED_FACE ( 'NONE', ( #2765 ), #22524, .F. ) ;
#35898=DIRECTION ( 'NONE',  ( 0.000000000000000000, 1.000000000000000000, -2.537652627714643577E-15 ) ) ;
#35901=DIRECTION ( 'NONE',  ( 0.000000000000000000, 0.000000000000000000, 1.000000000000000000 ) ) ;
#35909=DIRECTION ( 'NONE',  ( 1.000000000000000000, 0.000000000000000000, 2.958228394578794270E-31 ) ) ;
#35914=EDGE_CURVE ( 'NONE', #10238, #30616, #43439, .T. ) ;
#35919=EDGE_CURVE ( 'NONE', #23987, #39539, #4907, .T. ) ;
#35921=CARTESIAN_POINT ( 'NONE',  ( 181.0000000000000000, -272.4999999999999432, -355.9999999999999432 ) ) ;
#35922=CARTESIAN_POINT ( 'NONE',  ( 183.0000000000000000, -180.9999999999999716, -350.0000000000001705 ) ) ;
#35923=ADVANCED_FACE ( 'NONE', ( #10475 ), #18163, .T. ) ;
#35925=( NAMED_UNIT ( * ) PLANE_ANGLE_UNIT ( ) SI_UNIT ( $, .RADIAN. ) );
#35927=VERTEX_POINT ( 'NONE', #30747 ) ;
#35930=ORIENTED_EDGE ( 'NONE', *, *, #24045, .F. ) ;
#35933=VERTEX_POINT ( 'NONE', #210 ) ;
#35939=ADVANCED_FACE ( 'NONE', ( #34860 ), #50696, .F. ) ;
#35951=EDGE_LOOP ( 'NONE', ( #36877, #24511, #10504, #33508 ) ) ;
#35952=DIRECTION ( 'NONE',  ( 1.000000000000000000, 0.000000000000000000, 0.000000000000000000 ) ) ;
#35954=DIRECTION ( 'NONE',  ( 0.000000000000000000, 3.186989995019654210E-49, 1.000000000000000000 ) ) ;
#35958=EDGE_CURVE ( 'NONE', #36804, #16909, #19439, .T. ) ;
#35964=CARTESIAN_POINT ( 'NONE',  ( 349.9999999999999432, -184.9999999999999716, 355.9999999999997726 ) ) ;
#35967=ADVANCED_FACE ( 'NONE', ( #4046 ), #38698, .F. ) ;
#35970=VERTEX_POINT ( 'NONE', #3269 ) ;
#35972=DIRECTION ( 'NONE',  ( 0.000000000000000000, 5.664403186863042467E-17, 1.000000000000000000 ) ) ;
#35979=ORIENTED_EDGE ( 'NONE', *, *, #46870, .F. ) ;
#35983=FACE_OUTER_BOUND ( 'NONE', #36563, .T. ) ;
#35985=CARTESIAN_POINT ( 'NONE',  ( 339.9999999999999432, -166.6568542494925111, 341.6568542494923690 ) ) ;
#35986=PLANE ( 'NONE',  #39485 ) ;
#35992=CARTESIAN_POINT ( 'NONE',  ( 349.9999999999999432, -180.9999999999999716, 359.9999999999997726 ) ) ;
#35995=DIRECTION ( 'NONE',  ( 1.000000000000000000, -4.996003610813203446E-16, -7.930164450086814785E-16 ) ) ;
#35999=EDGE_CURVE ( 'NONE', #31506, #42696, #15597, .T. ) ;
#36004=VECTOR ( 'NONE', #13607, 1000.000000000000000 ) ;
#36007=LINE ( 'NONE', #24701, #48832 ) ;
#36009=ORIENTED_EDGE ( 'NONE', *, *, #19414, .T. ) ;
#36013=AXIS2_PLACEMENT_3D ( 'NONE', #18703, #23067, #38741 ) ;
#36014=PLANE ( 'NONE',  #42283 ) ;
#36019=ORIENTED_EDGE ( 'NONE', *, *, #42774, .F. ) ;
#36020=DIRECTION ( 'NONE',  ( 3.172065745548403743E-16, 1.000000000000000000, 0.000000000000000000 ) ) ;
#36030=DIRECTION ( 'NONE',  ( 0.000000000000000000, 1.000000000000000000, 0.000000000000000000 ) ) ;
#36033=DIRECTION ( 'NONE',  ( 0.000000000000000000, 0.000000000000000000, -1.000000000000000000 ) ) ;
#36035=DIRECTION ( 'NONE',  ( -1.000000000000000000, 0.000000000000000000, -7.793956916774525800E-48 ) ) ;
#36036=CARTESIAN_POINT ( 'NONE',  ( 340.0000000000000568, 181.0000000000000284, 341.9999999999997726 ) ) ;
#36042=FACE_OUTER_BOUND ( 'NONE', #25974, .T. ) ;
#36043=EDGE_LOOP ( 'NONE', ( #25268, #19662, #1655, #10361 ) ) ;
#36045=DIRECTION ( 'NONE',  ( 1.586032892321652236E-16, 1.000000000000000000, 6.853681917100419162E-49 ) ) ;
#36046=ADVANCED_FACE ( 'NONE', ( #23275 ), #3790, .F. ) ;
#36050=ORIENTED_EDGE ( 'NONE', *, *, #30285, .T. ) ;
#36057=ORIENTED_EDGE ( 'NONE', *, *, #5899, .T. ) ;
#36070=AXIS2_PLACEMENT_3D ( 'NONE', #22508, #3776, #47846 ) ;
#36072=AXIS2_PLACEMENT_3D ( 'NONE', #28575, #48030, #5981 ) ;
#36074=EDGE_LOOP ( 'NONE', ( #8110, #35205, #481, #30305, #43411, #11185, #45466, #35423 ) ) ;
#36075=ORIENTED_EDGE ( 'NONE', *, *, #30543, .F. ) ;
#36076=DIRECTION ( 'NONE',  ( 0.000000000000000000, 0.000000000000000000, -1.000000000000000000 ) ) ;
#36077=CIRCLE ( 'NONE', #11447, 2.000000000000001776 ) ;
#36081=CIRCLE ( 'NONE', #36936, 4.000000000000003553 ) ;
#36083=ORIENTED_EDGE ( 'NONE', *, *, #14902, .F. ) ;
#36085=ADVANCED_FACE ( 'NONE', ( #8666 ), #12492, .F. ) ;
#36088=ORIENTED_EDGE ( 'NONE', *, *, #7333, .T. ) ;
#36092=CARTESIAN_POINT ( 'NONE',  ( 350.0000000000000000, 185.0000000000000284, -356.0000000000002274 ) ) ;
#36093=LINE ( 'NONE', #32234, #47810 ) ;
#36103=DIRECTION ( 'NONE',  ( 1.000000000000000000, 0.000000000000000000, 0.000000000000000000 ) ) ;
#36106=ORIENTED_EDGE ( 'NONE', *, *, #13274, .F. ) ;
#36116=EDGE_LOOP ( 'NONE', ( #29602, #9331, #41988, #22672 ) ) ;
#36125=VERTEX_POINT ( 'NONE', #8413 ) ;
#36141=CIRCLE ( 'NONE', #13982, 4.000000000000003553 ) ;
#36143=CARTESIAN_POINT ( 'NONE',  ( 181.0000000000000000, -268.4999999999999432, -339.9999999999998863 ) ) ;
#36144=CARTESIAN_POINT ( 'NONE',  ( 356.0000000000001137, -166.9999999999999432, 341.9999999999998295 ) ) ;
#36145=VECTOR ( 'NONE', #11354, 1000.000000000000000 ) ;
#36148=CARTESIAN_POINT ( 'NONE',  ( 183.0000000000000000, -164.9999999999999432, -356.0000000000001705 ) ) ;
#36152=AXIS2_PLACEMENT_3D ( 'NONE', #26365, #42009, #6862 ) ;
#36155=CARTESIAN_POINT ( 'NONE',  ( 181.0000000000000284, -180.9999999999999716, -115.0000000000001279 ) ) ;
#36163=CARTESIAN_POINT ( 'NONE',  ( 168.9999999999999716, -268.4999999999999432, -349.9999999999999432 ) ) ;
#36168=DIRECTION ( 'NONE',  ( -1.000000000000000000, 0.000000000000000000, 0.000000000000000000 ) ) ;
#36169=DIRECTION ( 'NONE',  ( 1.333906992743555050E-23, -1.000000000000000000, 0.000000000000000000 ) ) ;
#36171=CARTESIAN_POINT ( 'NONE',  ( 181.0000000000000000, 8.000000000000062172, -350.0000000000001705 ) ) ;
#36172=ORIENTED_EDGE ( 'NONE', *, *, #49084, .T. ) ;
#36173=ORIENTED_EDGE ( 'NONE', *, *, #43441, .F. ) ;
#36175=AXIS2_PLACEMENT_3D ( 'NONE', #35304, #3454, #31191 ) ;
#36177=ORIENTED_EDGE ( 'NONE', *, *, #2719, .T. ) ;
#36179=DIRECTION ( 'NONE',  ( 0.000000000000000000, 2.537652627714642000E-15, 1.000000000000000000 ) ) ;
#36187=LINE ( 'NONE', #8735, #25138 ) ;
#36190=LINE ( 'NONE', #48176, #37904 ) ;
#36191=EDGE_CURVE ( 'NONE', #27608, #23039, #44280, .T. ) ;
#36192=ORIENTED_EDGE ( 'NONE', *, *, #23396, .T. ) ;
#36197=DIRECTION ( 'NONE',  ( -1.000000000000000000, -6.344131455081961406E-16, 4.759647537211363479E-16 ) ) ;
#36204=DIRECTION ( 'NONE',  ( -1.000000000000000000, 0.000000000000000000, 1.860490536778032451E-50 ) ) ;
#36212=CIRCLE ( 'NONE', #27189, 2.000000000000001776 ) ;
#36213=FACE_OUTER_BOUND ( 'NONE', #20376, .T. ) ;
#36221=ORIENTED_EDGE ( 'NONE', *, *, #5899, .F. ) ;
#36223=LINE ( 'NONE', #40315, #40886 ) ;
#36224=AXIS2_PLACEMENT_3D ( 'NONE', #35365, #50679, #4032 ) ;
#36234=VERTEX_POINT ( 'NONE', #37888 ) ;
#36246=DIRECTION ( 'NONE',  ( 0.000000000000000000, 1.000000000000000000, 0.000000000000000000 ) ) ;
#36248=DIRECTION ( 'NONE',  ( -1.000000000000000000, -0.000000000000000000, -0.000000000000000000 ) ) ;
#36249=VECTOR ( 'NONE', #24150, 1000.000000000000000 ) ;
#36251=ORIENTED_EDGE ( 'NONE', *, *, #31857, .T. ) ;
#36256=AXIS2_PLACEMENT_3D ( 'NONE', #23361, #16176, #19496 ) ;
#36274=ADVANCED_FACE ( 'NONE', ( #3979 ), #19112, .F. ) ;
#36278=EDGE_CURVE ( 'NONE', #35739, #29362, #18850, .T. ) ;
#36279=ORIENTED_EDGE ( 'NONE', *, *, #2424, .F. ) ;
#36280=DIRECTION ( 'NONE',  ( -1.000000000000000000, 0.000000000000000000, 1.860490536778032451E-50 ) ) ;
#36284=ORIENTED_EDGE ( 'NONE', *, *, #38250, .T. ) ;
#36288=PLANE ( 'NONE',  #16038 ) ;
#36294=DIRECTION ( 'NONE',  ( 0.000000000000000000, 1.000000000000000000, 0.000000000000000000 ) ) ;
#36295=CIRCLE ( 'NONE', #14124, 4.000000000000003553 ) ;
#36296=LINE ( 'NONE', #44200, #25285 ) ;
#36297=DIRECTION ( 'NONE',  ( -9.711650524620651178E-33, 1.223873602809432483E-48, -1.000000000000000000 ) ) ;
#36302=VERTEX_POINT ( 'NONE', #46783 ) ;
#36313=ORIENTED_EDGE ( 'NONE', *, *, #44291, .T. ) ;
#36314=ORIENTED_EDGE ( 'NONE', *, *, #47983, .F. ) ;
#36316=CARTESIAN_POINT ( 'NONE',  ( 169.0000000000000284, 175.0000000000000284, 359.9999999999998863 ) ) ;
#36337=ORIENTED_EDGE ( 'NONE', *, *, #36562, .T. ) ;
#36342=ORIENTED_EDGE ( 'NONE', *, *, #29644, .T. ) ;
#36346=FACE_BOUND ( 'NONE', #17472, .T. ) ;
#36348=ORIENTED_EDGE ( 'NONE', *, *, #36590, .T. ) ;
#36351=CYLINDRICAL_SURFACE ( 'NONE', #29780, 4.000000000000003553 ) ;
#36352=EDGE_CURVE ( 'NONE', #15608, #8293, #19856, .T. ) ;
#36363=AXIS2_PLACEMENT_3D ( 'NONE', #5720, #17783, #21369 ) ;
#36370=DIRECTION ( 'NONE',  ( -3.172065784643302499E-16, -1.000000000000000000, 2.537652627714642000E-15 ) ) ;
#36373=ORIENTED_EDGE ( 'NONE', *, *, #2693, .T. ) ;
#36387=FACE_OUTER_BOUND ( 'NONE', #30362, .T. ) ;
#36391=CARTESIAN_POINT ( 'NONE',  ( 350.0000000000001137, 167.0000000000000000, 343.9999999999997726 ) ) ;
#36405=EDGE_CURVE ( 'NONE', #20673, #47737, #28095, .T. ) ;
#36408=FACE_OUTER_BOUND ( 'NONE', #2051, .T. ) ;
#36409=DIRECTION ( 'NONE',  ( 0.000000000000000000, 0.000000000000000000, -1.000000000000000000 ) ) ;
#36410=EDGE_CURVE ( 'NONE', #6960, #15590, #5935, .T. ) ;
#36416=AXIS2_PLACEMENT_3D ( 'NONE', #36921, #36671, #48386 ) ;
#36423=ORIENTED_EDGE ( 'NONE', *, *, #19252, .T. ) ;
#36424=CARTESIAN_POINT ( 'NONE',  ( 183.0000000000000284, -180.9999999999999716, -115.0000000000001279 ) ) ;
#36429=VECTOR ( 'NONE', #9020, 1000.000000000000000 ) ;
#36430=PLANE ( 'NONE',  #33169 ) ;
#36431=CARTESIAN_POINT ( 'NONE',  ( 168.9999999999998579, -166.9999999999999432, -340.0000000000001137 ) ) ;
#36442=CARTESIAN_POINT ( 'NONE',  ( 360.0000000000000000, -169.0000000000000568, -344.0000000000002842 ) ) ;
#36447=PLANE ( 'NONE',  #35455 ) ;
#36448=VECTOR ( 'NONE', #1190, 1000.000000000000000 ) ;
#36450=CARTESIAN_POINT ( 'NONE',  ( 164.9999999999999716, -9.999999999999953815, -350.0000000000001705 ) ) ;
#36451=CARTESIAN_POINT ( 'NONE',  ( 358.0000000000000000, -169.0000000000001137, -344.0000000000002842 ) ) ;
#36457=EDGE_LOOP ( 'NONE', ( #15710, #48499, #6836, #6447 ) ) ;
#36459=DIRECTION ( 'NONE',  ( -0.000000000000000000, -3.186989995019654210E-49, -1.000000000000000000 ) ) ;
#36460=DIRECTION ( 'NONE',  ( 0.000000000000000000, -2.537652627714643577E-15, -1.000000000000000000 ) ) ;
#36475=CARTESIAN_POINT ( 'NONE',  ( 344.0000000000000568, -167.0000000000001137, 342.0000000000000000 ) ) ;
#36479=DIRECTION ( 'NONE',  ( 7.793956916774525800E-48, 0.000000000000000000, 1.000000000000000000 ) ) ;
#36483=VECTOR ( 'NONE', #38950, 1000.000000000000000 ) ;
#36486=DIRECTION ( 'NONE',  ( 1.000000000000000000, -1.586032892321652236E-16, -1.586032892321651989E-16 ) ) ;
#36488=VERTEX_POINT ( 'NONE', #16800 ) ;
#36489=DIRECTION ( 'NONE',  ( 0.000000000000000000, 2.537652627714642000E-15, 1.000000000000000000 ) ) ;
#36491=EDGE_CURVE ( 'NONE', #48821, #8324, #8353, .T. ) ;
#36494=EDGE_CURVE ( 'NONE', #32259, #47711, #1414, .T. ) ;
#36499=ORIENTED_EDGE ( 'NONE', *, *, #17362, .T. ) ;
#36509=CARTESIAN_POINT ( 'NONE',  ( 168.9999999999999716, -164.9999999999999432, 355.9999999999998863 ) ) ;
#36511=EDGE_LOOP ( 'NONE', ( #30756, #22158, #33849, #31268, #19066, #17723, #19186, #18488 ) ) ;
#36517=EDGE_CURVE ( 'NONE', #5465, #11313, #50127, .T. ) ;
#36518=CARTESIAN_POINT ( 'NONE',  ( 350.0000000000000000, -168.9999999999999432, -360.0000000000002274 ) ) ;
#36520=DIRECTION ( 'NONE',  ( -7.793956916774524585E-48, 0.000000000000000000, -1.000000000000000000 ) ) ;
#36526=ORIENTED_EDGE ( 'NONE', *, *, #10874, .T. ) ;
#36536=DIRECTION ( 'NONE',  ( -2.958228394578794708E-31, 0.000000000000000000, 1.000000000000000000 ) ) ;
#36537=EDGE_LOOP ( 'NONE', ( #26527, #11353, #26784, #7329 ) ) ;
#36540=CIRCLE ( 'NONE', #47127, 2.000000000000001776 ) ;
#36545=CIRCLE ( 'NONE', #21746, 3.749999999999975575 ) ;
#36546=CARTESIAN_POINT ( 'NONE',  ( 183.0000000000000000, -93.49999999999998579, -115.0000000000001563 ) ) ;
#36547=VERTEX_POINT ( 'NONE', #9603 ) ;
#36553=CIRCLE ( 'NONE', #45170, 4.000000000000003553 ) ;
#36562=EDGE_CURVE ( 'NONE', #12204, #5465, #11309, .T. ) ;
#36563=EDGE_LOOP ( 'NONE', ( #19336, #3252, #20164, #19953 ) ) ;
#36568=CARTESIAN_POINT ( 'NONE',  ( 169.0000000000000000, 2.775557561562891351E-14, -97.00000000000014211 ) ) ;
#36574=EDGE_CURVE ( 'NONE', #28586, #44854, #3343, .T. ) ;
#36581=ORIENTED_EDGE ( 'NONE', *, *, #22663, .F. ) ;
#36585=CARTESIAN_POINT ( 'NONE',  ( 356.0000000000000568, 185.0000000000001137, 359.9999999999998295 ) ) ;
#36586=VECTOR ( 'NONE', #15175, 1000.000000000000000 ) ;
#36587=ORIENTED_EDGE ( 'NONE', *, *, #15821, .F. ) ;
#36588=ORIENTED_EDGE ( 'NONE', *, *, #35253, .F. ) ;
#36590=EDGE_CURVE ( 'NONE', #269, #39568, #40344, .T. ) ;
#36591=AXIS2_PLACEMENT_3D ( 'NONE', #20435, #35869, #697 ) ;
#36597=ORIENTED_EDGE ( 'NONE', *, *, #3692, .T. ) ;
#36599=CARTESIAN_POINT ( 'NONE',  ( 355.9999999999999432, -185.0000000000000284, 359.9999999999998295 ) ) ;
#36605=CIRCLE ( 'NONE', #43126, 4.000000000000003553 ) ;
#36608=CARTESIAN_POINT ( 'NONE',  ( 185.0000000000000000, 165.0000000000000000, -356.0000000000001705 ) ) ;
#36610=CARTESIAN_POINT ( 'NONE',  ( 183.0000000000000284, -180.9999999999993747, -115.0000000000001279 ) ) ;
#36611=AXIS2_PLACEMENT_3D ( 'NONE', #21722, #44114, #48879 ) ;
#36617=PLANE ( 'NONE',  #32341 ) ;
#36621=DIRECTION ( 'NONE',  ( 0.000000000000000000, 0.000000000000000000, 1.000000000000000000 ) ) ;
#36627=ORIENTED_EDGE ( 'NONE', *, *, #5195, .F. ) ;
#36628=CARTESIAN_POINT ( 'NONE',  ( 360.0000000000000568, 165.0000000000000000, -106.0000000000001990 ) ) ;
#36630=EDGE_CURVE ( 'NONE', #2449, #19301, #41979, .T. ) ;
#36633=CARTESIAN_POINT ( 'NONE',  ( 185.0000000000000284, -174.9999999999999716, -99.00000000000014211 ) ) ;
#36643=ADVANCED_FACE ( 'NONE', ( #43352 ), #31589, .T. ) ;
#36644=AXIS2_PLACEMENT_3D ( 'NONE', #22975, #28544, #11957 ) ;
#36650=ADVANCED_FACE ( 'NONE', ( #20273 ), #779, .F. ) ;
#36654=CARTESIAN_POINT ( 'NONE',  ( 185.0000000000000000, -5.999999999999950262, 339.9999999999998295 ) ) ;
#36657=DIRECTION ( 'NONE',  ( 1.000000000000000000, 0.000000000000000000, 0.000000000000000000 ) ) ;
#36658=( NAMED_UNIT ( * ) PLANE_ANGLE_UNIT ( ) SI_UNIT ( $, .RADIAN. ) );
#36659=ORIENTED_EDGE ( 'NONE', *, *, #22227, .T. ) ;
#36666=LINE ( 'NONE', #1490, #14312 ) ;
#36669=CARTESIAN_POINT ( 'NONE',  ( 357.1715728752537871, -183.0000000000000284, 357.9999999999998295 ) ) ;
#36671=DIRECTION ( 'NONE',  ( -1.000000000000000000, -0.000000000000000000, -0.000000000000000000 ) ) ;
#36674=CARTESIAN_POINT ( 'NONE',  ( 181.0000000000000284, -174.9999999999999716, -113.0000000000001563 ) ) ;
#36677=DIRECTION ( 'NONE',  ( 1.000000000000000000, 0.000000000000000000, 0.000000000000000000 ) ) ;
#36693=FACE_OUTER_BOUND ( 'NONE', #46033, .T. ) ;
#36696=ORIENTED_EDGE ( 'NONE', *, *, #25889, .T. ) ;
#36704=CARTESIAN_POINT ( 'NONE',  ( 349.9999999999999432, -184.9999999999999716, 343.9999999999997726 ) ) ;
#36706=ORIENTED_EDGE ( 'NONE', *, *, #27182, .F. ) ;
#36709=EDGE_CURVE ( 'NONE', #43962, #25778, #25576, .T. ) ;
#36710=CARTESIAN_POINT ( 'NONE',  ( 185.0000000000000284, 2.775557561562891351E-14, -99.00000000000014211 ) ) ;
#36713=ORIENTED_EDGE ( 'NONE', *, *, #48795, .T. ) ;
#36720=ORIENTED_EDGE ( 'NONE', *, *, #2424, .T. ) ;
#36722=CARTESIAN_POINT ( 'NONE',  ( 168.9999999999999716, 165.0000000000000000, -344.0000000000001137 ) ) ;
#36723=CARTESIAN_POINT ( 'NONE',  ( 355.9999999999999432, 183.0000000000002558, -358.0000000000003411 ) ) ;
#36727=DIRECTION ( 'NONE',  ( 1.000000000000000000, -0.000000000000000000, 0.000000000000000000 ) ) ;
#36731=EDGE_CURVE ( 'NONE', #40834, #18563, #20670, .T. ) ;
#36732=VECTOR ( 'NONE', #27040, 1000.000000000000000 ) ;
#36735=ADVANCED_FACE ( 'NONE', ( #7721, #38773 ), #27719, .T. ) ;
#36739=DIRECTION ( 'NONE',  ( -1.000000000000000000, 0.000000000000000000, -7.793956916774525800E-48 ) ) ;
#36742=ORIENTED_EDGE ( 'NONE', *, *, #37858, .F. ) ;
#36744=CARTESIAN_POINT ( 'NONE',  ( 185.0000000000000000, -174.9999999999999716, -356.0000000000001705 ) ) ;
#36745=DIRECTION ( 'NONE',  ( 0.000000000000000000, 0.000000000000000000, -1.000000000000000000 ) ) ;
#36768=CARTESIAN_POINT ( 'NONE',  ( 357.1715728752537302, -183.0000000000001705, -358.0000000000003411 ) ) ;
#36770=DIRECTION ( 'NONE',  ( 1.000000000000000000, 0.000000000000000000, -1.586032892321652482E-16 ) ) ;
#36771=DIRECTION ( 'NONE',  ( -1.000000000000000000, 0.000000000000000000, 0.000000000000000000 ) ) ;
#36772=ORIENTED_EDGE ( 'NONE', *, *, #23465, .F. ) ;
#36774=DIRECTION ( 'NONE',  ( 0.000000000000000000, 1.000000000000000000, -5.664403186863042467E-17 ) ) ;
#36775=DIRECTION ( 'NONE',  ( -1.000000000000000000, 0.000000000000000000, 0.000000000000000000 ) ) ;
#36781=FACE_OUTER_BOUND ( 'NONE', #31228, .T. ) ;
#36787=CARTESIAN_POINT ( 'NONE',  ( 169.0000000000000000, -272.5000000000000000, -94.99999999999988631 ) ) ;
#36791=DIRECTION ( 'NONE',  ( -0.000000000000000000, -6.123233995736766036E-17, 1.000000000000000000 ) ) ;
#36795=LINE ( 'NONE', #36546, #32182 ) ;
#36799=CARTESIAN_POINT ( 'NONE',  ( 0.000000000000000000, 185.0000000000000284, -356.0000000000002274 ) ) ;
#36803=CYLINDRICAL_SURFACE ( 'NONE', #27001, 2.000000000000001776 ) ;
#36804=VERTEX_POINT ( 'NONE', #31068 ) ;
#36810=VECTOR ( 'NONE', #34449, 1000.000000000000000 ) ;
#36811=EDGE_CURVE ( 'NONE', #18711, #3809, #46669, .T. ) ;
#36812=CARTESIAN_POINT ( 'NONE',  ( 168.9999999999999716, 8.000000000000062172, -350.0000000000001705 ) ) ;
#36814=DIRECTION ( 'NONE',  ( 0.000000000000000000, -2.537652627714643577E-15, -1.000000000000000000 ) ) ;
#36822=DIRECTION ( 'NONE',  ( 1.110223024625156171E-16, -0.7071067811865475727, -0.7071067811865475727 ) ) ;
#36828=ORIENTED_EDGE ( 'NONE', *, *, #12063, .T. ) ;
#36830=DIRECTION ( 'NONE',  ( -3.172065784643302499E-16, -1.000000000000000000, 2.537652627714642000E-15 ) ) ;
#36838=EDGE_CURVE ( 'NONE', #6015, #35970, #2032, .T. ) ;
#36839=DIRECTION ( 'NONE',  ( -1.000000000000000000, -0.000000000000000000, -0.000000000000000000 ) ) ;
#36840=ORIENTED_EDGE ( 'NONE', *, *, #13619, .T. ) ;
#36847=EDGE_CURVE ( 'NONE', #38131, #30152, #13064, .T. ) ;
#36854=DIRECTION ( 'NONE',  ( 0.000000000000000000, 0.000000000000000000, -1.000000000000000000 ) ) ;
#36855=EDGE_CURVE ( 'NONE', #23492, #50585, #36190, .T. ) ;
#36858=FACE_OUTER_BOUND ( 'NONE', #7242, .T. ) ;
#36860=AXIS2_PLACEMENT_3D ( 'NONE', #3707, #31174, #11665 ) ;
#36867=ADVANCED_FACE ( 'NONE', ( #32336 ), #36447, .F. ) ;
#36868=FACE_OUTER_BOUND ( 'NONE', #31556, .T. ) ;
#36871=VECTOR ( 'NONE', #31437, 1000.000000000000000 ) ;
#36872=CARTESIAN_POINT ( 'NONE',  ( 344.0000000000000000, -174.9999999999999432, 341.9999999999998295 ) ) ;
#36877=ORIENTED_EDGE ( 'NONE', *, *, #5123, .F. ) ;
#36879=ADVANCED_FACE ( 'NONE', ( #5619 ), #32591, .F. ) ;
#36880=EDGE_CURVE ( 'NONE', #3051, #21391, #48924, .T. ) ;
#36886=CYLINDRICAL_SURFACE ( 'NONE', #6038, 4.000000000000003553 ) ;
#36901=DIRECTION ( 'NONE',  ( 1.000000000000000000, 0.000000000000000000, 0.000000000000000000 ) ) ;
#36905=ORIENTED_EDGE ( 'NONE', *, *, #21401, .F. ) ;
#36913=CARTESIAN_POINT ( 'NONE',  ( 185.0000000000000000, -164.9999999999999432, 343.9999999999998863 ) ) ;
#36921=CARTESIAN_POINT ( 'NONE',  ( 4.999999999999999112, 175.0000000000000284, 350.0000000000002274 ) ) ;
#36936=AXIS2_PLACEMENT_3D ( 'NONE', #3292, #22799, #7670 ) ;
#36939=CARTESIAN_POINT ( 'NONE',  ( 356.0000000000000000, -165.0000000000001137, -340.0000000000002842 ) ) ;
#36943=CARTESIAN_POINT ( 'NONE',  ( 181.0000000000000000, -272.4999999999999432, -343.9999999999999432 ) ) ;
#36962=CARTESIAN_POINT ( 'NONE',  ( 350.0000000000000000, -168.9999999999999432, -360.0000000000002274 ) ) ;
#36967=FACE_OUTER_BOUND ( 'NONE', #23769, .T. ) ;
#36977=PLANE ( 'NONE',  #49288 ) ;
#36982=EDGE_CURVE ( 'NONE', #16242, #49685, #1885, .T. ) ;
#36985=ORIENTED_EDGE ( 'NONE', *, *, #19540, .T. ) ;
#36986=EDGE_CURVE ( 'NONE', #37443, #25256, #22341, .T. ) ;
#36988=ADVANCED_FACE ( 'NONE', ( #33593 ), #38215, .F. ) ;
#36996=LINE ( 'NONE', #26170, #31200 ) ;
#37001=CARTESIAN_POINT ( 'NONE',  ( 181.0000000000000000, 165.0000000000000000, -356.0000000000001705 ) ) ;
#37002=CIRCLE ( 'NONE', #14835, 3.749999999999975575 ) ;
#37013=CARTESIAN_POINT ( 'NONE',  ( 169.0000000000000000, -174.9999999999999716, -99.00000000000014211 ) ) ;
#37014=ORIENTED_EDGE ( 'NONE', *, *, #22515, .T. ) ;
#37017=DIRECTION ( 'NONE',  ( -1.000000000000000000, -0.000000000000000000, -0.000000000000000000 ) ) ;
#37019=DIRECTION ( 'NONE',  ( 0.000000000000000000, -2.537652627714643577E-15, -1.000000000000000000 ) ) ;
#37028=LINE ( 'NONE', #12627, #16386 ) ;
#37030=CARTESIAN_POINT ( 'NONE',  ( 168.9999999999999716, -252.4999999999999432, -349.9999999999999432 ) ) ;
#37034=CARTESIAN_POINT ( 'NONE',  ( 168.9999999999999716, 175.0000000000000284, -340.0000000000001137 ) ) ;
#37036=ORIENTED_EDGE ( 'NONE', *, *, #36630, .T. ) ;
#37039=LINE ( 'NONE', #25206, #46767 ) ;
#37040=CARTESIAN_POINT ( 'NONE',  ( 339.9999999999999432, 181.0000000000000284, -358.0000000000002274 ) ) ;
#37052=VERTEX_POINT ( 'NONE', #19847 ) ;
#37058=VERTEX_POINT ( 'NONE', #23712 ) ;
#37067=CIRCLE ( 'NONE', #15721, 4.000000000000003553 ) ;
#37072=ORIENTED_EDGE ( 'NONE', *, *, #32149, .T. ) ;
#37076=EDGE_CURVE ( 'NONE', #47178, #12553, #31683, .T. ) ;
#37091=ORIENTED_EDGE ( 'NONE', *, *, #8393, .F. ) ;
#37098=FACE_OUTER_BOUND ( 'NONE', #6140, .T. ) ;
#37106=CARTESIAN_POINT ( 'NONE',  ( 185.0000000000000000, -174.9999999999999716, -340.0000000000001137 ) ) ;
#37113=FACE_BOUND ( 'NONE', #43038, .T. ) ;
#37114=FACE_OUTER_BOUND ( 'NONE', #34596, .T. ) ;
#37116=EDGE_CURVE ( 'NONE', #37058, #14195, #27268, .T. ) ;
#37117=DIRECTION ( 'NONE',  ( -1.121065046350011585E-16, -0.7071067811865475727, -0.7071067811865474617 ) ) ;
#37127=CARTESIAN_POINT ( 'NONE',  ( 360.0000000000001137, 169.0000000000000000, 349.9999999999998295 ) ) ;
#37129=VERTEX_POINT ( 'NONE', #4719 ) ;
#37131=EDGE_CURVE ( 'NONE', #3587, #49828, #373, .T. ) ;
#37132=ADVANCED_FACE ( 'NONE', ( #31930 ), #20357, .F. ) ;
#37133=ORIENTED_EDGE ( 'NONE', *, *, #47160, .F. ) ;
#37135=AXIS2_PLACEMENT_3D ( 'NONE', #26367, #45818, #18901 ) ;
#37137=EDGE_CURVE ( 'NONE', #32721, #18711, #118, .T. ) ;
#37141=DIRECTION ( 'NONE',  ( 1.000000000000000000, 0.000000000000000000, 0.000000000000000000 ) ) ;
#37142=ORIENTED_EDGE ( 'NONE', *, *, #16208, .T. ) ;
#37147=CARTESIAN_POINT ( 'NONE',  ( 185.0000000000000000, 175.0000000000000284, -356.0000000000001705 ) ) ;
#37149=VERTEX_POINT ( 'NONE', #32672 ) ;
#37156=CARTESIAN_POINT ( 'NONE',  ( 0.000000000000000000, 185.0000000000000284, 343.9999999999997726 ) ) ;
#37157=DIRECTION ( 'NONE',  ( 1.333906992743555050E-23, -1.000000000000000000, 0.000000000000000000 ) ) ;
#37159=EDGE_CURVE ( 'NONE', #46544, #49245, #50157, .T. ) ;
#37161=EDGE_CURVE ( 'NONE', #1515, #17667, #36795, .T. ) ;
#37170=AXIS2_PLACEMENT_3D ( 'NONE', #14225, #41436, #14488 ) ;
#37177=CIRCLE ( 'NONE', #28943, 4.000000000000003553 ) ;
#37179=ORIENTED_EDGE ( 'NONE', *, *, #31142, .T. ) ;
#37183=LINE ( 'NONE', #44080, #26284 ) ;
#37187=DIRECTION ( 'NONE',  ( 0.000000000000000000, 0.000000000000000000, -1.000000000000000000 ) ) ;
#37189=ORIENTED_EDGE ( 'NONE', *, *, #31638, .F. ) ;
#37190=CARTESIAN_POINT ( 'NONE',  ( 0.000000000000000000, 169.0000000000000000, -358.0000000000002274 ) ) ;
#37191=LINE ( 'NONE', #2755, #48716 ) ;
#37193=CARTESIAN_POINT ( 'NONE',  ( 181.0000000000000284, -174.9999999999999716, -97.00000000000014211 ) ) ;
#37196=VERTEX_POINT ( 'NONE', #44936 ) ;
#37200=ORIENTED_EDGE ( 'NONE', *, *, #8618, .F. ) ;
#37205=CARTESIAN_POINT ( 'NONE',  ( 357.1715728752537302, 183.0000000000002558, -358.0000000000003979 ) ) ;
#37209=FACE_OUTER_BOUND ( 'NONE', #42287, .T. ) ;
#37210=EDGE_CURVE ( 'NONE', #30152, #16044, #44442, .T. ) ;
#37217=CYLINDRICAL_SURFACE ( 'NONE', #14483, 2.000000000000001776 ) ;
#37222=CARTESIAN_POINT ( 'NONE',  ( 339.9999999999999432, -182.9999999999999716, -344.0000000000001705 ) ) ;
#37228=CARTESIAN_POINT ( 'NONE',  ( 169.0000000000000000, -9.999999999999953815, -97.00000000000014211 ) ) ;
#37232=( BOUNDED_CURVE ( )  B_SPLINE_CURVE ( 3, ( #16657, #23603, #39525, #27712 ),
 .UNSPECIFIED., .F., .F. ) 
 B_SPLINE_CURVE_WITH_KNOTS ( ( 4, 4 ),
 ( 3.141592653589793116, 4.712388980384689674 ),
 .UNSPECIFIED. ) 
 CURVE ( )  GEOMETRIC_REPRESENTATION_ITEM ( )  RATIONAL_B_SPLINE_CURVE ( ( 1.000000000000000000, 0.8047378541243649375, 0.8047378541243649375, 1.000000000000000000 ) ) 
 REPRESENTATION_ITEM ( '' )  );
#37233=CARTESIAN_POINT ( 'NONE',  ( 181.0000000000000000, -272.4999999999999432, -355.9999999999999432 ) ) ;
#37240=VECTOR ( 'NONE', #10163, 1000.000000000000000 ) ;
#37243=VERTEX_POINT ( 'NONE', #37308 ) ;
#37252=ORIENTED_EDGE ( 'NONE', *, *, #31784, .F. ) ;
#37259=CARTESIAN_POINT ( 'NONE',  ( 360.0000000000001137, 169.0000000000000000, 343.9999999999998295 ) ) ;
#37266=ORIENTED_EDGE ( 'NONE', *, *, #4042, .F. ) ;
#37268=LINE ( 'NONE', #17738, #6849 ) ;
#37275=CARTESIAN_POINT ( 'NONE',  ( 357.9999999999999432, -177.9999999999999147, -353.0000000000001705 ) ) ;
#37284=CARTESIAN_POINT ( 'NONE',  ( 185.0000000000000000, -93.50000000000005684, -340.0000000000001137 ) ) ;
#37286=VECTOR ( 'NONE', #10055, 1000.000000000000000 ) ;
#37308=CARTESIAN_POINT ( 'NONE',  ( 339.9999999999998863, -166.9999999999999432, 343.9999999999997726 ) ) ;
#37309=ORIENTED_EDGE ( 'NONE', *, *, #31638, .T. ) ;
#37311=DIRECTION ( 'NONE',  ( -1.000000000000000000, 0.000000000000000000, 0.000000000000000000 ) ) ;
#37314=CARTESIAN_POINT ( 'NONE',  ( 339.9999999999998863, -180.9999999999999716, 343.9999999999997726 ) ) ;
#37316=VECTOR ( 'NONE', #6248, 1000.000000000000000 ) ;
#37317=DIRECTION ( 'NONE',  ( 1.000000000000000000, 0.000000000000000000, 0.000000000000000000 ) ) ;
#37322=VECTOR ( 'NONE', #22740, 1000.000000000000000 ) ;
#37330=ORIENTED_EDGE ( 'NONE', *, *, #18676, .T. ) ;
#37335=VECTOR ( 'NONE', #16092, 1000.000000000000000 ) ;
#37339=DIRECTION ( 'NONE',  ( 0.000000000000000000, -1.580451535867971417E-48, 1.000000000000000000 ) ) ;
#37342=VECTOR ( 'NONE', #6101, 1000.000000000000000 ) ;
#37348=CYLINDRICAL_SURFACE ( 'NONE', #30666, 3.749999999999975575 ) ;
#37355=CARTESIAN_POINT ( 'NONE',  ( 169.0000000000000284, 175.0000000000000284, 355.9999999999998863 ) ) ;
#37358=ORIENTED_EDGE ( 'NONE', *, *, #13591, .F. ) ;
#37364=CARTESIAN_POINT ( 'NONE',  ( 181.0000000000000000, -180.9999999999999716, -350.0000000000001705 ) ) ;
#37369=LINE ( 'NONE', #1939, #43296 ) ;
#37370=CARTESIAN_POINT ( 'NONE',  ( 358.3431457505075741, -185.0000000000001421, -360.0000000000003411 ) ) ;
#37371=EDGE_CURVE ( 'NONE', #27608, #43697, #30090, .T. ) ;
#37373=CARTESIAN_POINT ( 'NONE',  ( 166.9999999999999716, 175.0000000000000284, -356.0000000000001705 ) ) ;
#37381=VECTOR ( 'NONE', #46443, 1000.000000000000000 ) ;
#37384=AXIS2_PLACEMENT_3D ( 'NONE', #30580, #50013, #19006 ) ;
#37394=DIRECTION ( 'NONE',  ( -0.000000000000000000, -1.000000000000000000, 2.537652627714643577E-15 ) ) ;
#37408=ORIENTED_EDGE ( 'NONE', *, *, #32558, .F. ) ;
#37409=DIRECTION ( 'NONE',  ( 1.612977847700450206E-50, 0.000000000000000000, 1.000000000000000000 ) ) ;
#37414=VECTOR ( 'NONE', #17987, 1000.000000000000000 ) ;
#37416=AXIS2_PLACEMENT_3D ( 'NONE', #20730, #6088, #28683 ) ;
#37422=VECTOR ( 'NONE', #29538, 1000.000000000000000 ) ;
#37443=VERTEX_POINT ( 'NONE', #34705 ) ;
#37454=CARTESIAN_POINT ( 'NONE',  ( 0.000000000000000000, -168.9999999999999432, -344.0000000000001705 ) ) ;
#37458=DIRECTION ( 'NONE',  ( 0.000000000000000000, 0.000000000000000000, 1.000000000000000000 ) ) ;
#37461=CARTESIAN_POINT ( 'NONE',  ( -5.000000000000000000, 165.2000000000000171, -359.8000000000002387 ) ) ;
#37464=CYLINDRICAL_SURFACE ( 'NONE', #17942, 2.000000000000001776 ) ;
#37477=DIRECTION ( 'NONE',  ( -1.586032892321652236E-16, -1.000000000000000000, -6.853681917100419162E-49 ) ) ;
#37480=EDGE_CURVE ( 'NONE', #7928, #16503, #37177, .T. ) ;
#37485=FACE_OUTER_BOUND ( 'NONE', #43965, .T. ) ;
#37487=EDGE_CURVE ( 'NONE', #42500, #1045, #46113, .T. ) ;
#37491=ORIENTED_EDGE ( 'NONE', *, *, #34484, .T. ) ;
#37493=LINE ( 'NONE', #2306, #41097 ) ;
#37494=FACE_OUTER_BOUND ( 'NONE', #41259, .T. ) ;
#37497=DIRECTION ( 'NONE',  ( -1.000000000000000000, -0.000000000000000000, -0.000000000000000000 ) ) ;
#37500=ORIENTED_EDGE ( 'NONE', *, *, #6058, .T. ) ;
#37506=EDGE_CURVE ( 'NONE', #3572, #50585, #31418, .T. ) ;
#37525=CARTESIAN_POINT ( 'NONE',  ( 356.0000000000000568, 165.0000000000000000, -94.00000000000019895 ) ) ;
#37534=VERTEX_POINT ( 'NONE', #1563 ) ;
#37536=ORIENTED_EDGE ( 'NONE', *, *, #1733, .T. ) ;
#37542=VERTEX_POINT ( 'NONE', #24662 ) ;
#37547=EDGE_CURVE ( 'NONE', #17736, #26366, #22565, .T. ) ;
#37553=DIRECTION ( 'NONE',  ( 1.000000000000000000, 0.000000000000000000, -1.860490536778032451E-50 ) ) ;
#37559=CARTESIAN_POINT ( 'NONE',  ( 166.9999999999999716, -168.9999999999999432, -350.0000000000001705 ) ) ;
#37560=EDGE_LOOP ( 'NONE', ( #12507, #7967, #10174, #25949 ) ) ;
#37567=ORIENTED_EDGE ( 'NONE', *, *, #32201, .T. ) ;
#37568=ADVANCED_FACE ( 'NONE', ( #41311 ), #21054, .T. ) ;
#37580=EDGE_LOOP ( 'NONE', ( #25145, #31316, #16593, #27403, #38579, #50491, #24206, #50326 ) ) ;
#37581=DIRECTION ( 'NONE',  ( -1.000000000000000000, 0.000000000000000000, 0.000000000000000000 ) ) ;
#37588=CARTESIAN_POINT ( 'NONE',  ( 181.0000000000000000, -184.9999999999999716, -344.0000000000001137 ) ) ;
#37589=FACE_OUTER_BOUND ( 'NONE', #31894, .T. ) ;
#37596=ORIENTED_EDGE ( 'NONE', *, *, #31869, .F. ) ;
#37598=ORIENTED_EDGE ( 'NONE', *, *, #10583, .F. ) ;
#37602=EDGE_CURVE ( 'NONE', #49709, #21399, #20794, .T. ) ;
#37607=DIRECTION ( 'NONE',  ( 0.000000000000000000, 0.000000000000000000, 1.000000000000000000 ) ) ;
#37608=ADVANCED_FACE ( 'NONE', ( #49717 ), #41562, .F. ) ;
#37614=AXIS2_PLACEMENT_3D ( 'NONE', #28067, #40383, #24480 ) ;
#37618=DIRECTION ( 'NONE',  ( 0.000000000000000000, 2.969158215481698263E-48, -1.000000000000000000 ) ) ;
#37621=CLOSED_SHELL ( 'NONE', ( #50261, #41365, #33164, #10496, #9698, #17560, #1795, #47419 ) ) ;
#37632=ORIENTED_EDGE ( 'NONE', *, *, #17964, .F. ) ;
#37639=ORIENTED_EDGE ( 'NONE', *, *, #28836, .F. ) ;
#37641=EDGE_CURVE ( 'NONE', #35337, #20217, #3547, .T. ) ;
#37648=DIRECTION ( 'NONE',  ( 0.000000000000000000, 1.000000000000000000, 0.000000000000000000 ) ) ;
#37649=LINE ( 'NONE', #2477, #41842 ) ;
#37652=DIRECTION ( 'NONE',  ( 0.000000000000000000, 0.000000000000000000, -1.000000000000000000 ) ) ;
#37659=CIRCLE ( 'NONE', #38464, 2.000000000000001776 ) ;
#37674=CYLINDRICAL_SURFACE ( 'NONE', #12396, 2.000000000000001776 ) ;
#37675=AXIS2_PLACEMENT_3D ( 'NONE', #35103, #7381, #23008 ) ;
#37683=AXIS2_PLACEMENT_3D ( 'NONE', #8802, #47994, #28293 ) ;
#37689=CARTESIAN_POINT ( 'NONE',  ( -5.000000000000000000, -175.0000000000000284, -346.2500000000002274 ) ) ;
#37694=CARTESIAN_POINT ( 'NONE',  ( 168.9999999999999716, 175.0000000000000284, -360.0000000000001705 ) ) ;
#37698=DIRECTION ( 'NONE',  ( 0.000000000000000000, 0.000000000000000000, -1.000000000000000000 ) ) ;
#37699=EDGE_CURVE ( 'NONE', #6656, #26366, #15120, .T. ) ;
#37702=ORIENTED_EDGE ( 'NONE', *, *, #6207, .F. ) ;
#37706=ORIENTED_EDGE ( 'NONE', *, *, #39520, .T. ) ;
#37716=( BOUNDED_CURVE ( )  B_SPLINE_CURVE ( 3, ( #45335, #26112, #6877, #6118 ),
 .UNSPECIFIED., .F., .F. ) 
 B_SPLINE_CURVE_WITH_KNOTS ( ( 4, 4 ),
 ( 1.570796326794889675, 3.141592653589793116 ),
 .UNSPECIFIED. ) 
 CURVE ( )  GEOMETRIC_REPRESENTATION_ITEM ( )  RATIONAL_B_SPLINE_CURVE ( ( 1.000000000000000000, 0.8047378541243634942, 0.8047378541243634942, 1.000000000000000000 ) ) 
 REPRESENTATION_ITEM ( '' )  );
#37720=ORIENTED_EDGE ( 'NONE', *, *, #25238, .T. ) ;
#37732=DIRECTION ( 'NONE',  ( 0.000000000000000000, -2.265761274745217480E-16, 1.000000000000000000 ) ) ;
#37733=EDGE_LOOP ( 'NONE', ( #31962, #26812, #36772, #31977 ) ) ;
#37737=( BOUNDED_CURVE ( )  B_SPLINE_CURVE ( 3, ( #48751, #45163, #20840, #2106 ),
 .UNSPECIFIED., .F., .F. ) 
 B_SPLINE_CURVE_WITH_KNOTS ( ( 4, 4 ),
 ( 4.712388980384689674, 6.283185307179586232 ),
 .UNSPECIFIED. ) 
 CURVE ( )  GEOMETRIC_REPRESENTATION_ITEM ( )  RATIONAL_B_SPLINE_CURVE ( ( 1.000000000000000000, 0.8047378541243649375, 0.8047378541243649375, 1.000000000000000000 ) ) 
 REPRESENTATION_ITEM ( '' )  );
#37738=LINE ( 'NONE', #21556, #36004 ) ;
#37745=CARTESIAN_POINT ( 'NONE',  ( 181.0000000000000000, -184.9999999999999716, -356.0000000000001705 ) ) ;
#37746=EDGE_LOOP ( 'NONE', ( #19239, #36985, #5713, #8556 ) ) ;
#37751=ORIENTED_EDGE ( 'NONE', *, *, #28252, .F. ) ;
#37752=AXIS2_PLACEMENT_3D ( 'NONE', #33582, #14567, #45595 ) ;
#37754=AXIS2_PLACEMENT_3D ( 'NONE', #34650, #19222, #19480 ) ;
#37760=CARTESIAN_POINT ( 'NONE',  ( 167.0000000000000284, 165.0000000000000000, 343.9999999999998863 ) ) ;
#37762=VECTOR ( 'NONE', #24011, 1000.000000000000000 ) ;
#37763=EDGE_LOOP ( 'NONE', ( #17530, #6851, #4373, #12803 ) ) ;
#37770=ORIENTED_EDGE ( 'NONE', *, *, #28619, .T. ) ;
#37775=EDGE_CURVE ( 'NONE', #30452, #22310, #43578, .T. ) ;
#37777=ORIENTED_EDGE ( 'NONE', *, *, #24881, .F. ) ;
#37789=CIRCLE ( 'NONE', #35349, 2.000000000000001776 ) ;
#37795=EDGE_CURVE ( 'NONE', #45390, #48932, #12530, .T. ) ;
#37800=ORIENTED_EDGE ( 'NONE', *, *, #43107, .T. ) ;
#37802=ADVANCED_FACE ( 'NONE', ( #38996 ), #32052, .T. ) ;
#37805=PLANE ( 'NONE',  #25014 ) ;
#37811=VERTEX_POINT ( 'NONE', #15887 ) ;
#37816=ORIENTED_EDGE ( 'NONE', *, *, #13704, .T. ) ;
#37817=CARTESIAN_POINT ( 'NONE',  ( 4.999999999999999112, 175.0000000000000284, 353.7500000000001705 ) ) ;
#37819=CARTESIAN_POINT ( 'NONE',  ( 168.9999999999999716, -5.999999999999950262, 339.9999999999998295 ) ) ;
#37821=EDGE_CURVE ( 'NONE', #40366, #34859, #15384, .T. ) ;
#37826=DIRECTION ( 'NONE',  ( 0.000000000000000000, -1.000000000000000000, 0.000000000000000000 ) ) ;
#37830=EDGE_LOOP ( 'NONE', ( #46802, #8532, #22140, #25761, #30891, #15080, #25882, #31301 ) ) ;
#37832=LINE ( 'NONE', #2648, #2010 ) ;
#37847=CARTESIAN_POINT ( 'NONE',  ( 344.0000000000000568, 165.0000000000000000, -110.0000000000002132 ) ) ;
#37848=VERTEX_POINT ( 'NONE', #504 ) ;
#37852=LINE ( 'NONE', #26287, #48520 ) ;
#37853=ORIENTED_EDGE ( 'NONE', *, *, #43989, .T. ) ;
#37854=DIRECTION ( 'NONE',  ( -4.758098676964957447E-16, -1.000000000000000000, 7.143884938411937192E-48 ) ) ;
#37855=CARTESIAN_POINT ( 'NONE',  ( 168.9999999999999716, -256.4999999999999432, -339.9999999999998863 ) ) ;
#37858=EDGE_CURVE ( 'NONE', #16503, #17104, #16141, .T. ) ;
#37868=AXIS2_PLACEMENT_3D ( 'NONE', #1132, #1382, #627 ) ;
#37874=FACE_OUTER_BOUND ( 'NONE', #36537, .T. ) ;
#37878=DIRECTION ( 'NONE',  ( 0.000000000000000000, -1.000000000000000000, 0.000000000000000000 ) ) ;
#37886=EDGE_CURVE ( 'NONE', #15688, #48233, #6544, .T. ) ;
#37887=EDGE_LOOP ( 'NONE', ( #34160, #36696, #42326, #1166 ) ) ;
#37888=CARTESIAN_POINT ( 'NONE',  ( 168.9999999999999716, -272.5000000000000000, -114.9999999999999005 ) ) ;
#37892=VECTOR ( 'NONE', #41793, 1000.000000000000000 ) ;
#37900=EDGE_CURVE ( 'NONE', #46025, #26544, #1692, .T. ) ;
#37902=ORIENTED_EDGE ( 'NONE', *, *, #18925, .T. ) ;
#37904=VECTOR ( 'NONE', #44847, 1000.000000000000000 ) ;
#37912=VERTEX_POINT ( 'NONE', #33260 ) ;
#37915=CARTESIAN_POINT ( 'NONE',  ( 339.9999999999998863, -185.0000000000001421, -349.9999999999998863 ) ) ;
#37917=CARTESIAN_POINT ( 'NONE',  ( 340.0000000000000568, 181.0000000000000284, 339.9999999999997726 ) ) ;
#37923=DIRECTION ( 'NONE',  ( 0.000000000000000000, -0.000000000000000000, -1.000000000000000000 ) ) ;
#37926=VECTOR ( 'NONE', #39313, 1000.000000000000000 ) ;
#37928=DIRECTION ( 'NONE',  ( 0.000000000000000000, 0.000000000000000000, 1.000000000000000000 ) ) ;
#37929=AXIS2_PLACEMENT_3D ( 'NONE', #40055, #301, #4880 ) ;
#37934=ORIENTED_EDGE ( 'NONE', *, *, #7078, .T. ) ;
#37936=AXIS2_PLACEMENT_3D ( 'NONE', #6377, #42032, #37458 ) ;
#37939=DIRECTION ( 'NONE',  ( -0.000000000000000000, 0.000000000000000000, 1.000000000000000000 ) ) ;
#37941=DIRECTION ( 'NONE',  ( 0.000000000000000000, 0.000000000000000000, -1.000000000000000000 ) ) ;
#37947=CARTESIAN_POINT ( 'NONE',  ( 181.0000000000000568, -164.9999999999999432, 339.9999999999997726 ) ) ;
#37950=CARTESIAN_POINT ( 'NONE',  ( 168.9999999999999716, -5.999999999999950262, -350.0000000000001705 ) ) ;
#37951=CARTESIAN_POINT ( 'NONE',  ( 355.9999999999999432, -185.0000000000001421, -360.0000000000003411 ) ) ;
#37952=CARTESIAN_POINT ( 'NONE',  ( 357.9999999999999432, 181.0000000000002558, -356.0000000000003411 ) ) ;
#37957=CYLINDRICAL_SURFACE ( 'NONE', #1256, 2.000000000000001776 ) ;
#37962=FACE_OUTER_BOUND ( 'NONE', #20823, .T. ) ;
#37964=AXIS2_PLACEMENT_3D ( 'NONE', #41014, #33327, #17159 ) ;
#37968=CARTESIAN_POINT ( 'NONE',  ( 344.0000000000000000, 165.0000000000000000, -106.0000000000001990 ) ) ;
#37971=ORIENTED_EDGE ( 'NONE', *, *, #4534, .F. ) ;
#37974=DIRECTION ( 'NONE',  ( 0.000000000000000000, 0.000000000000000000, 1.000000000000000000 ) ) ;
#37977=AXIS2_PLACEMENT_3D ( 'NONE', #30272, #18197, #38246 ) ;
#37983=CARTESIAN_POINT ( 'NONE',  ( 181.0000000000000000, -272.5000000000000000, -114.9999999999999147 ) ) ;
#37987=CARTESIAN_POINT ( 'NONE',  ( 339.9999999999998863, -180.9999999999999716, 343.9999999999997726 ) ) ;
#37992=ADVANCED_FACE ( 'NONE', ( #37113, #13732 ), #29387, .F. ) ;
#37999=VECTOR ( 'NONE', #33500, 1000.000000000000000 ) ;
#38003=ORIENTED_EDGE ( 'NONE', *, *, #43450, .F. ) ;
#38016=VECTOR ( 'NONE', #48009, 1000.000000000000000 ) ;
#38019=DIRECTION ( 'NONE',  ( -1.586032892321652236E-16, -1.000000000000000000, -6.853681917100419162E-49 ) ) ;
#38022=EDGE_CURVE ( 'NONE', #42571, #43608, #10136, .T. ) ;
#38029=VECTOR ( 'NONE', #1779, 1000.000000000000000 ) ;
#38030=VERTEX_POINT ( 'NONE', #42946 ) ;
#38032=ORIENTED_EDGE ( 'NONE', *, *, #36278, .F. ) ;
#38035=( BOUNDED_CURVE ( )  B_SPLINE_CURVE ( 3, ( #48628, #28925, #21471, #16620 ),
 .UNSPECIFIED., .F., .F. ) 
 B_SPLINE_CURVE_WITH_KNOTS ( ( 4, 4 ),
 ( 4.712388980384689674, 6.283185307179586232 ),
 .UNSPECIFIED. ) 
 CURVE ( )  GEOMETRIC_REPRESENTATION_ITEM ( )  RATIONAL_B_SPLINE_CURVE ( ( 1.000000000000000000, 0.8047378541243649375, 0.8047378541243649375, 1.000000000000000000 ) ) 
 REPRESENTATION_ITEM ( '' )  );
#38036=CARTESIAN_POINT ( 'NONE',  ( 181.0000000000000000, -174.9999999999999716, -340.0000000000001137 ) ) ;
#38049=LINE ( 'NONE', #6985, #47076 ) ;
#38050=ADVANCED_FACE ( 'NONE', ( #38114 ), #42439, .F. ) ;
#38055=VERTEX_POINT ( 'NONE', #46760 ) ;
#38059=DIRECTION ( 'NONE',  ( 1.000000000000000000, -1.586032997072805650E-16, -4.759647537211363479E-16 ) ) ;
#38060=LINE ( 'NONE', #21377, #22251 ) ;
#38066=LINE ( 'NONE', #41897, #49880 ) ;
#38067=CARTESIAN_POINT ( 'NONE',  ( 0.000000000000000000, 167.0000000000000000, 343.9999999999997726 ) ) ;
#38068=AXIS2_PLACEMENT_3D ( 'NONE', #18530, #45958, #3648 ) ;
#38071=DIRECTION ( 'NONE',  ( 1.000000000000000000, 0.000000000000000000, 0.000000000000000000 ) ) ;
#38075=VERTEX_POINT ( 'NONE', #34258 ) ;
#38079=DIRECTION ( 'NONE',  ( 0.000000000000000000, -2.537652627714643577E-15, -1.000000000000000000 ) ) ;
#38085=EDGE_CURVE ( 'NONE', #43697, #20947, #3440, .T. ) ;
#38087=LINE ( 'NONE', #19064, #10761 ) ;
#38092=DIRECTION ( 'NONE',  ( 0.000000000000000000, -1.000000000000000000, -1.544785076050074834E-48 ) ) ;
#38093=CYLINDRICAL_SURFACE ( 'NONE', #1961, 2.000000000000001776 ) ;
#38105=ORIENTED_EDGE ( 'NONE', *, *, #11103, .F. ) ;
#38111=AXIS2_PLACEMENT_3D ( 'NONE', #24085, #20223, #724 ) ;
#38113=EDGE_CURVE ( 'NONE', #13420, #23604, #7300, .T. ) ;
#38114=FACE_OUTER_BOUND ( 'NONE', #33248, .T. ) ;
#38118=PLANE ( 'NONE',  #6563 ) ;
#38121=VERTEX_POINT ( 'NONE', #5222 ) ;
#38124=PLANE ( 'NONE',  #26 ) ;
#38125=MANIFOLD_SOLID_BREP ( 'Square tube 20 X 20 X 2(1)[5]', #6458 ) ;
#38131=VERTEX_POINT ( 'NONE', #20872 ) ;
#38138=VERTEX_POINT ( 'NONE', #43958 ) ;
#38139=EDGE_CURVE ( 'NONE', #16044, #24255, #32678, .T. ) ;
#38143=VECTOR ( 'NONE', #27668, 1000.000000000000000 ) ;
#38149=DIRECTION ( 'NONE',  ( 1.000000000000000000, -4.996003610813203446E-16, 1.033975765691284410E-24 ) ) ;
#38152=VERTEX_POINT ( 'NONE', #44449 ) ;
#38156=ORIENTED_EDGE ( 'NONE', *, *, #13992, .T. ) ;
#38157=ORIENTED_EDGE ( 'NONE', *, *, #20109, .F. ) ;
#38158=FACE_OUTER_BOUND ( 'NONE', #23952, .T. ) ;
#38162=ORIENTED_EDGE ( 'NONE', *, *, #15905, .T. ) ;
#38168=CARTESIAN_POINT ( 'NONE',  ( 339.9999999999998863, -168.9999999999999432, 357.9999999999997726 ) ) ;
#38173=DIRECTION ( 'NONE',  ( 1.000000000000000000, 0.000000000000000000, 0.000000000000000000 ) ) ;
#38176=CIRCLE ( 'NONE', #22579, 3.749999999999975575 ) ;
#38182=ADVANCED_FACE ( 'NONE', ( #24734 ), #40388, .F. ) ;
#38184=ORIENTED_EDGE ( 'NONE', *, *, #38427, .T. ) ;
#38190=CIRCLE ( 'NONE', #497, 4.000000000000003553 ) ;
#38198=CARTESIAN_POINT ( 'NONE',  ( 165.0000000000000000, -5.999999999999950262, 339.9999999999998863 ) ) ;
#38206=CIRCLE ( 'NONE', #21812, 3.749999999999975575 ) ;
#38207=ORIENTED_EDGE ( 'NONE', *, *, #1064, .T. ) ;
#38213=CARTESIAN_POINT ( 'NONE',  ( 167.0000000000000284, 175.0000000000000284, 343.9999999999998863 ) ) ;
#38215=CYLINDRICAL_SURFACE ( 'NONE', #28108, 2.000000000000001776 ) ;
#38219=AXIS2_PLACEMENT_3D ( 'NONE', #25829, #1969, #41974 ) ;
#38228=DIRECTION ( 'NONE',  ( 0.000000000000000000, 2.537652627714642000E-15, 1.000000000000000000 ) ) ;
#38230=ADVANCED_FACE ( 'NONE', ( #21625 ), #17281, .T. ) ;
#38235=LINE ( 'NONE', #38485, #25822 ) ;
#38239=DIRECTION ( 'NONE',  ( 1.000000000000000000, 0.000000000000000000, 0.000000000000000000 ) ) ;
#38241=ADVANCED_FACE ( 'NONE', ( #25994 ), #22136, .T. ) ;
#38244=LINE ( 'NONE', #30028, #30628 ) ;
#38246=DIRECTION ( 'NONE',  ( 0.000000000000000000, 1.000000000000000000, 0.000000000000000000 ) ) ;
#38249=CYLINDRICAL_SURFACE ( 'NONE', #36013, 2.000000000000001776 ) ;
#38250=EDGE_CURVE ( 'NONE', #21405, #34922, #32138, .T. ) ;
#38255=VECTOR ( 'NONE', #24397, 1000.000000000000000 ) ;
#38261=ADVANCED_FACE ( 'NONE', ( #33200, #29083 ), #13675, .T. ) ;
#38268=CARTESIAN_POINT ( 'NONE',  ( 339.9999999999999432, -168.9999999999999432, -342.0000000000001705 ) ) ;
#38271=CARTESIAN_POINT ( 'NONE',  ( 341.9999999999999432, -165.0000000000001137, -106.0000000000001990 ) ) ;
#38281=AXIS2_PLACEMENT_3D ( 'NONE', #22729, #17864, #15036 ) ;
#38286=LINE ( 'NONE', #2342, #17985 ) ;
#38290=ADVANCED_FACE ( 'NONE', ( #41125 ), #13910, .F. ) ;
#38297=DIRECTION ( 'NONE',  ( 0.000000000000000000, 5.664403186863042467E-17, 1.000000000000000000 ) ) ;
#38299=ORIENTED_EDGE ( 'NONE', *, *, #49062, .F. ) ;
#38303=DIRECTION ( 'NONE',  ( -1.000000000000000000, 0.000000000000000000, -7.793956916774525800E-48 ) ) ;
#38306=MANIFOLD_SOLID_BREP ( 'Cut-Extrude1[1]', #37621 ) ;
#38308=CARTESIAN_POINT ( 'NONE',  ( 342.0000000000000568, 172.0000000000000000, 346.9999999999998295 ) ) ;
#38314=ORIENTED_EDGE ( 'NONE', *, *, #23710, .T. ) ;
#38327=DIRECTION ( 'NONE',  ( -1.000000000000000000, 0.000000000000000000, 0.000000000000000000 ) ) ;
#38328=( BOUNDED_CURVE ( )  B_SPLINE_CURVE ( 3, ( #12323, #50516, #7483, #43123 ),
 .UNSPECIFIED., .F., .F. ) 
 B_SPLINE_CURVE_WITH_KNOTS ( ( 4, 4 ),
 ( 4.712388980384703885, 6.283185307179586232 ),
 .UNSPECIFIED. ) 
 CURVE ( )  GEOMETRIC_REPRESENTATION_ITEM ( )  RATIONAL_B_SPLINE_CURVE ( ( 1.000000000000000000, 0.8047378541243683792, 0.8047378541243683792, 1.000000000000000000 ) ) 
 REPRESENTATION_ITEM ( '' )  );
#38334=EDGE_LOOP ( 'NONE', ( #40454, #9493, #34848, #20216, #40476, #10875, #7049, #33807 ) ) ;
#38348=CARTESIAN_POINT ( 'NONE',  ( 340.0000000000000568, 181.0000000000000284, 355.9999999999998295 ) ) ;
#38353=CARTESIAN_POINT ( 'NONE',  ( 0.000000000000000000, 184.8000000000000114, 340.1999999999997044 ) ) ;
#38360=VERTEX_POINT ( 'NONE', #23404 ) ;
#38362=VECTOR ( 'NONE', #38864, 1000.000000000000000 ) ;
#38368=DIRECTION ( 'NONE',  ( 1.612977847700450206E-50, 0.000000000000000000, 1.000000000000000000 ) ) ;
#38372=ADVANCED_FACE ( 'NONE', ( #26489 ), #3376, .T. ) ;
#38377=MANIFOLD_SOLID_BREP ( 'Square tube 20 X 20 X 2(1)[9]', #38423 ) ;
#38379=FACE_OUTER_BOUND ( 'NONE', #30117, .T. ) ;
#38397=FACE_OUTER_BOUND ( 'NONE', #26896, .T. ) ;
#38404=DIRECTION ( 'NONE',  ( -1.000000000000000000, 0.000000000000000000, 1.860490536778032451E-50 ) ) ;
#38407=FACE_OUTER_BOUND ( 'NONE', #45047, .T. ) ;
#38415=DIRECTION ( 'NONE',  ( -1.000000000000000000, 0.000000000000000000, -1.612977847700450206E-50 ) ) ;
#38419=EDGE_LOOP ( 'NONE', ( #46030, #44909, #19465, #36587 ) ) ;
#38423=CLOSED_SHELL ( 'NONE', ( #8303, #37132, #29173, #3640, #47079, #18589, #50232, #14929, #13775, #38182, #42200, #40626, #33303, #36650, #6958, #18909, #33339, #17155 ) ) ;
#38427=EDGE_CURVE ( 'NONE', #29740, #13231, #39830, .T. ) ;
#38428=CARTESIAN_POINT ( 'NONE',  ( 342.8284271247461561, -167.0000000000001137, 341.9999999999999432 ) ) ;
#38436=FACE_OUTER_BOUND ( 'NONE', #9202, .T. ) ;
#38444=ORIENTED_EDGE ( 'NONE', *, *, #25960, .T. ) ;
#38446=ORIENTED_EDGE ( 'NONE', *, *, #16569, .T. ) ;
#38447=ADVANCED_FACE ( 'NONE', ( #15959 ), #8520, .T. ) ;
#38448=DIRECTION ( 'NONE',  ( -1.612977847700450206E-50, 0.000000000000000000, -1.000000000000000000 ) ) ;
#38450=AXIS2_PLACEMENT_3D ( 'NONE', #23587, #31558, #47143 ) ;
#38459=CIRCLE ( 'NONE', #30233, 4.000000000000003553 ) ;
#38464=AXIS2_PLACEMENT_3D ( 'NONE', #30228, #11249, #46089 ) ;
#38468=DIRECTION ( 'NONE',  ( -0.000000000000000000, -3.186989995019654210E-49, -1.000000000000000000 ) ) ;
#38470=ORIENTED_EDGE ( 'NONE', *, *, #46575, .F. ) ;
#38472=ORIENTED_EDGE ( 'NONE', *, *, #677, .T. ) ;
#38485=CARTESIAN_POINT ( 'NONE',  ( 181.0000000000000284, 2.775557561562891351E-14, -115.0000000000001563 ) ) ;
#38490=VERTEX_POINT ( 'NONE', #21313 ) ;
#38492=CARTESIAN_POINT ( 'NONE',  ( 166.9999999999999716, -81.49999999999997158, -350.0000000000001705 ) ) ;
#38497=VECTOR ( 'NONE', #38404, 1000.000000000000000 ) ;
#38499=CIRCLE ( 'NONE', #49044, 2.000000000000001776 ) ;
#38507=CARTESIAN_POINT ( 'NONE',  ( 168.9999999999998579, -272.5000000000000000, -112.9999999999999005 ) ) ;
#38508=ORIENTED_EDGE ( 'NONE', *, *, #28385, .F. ) ;
#38515=PLANE ( 'NONE',  #41264 ) ;
#38520=ORIENTED_EDGE ( 'NONE', *, *, #46363, .F. ) ;
#38522=FACE_OUTER_BOUND ( 'NONE', #8252, .T. ) ;
#38525=CIRCLE ( 'NONE', #33606, 4.000000000000003553 ) ;
#38526=EDGE_CURVE ( 'NONE', #19896, #24656, #44138, .T. ) ;
#38542=EDGE_CURVE ( 'NONE', #38121, #28737, #9510, .T. ) ;
#38547=CARTESIAN_POINT ( 'NONE',  ( 339.9999999999999432, 183.0000000000000284, -344.0000000000001705 ) ) ;
#38551=ORIENTED_EDGE ( 'NONE', *, *, #34914, .T. ) ;
#38554=DIRECTION ( 'NONE',  ( -1.000000000000000000, 0.000000000000000000, 0.000000000000000000 ) ) ;
#38558=ORIENTED_EDGE ( 'NONE', *, *, #19874, .F. ) ;
#38571=CARTESIAN_POINT ( 'NONE',  ( 339.9999999999997726, -183.3431457505076878, 358.3431457505077447 ) ) ;
#38573=AXIS2_PLACEMENT_3D ( 'NONE', #40812, #37497, #44881 ) ;
#38575=ORIENTED_EDGE ( 'NONE', *, *, #5062, .F. ) ;
#38577=FACE_OUTER_BOUND ( 'NONE', #19795, .T. ) ;
#38578=DIRECTION ( 'NONE',  ( -1.000000000000000000, 0.000000000000000000, 0.000000000000000000 ) ) ;
#38579=ORIENTED_EDGE ( 'NONE', *, *, #11580, .F. ) ;
#38585=LINE ( 'NONE', #3660, #26745 ) ;
#38586=CARTESIAN_POINT ( 'NONE',  ( 165.0000000000000284, 165.0000000000000000, 355.9999999999998863 ) ) ;
#38591=VERTEX_POINT ( 'NONE', #1575 ) ;
#38593=EDGE_LOOP ( 'NONE', ( #44410, #16234, #45209, #12811 ) ) ;
#38597=EDGE_CURVE ( 'NONE', #20258, #17953, #10432, .T. ) ;
#38600=VERTEX_POINT ( 'NONE', #25678 ) ;
#38606=ORIENTED_EDGE ( 'NONE', *, *, #33733, .T. ) ;
#38608=AXIS2_PLACEMENT_3D ( 'NONE', #50359, #3962, #46765 ) ;
#38610=DIRECTION ( 'NONE',  ( 0.000000000000000000, 0.000000000000000000, -1.000000000000000000 ) ) ;
#38613=DIRECTION ( 'NONE',  ( 0.000000000000000000, -0.000000000000000000, 1.000000000000000000 ) ) ;
#38625=CARTESIAN_POINT ( 'NONE',  ( 185.0000000000000000, -164.9999999999999432, 355.9999999999998863 ) ) ;
#38628=EDGE_CURVE ( 'NONE', #38600, #44276, #22571, .T. ) ;
#38630=ORIENTED_EDGE ( 'NONE', *, *, #40096, .T. ) ;
#38633=CARTESIAN_POINT ( 'NONE',  ( 344.0000000000000000, -167.0000000000000853, -342.0000000000002842 ) ) ;
#38636=VECTOR ( 'NONE', #22264, 1000.000000000000000 ) ;
#38640=ORIENTED_EDGE ( 'NONE', *, *, #43441, .T. ) ;
#38653=ORIENTED_EDGE ( 'NONE', *, *, #9079, .T. ) ;
#38660=ORIENTED_EDGE ( 'NONE', *, *, #8649, .T. ) ;
#38664=CARTESIAN_POINT ( 'NONE',  ( 360.0000000000001137, 181.0000000000000284, 355.9999999999998295 ) ) ;
#38665=VECTOR ( 'NONE', #33938, 1000.000000000000000 ) ;
#38671=DIRECTION ( 'NONE',  ( -3.364279341222519273E-16, 0.7071067811865474617, -0.7071067811865476838 ) ) ;
#38672=CIRCLE ( 'NONE', #7537, 2.000000000000001776 ) ;
#38673=DIRECTION ( 'NONE',  ( 1.000000000000000000, 0.000000000000000000, 0.000000000000000000 ) ) ;
#38676=DIRECTION ( 'NONE',  ( -3.172065784643302499E-16, -1.000000000000000000, 2.537652627714642000E-15 ) ) ;
#38686=CARTESIAN_POINT ( 'NONE',  ( 181.0000000000000000, -256.4999999999999432, -339.9999999999998863 ) ) ;
#38689=DIRECTION ( 'NONE',  ( 0.000000000000000000, 0.000000000000000000, 1.000000000000000000 ) ) ;
#38691=VECTOR ( 'NONE', #36727, 1000.000000000000000 ) ;
#38695=ORIENTED_EDGE ( 'NONE', *, *, #36352, .T. ) ;
#38696=DIRECTION ( 'NONE',  ( 0.000000000000000000, 0.000000000000000000, 1.000000000000000000 ) ) ;
#38698=CYLINDRICAL_SURFACE ( 'NONE', #45855, 2.000000000000001776 ) ;
#38700=UNCERTAINTY_MEASURE_WITH_UNIT (LENGTH_MEASURE( 1.000000000000000082E-05 ), #20976, 'distance_accuracy_value', 'NONE');
#38701=LINE ( 'NONE', #4488, #34353 ) ;
#38705=DIRECTION ( 'NONE',  ( -1.000000000000000000, 0.000000000000000000, 0.000000000000000000 ) ) ;
#38709=VERTEX_POINT ( 'NONE', #40013 ) ;
#38717=CIRCLE ( 'NONE', #5108, 3.749999999999975575 ) ;
#38719=ORIENTED_EDGE ( 'NONE', *, *, #35253, .T. ) ;
#38722=LINE ( 'NONE', #49704, #17239 ) ;
#38728=CARTESIAN_POINT ( 'NONE',  ( 185.0000000000000568, 165.0000000000000000, 343.9999999999998863 ) ) ;
#38734=PLANE ( 'NONE',  #7883 ) ;
#38737=CARTESIAN_POINT ( 'NONE',  ( 356.0000000000000000, 174.9999999999996589, -344.0000000000002842 ) ) ;
#38741=DIRECTION ( 'NONE',  ( -1.000000000000000000, 0.000000000000000000, 0.000000000000000000 ) ) ;
#38744=EDGE_CURVE ( 'NONE', #25569, #35217, #23970, .T. ) ;
#38746=ADVANCED_BREP_SHAPE_REPRESENTATION ( '', ( #22493, #39637, #39816, #5102, #38125, #22914, #39303, #39060, #38377, #4445, #21989, #21395, #39561, #22072, #21149, #21477, #5021, #22244, #38306, #4281, #21652, #5610, #45486 ), #41416 ) ;
#38756=AXIS2_PLACEMENT_3D ( 'NONE', #2103, #5937, #21586 ) ;
#38761=ORIENTED_EDGE ( 'NONE', *, *, #48777, .T. ) ;
#38768=CARTESIAN_POINT ( 'NONE',  ( 167.0000000000000284, 165.0000000000000000, 355.9999999999998863 ) ) ;
#38773=FACE_OUTER_BOUND ( 'NONE', #901, .T. ) ;
#38776=CARTESIAN_POINT ( 'NONE',  ( 181.0000000000000568, 165.0000000000000000, 355.9999999999998863 ) ) ;
#38778=ORIENTED_EDGE ( 'NONE', *, *, #15788, .T. ) ;
#38779=CYLINDRICAL_SURFACE ( 'NONE', #30312, 4.000000000000003553 ) ;
#38785=DIRECTION ( 'NONE',  ( -3.172065784643302499E-16, -1.000000000000000000, 2.537652627714642000E-15 ) ) ;
#38791=( NAMED_UNIT ( * ) SI_UNIT ( $, .STERADIAN. ) SOLID_ANGLE_UNIT ( ) );
#38792=EDGE_CURVE ( 'NONE', #11587, #23937, #4831, .T. ) ;
#38797=CARTESIAN_POINT ( 'NONE',  ( 164.9999999999999716, -174.9999999999999716, -340.0000000000001137 ) ) ;
#38798=FACE_OUTER_BOUND ( 'NONE', #11259, .T. ) ;
#38800=AXIS2_PLACEMENT_3D ( 'NONE', #30157, #13990, #37878 ) ;
#38812=( NAMED_UNIT ( * ) PLANE_ANGLE_UNIT ( ) SI_UNIT ( $, .RADIAN. ) );
#38816=CARTESIAN_POINT ( 'NONE',  ( 169.0000000000000000, -168.9999999999999432, -115.0000000000001847 ) ) ;
#38825=AXIS2_PLACEMENT_3D ( 'NONE', #13208, #9618, #16564 ) ;
#38828=EDGE_LOOP ( 'NONE', ( #3282, #17100, #28704, #29707 ) ) ;
#38840=VERTEX_POINT ( 'NONE', #5084 ) ;
#38842=CARTESIAN_POINT ( 'NONE',  ( 0.000000000000000000, 184.8000000000000114, -359.8000000000002387 ) ) ;
#38847=VECTOR ( 'NONE', #3308, 1000.000000000000000 ) ;
#38848=ORIENTED_EDGE ( 'NONE', *, *, #45832, .T. ) ;
#38849=FACE_OUTER_BOUND ( 'NONE', #37746, .T. ) ;
#38850=CARTESIAN_POINT ( 'NONE',  ( 0.000000000000000000, 183.0000000000000284, 343.9999999999997726 ) ) ;
#38855=EDGE_LOOP ( 'NONE', ( #17916, #22340 ) ) ;
#38864=DIRECTION ( 'NONE',  ( -0.000000000000000000, -1.000000000000000000, -0.000000000000000000 ) ) ;
#38866=DIRECTION ( 'NONE',  ( 1.000000000000000000, 0.000000000000000000, 0.000000000000000000 ) ) ;
#38870=VERTEX_POINT ( 'NONE', #36424 ) ;
#38875=DIRECTION ( 'NONE',  ( 0.000000000000000000, 0.000000000000000000, 1.000000000000000000 ) ) ;
#38881=CYLINDRICAL_SURFACE ( 'NONE', #36860, 4.000000000000003553 ) ;
#38886=ADVANCED_FACE ( 'NONE', ( #28950 ), #16911, .T. ) ;
#38888=ORIENTED_EDGE ( 'NONE', *, *, #23459, .F. ) ;
#38904=VECTOR ( 'NONE', #2800, 1000.000000000000000 ) ;
#38910=CARTESIAN_POINT ( 'NONE',  ( 356.0000000000006253, 167.0000000000000000, 341.9999999999998863 ) ) ;
#38911=DIRECTION ( 'NONE',  ( -1.000000000000000000, 0.000000000000000000, 0.000000000000000000 ) ) ;
#38918=UNCERTAINTY_MEASURE_WITH_UNIT (LENGTH_MEASURE( 1.000000000000000082E-05 ), #13172, 'distance_accuracy_value', 'NONE');
#38919=ORIENTED_EDGE ( 'NONE', *, *, #18111, .F. ) ;
#38929=LINE ( 'NONE', #4010, #17114 ) ;
#38932=CARTESIAN_POINT ( 'NONE',  ( 168.9999999999999716, -174.9999999999999716, -340.0000000000001137 ) ) ;
#38937=VECTOR ( 'NONE', #14503, 1000.000000000000000 ) ;
#38944=DIRECTION ( 'NONE',  ( -1.000000000000000000, 0.000000000000000000, 0.000000000000000000 ) ) ;
#38947=DIRECTION ( 'NONE',  ( 0.000000000000000000, -1.000000000000000000, -3.186989995019654210E-49 ) ) ;
#38950=DIRECTION ( 'NONE',  ( 0.000000000000000000, 1.000000000000000000, 0.000000000000000000 ) ) ;
#38953=( NAMED_UNIT ( * ) SI_UNIT ( $, .STERADIAN. ) SOLID_ANGLE_UNIT ( ) );
#38954=ORIENTED_EDGE ( 'NONE', *, *, #36410, .F. ) ;
#38958=EDGE_LOOP ( 'NONE', ( #28270, #26733, #13428, #45833, #7926, #18234, #8130, #34219 ) ) ;
#38959=DIRECTION ( 'NONE',  ( 1.000000000000000000, 0.000000000000000000, 0.000000000000000000 ) ) ;
#38960=CARTESIAN_POINT ( 'NONE',  ( 340.0000000000000568, 181.0000000000000284, 355.9999999999997726 ) ) ;
#38964=CARTESIAN_POINT ( 'NONE',  ( 355.9999999999999432, -185.0000000000001421, -360.0000000000003411 ) ) ;
#38965=VECTOR ( 'NONE', #899, 1000.000000000000000 ) ;
#38970=EDGE_LOOP ( 'NONE', ( #2175, #15083, #20461, #45721 ) ) ;
#38972=EDGE_LOOP ( 'NONE', ( #34647, #151, #5391, #22739, #1612, #30492, #27412, #31310 ) ) ;
#38973=VERTEX_POINT ( 'NONE', #11228 ) ;
#38982=CARTESIAN_POINT ( 'NONE',  ( 339.9999999999999432, -169.0000000000001137, -344.0000000000002842 ) ) ;
#38991=AXIS2_PLACEMENT_3D ( 'NONE', #45748, #33499, #1937 ) ;
#38996=FACE_OUTER_BOUND ( 'NONE', #39137, .T. ) ;
#38998=PLANE ( 'NONE',  #2396 ) ;
#39000=CARTESIAN_POINT ( 'NONE',  ( 342.8284271247462129, 182.9999999999999716, 357.9999999999996589 ) ) ;
#39003=VECTOR ( 'NONE', #15915, 1000.000000000000000 ) ;
#39005=ORIENTED_EDGE ( 'NONE', *, *, #49902, .F. ) ;
#39007=CARTESIAN_POINT ( 'NONE',  ( 350.0000000000000000, -180.9999999999999716, -360.0000000000002274 ) ) ;
#39008=AXIS2_PLACEMENT_3D ( 'NONE', #23176, #26275, #10864 ) ;
#39010=CARTESIAN_POINT ( 'NONE',  ( 185.0000000000000284, 6.000000000000060396, 339.9999999999998863 ) ) ;
#39011=ADVANCED_FACE ( 'NONE', ( #46338 ), #10460, .T. ) ;
#39014=CARTESIAN_POINT ( 'NONE',  ( 168.9999999999999716, -270.5000000000000000, -114.9999999999999147 ) ) ;
#39032=CARTESIAN_POINT ( 'NONE',  ( 0.000000000000000000, 183.0000000000000284, -356.0000000000002274 ) ) ;
#39036=DIRECTION ( 'NONE',  ( 1.000000000000000000, 0.000000000000000000, 0.000000000000000000 ) ) ;
#39040=DIRECTION ( 'NONE',  ( 1.000000000000000000, 0.000000000000000000, 0.000000000000000000 ) ) ;
#39045=AXIS2_PLACEMENT_3D ( 'NONE', #39655, #32466, #47303 ) ;
#39048=ORIENTED_EDGE ( 'NONE', *, *, #427, .F. ) ;
#39052=EDGE_CURVE ( 'NONE', #27797, #44740, #27383, .T. ) ;
#39060=MANIFOLD_SOLID_BREP ( 'Square tube 20 X 20 X 2(1)[8]', #20377 ) ;
#39067=ADVANCED_FACE ( 'NONE', ( #47595 ), #28140, .F. ) ;
#39068=EDGE_CURVE ( 'NONE', #18793, #4444, #35608, .T. ) ;
#39071=ORIENTED_EDGE ( 'NONE', *, *, #3763, .T. ) ;
#39072=EDGE_CURVE ( 'NONE', #18367, #27545, #20183, .T. ) ;
#39076=CARTESIAN_POINT ( 'NONE',  ( 339.9999999999999432, 166.6568542494925396, -341.6568542494925396 ) ) ;
#39078=ORIENTED_EDGE ( 'NONE', *, *, #48550, .F. ) ;
#39082=DIRECTION ( 'NONE',  ( -1.000000000000000000, 0.000000000000000000, 0.000000000000000000 ) ) ;
#39086=DIRECTION ( 'NONE',  ( 1.000000000000000000, -0.000000000000000000, 0.000000000000000000 ) ) ;
#39089=CARTESIAN_POINT ( 'NONE',  ( 339.9999999999999432, -168.9999999999999432, -360.0000000000002274 ) ) ;
#39097=ORIENTED_EDGE ( 'NONE', *, *, #8064, .F. ) ;
#39101=EDGE_LOOP ( 'NONE', ( #17883, #49078, #13494, #7931 ) ) ;
#39107=ADVANCED_FACE ( 'NONE', ( #43013 ), #35362, .F. ) ;
#39109=VERTEX_POINT ( 'NONE', #47083 ) ;
#39110=ORIENTED_EDGE ( 'NONE', *, *, #44744, .F. ) ;
#39112=DIRECTION ( 'NONE',  ( 0.000000000000000000, 5.664403186863042467E-17, 1.000000000000000000 ) ) ;
#39118=ORIENTED_EDGE ( 'NONE', *, *, #17243, .T. ) ;
#39120=DIRECTION ( 'NONE',  ( 0.000000000000000000, -1.000000000000000000, 0.000000000000000000 ) ) ;
#39127=DIRECTION ( 'NONE',  ( -1.000000000000000000, 0.000000000000000000, -1.612977847700450206E-50 ) ) ;
#39137=EDGE_LOOP ( 'NONE', ( #49010, #45156, #19799, #9927 ) ) ;
#39138=FACE_OUTER_BOUND ( 'NONE', #38828, .T. ) ;
#39139=CARTESIAN_POINT ( 'NONE',  ( 339.9999999999999432, -185.0000000000001421, -356.0000000000002274 ) ) ;
#39141=DIRECTION ( 'NONE',  ( 1.000000000000000000, 0.000000000000000000, 0.000000000000000000 ) ) ;
#39156=VERTEX_POINT ( 'NONE', #36628 ) ;
#39159=LINE ( 'NONE', #30956, #2938 ) ;
#39161=ADVANCED_FACE ( 'NONE', ( #16844, #21689 ), #44772, .T. ) ;
#39168=ORIENTED_EDGE ( 'NONE', *, *, #32557, .F. ) ;
#39170=CARTESIAN_POINT ( 'NONE',  ( 181.0000000000000284, -9.999999999999953815, -111.0000000000001563 ) ) ;
#39171=DIRECTION ( 'NONE',  ( 1.000000000000000000, 0.000000000000000000, 0.000000000000000000 ) ) ;
#39185=DIRECTION ( 'NONE',  ( 0.000000000000000000, -2.537652627714643577E-15, -1.000000000000000000 ) ) ;
#39190=AXIS2_PLACEMENT_3D ( 'NONE', #46324, #23777, #50666 ) ;
#39197=DIRECTION ( 'NONE',  ( 0.000000000000000000, 1.000000000000000000, 0.000000000000000000 ) ) ;
#39205=EDGE_LOOP ( 'NONE', ( #25765, #10155, #4515, #38954, #11370, #36075, #49428, #42061 ) ) ;
#39208=ADVANCED_FACE ( 'NONE', ( #37874 ), #49354, .F. ) ;
#39215=DIRECTION ( 'NONE',  ( -0.000000000000000000, -1.000000000000000000, -0.000000000000000000 ) ) ;
#39216=CARTESIAN_POINT ( 'NONE',  ( 165.0000000000000000, -174.9999999999999716, -99.00000000000014211 ) ) ;
#39221=CARTESIAN_POINT ( 'NONE',  ( 168.9999999999999716, 165.0000000000000000, -356.0000000000001705 ) ) ;
#39223=ORIENTED_EDGE ( 'NONE', *, *, #41507, .F. ) ;
#39228=LINE ( 'NONE', #23567, #28316 ) ;
#39244=FACE_OUTER_BOUND ( 'NONE', #4007, .T. ) ;
#39247=ORIENTED_EDGE ( 'NONE', *, *, #4528, .F. ) ;
#39250=CARTESIAN_POINT ( 'NONE',  ( 342.0000000000000568, 182.1715728752537871, 357.1715728752535597 ) ) ;
#39256=ORIENTED_EDGE ( 'NONE', *, *, #24576, .F. ) ;
#39257=LINE ( 'NONE', #42327, #21286 ) ;
#39261=CARTESIAN_POINT ( 'NONE',  ( 164.9999999999999716, -180.9999999999999716, -350.0000000000001705 ) ) ;
#39262=DIRECTION ( 'NONE',  ( 0.000000000000000000, 0.000000000000000000, -1.000000000000000000 ) ) ;
#39276=DIRECTION ( 'NONE',  ( -1.000000000000000000, 0.000000000000000000, 0.000000000000000000 ) ) ;
#39277=CARTESIAN_POINT ( 'NONE',  ( 169.0000000000000284, 175.0000000000000284, 339.9999999999998863 ) ) ;
#39281=ORIENTED_EDGE ( 'NONE', *, *, #19553, .T. ) ;
#39282=FACE_OUTER_BOUND ( 'NONE', #40661, .T. ) ;
#39285=FACE_OUTER_BOUND ( 'NONE', #21398, .T. ) ;
#39286=AXIS2_PLACEMENT_3D ( 'NONE', #40445, #5282, #39443 ) ;
#39290=AXIS2_PLACEMENT_3D ( 'NONE', #38816, #3645, #19291 ) ;
#39294=DIRECTION ( 'NONE',  ( 1.000000000000000000, 0.000000000000000000, 1.586032872232979935E-16 ) ) ;
#39297=ORIENTED_EDGE ( 'NONE', *, *, #39671, .T. ) ;
#39303=MANIFOLD_SOLID_BREP ( 'Square tube 20 X 20 X 2(1)[7]', #34309 ) ;
#39307=CARTESIAN_POINT ( 'NONE',  ( -5.000000000000000000, -175.0000000000000284, 353.7500000000001705 ) ) ;
#39309=EDGE_CURVE ( 'NONE', #48553, #49726, #14198, .T. ) ;
#39313=DIRECTION ( 'NONE',  ( 1.333906992743555050E-23, -1.000000000000000000, 0.000000000000000000 ) ) ;
#39327=VECTOR ( 'NONE', #17654, 1000.000000000000000 ) ;
#39329=ADVANCED_FACE ( 'NONE', ( #35480 ), #28525, .T. ) ;
#39333=ORIENTED_EDGE ( 'NONE', *, *, #37159, .T. ) ;
#39335=DIRECTION ( 'NONE',  ( 1.586032880504786307E-16, -1.654361225106055350E-24, 1.000000000000000000 ) ) ;
#39336=DIRECTION ( 'NONE',  ( 0.000000000000000000, -1.000000000000000000, -3.186989995019654210E-49 ) ) ;
#39338=AXIS2_PLACEMENT_3D ( 'NONE', #15928, #47431, #35189 ) ;
#39344=VERTEX_POINT ( 'NONE', #20311 ) ;
#39346=PLANE ( 'NONE',  #30026 ) ;
#39347=DIRECTION ( 'NONE',  ( 1.110223024625156171E-16, -0.7071067811865474617, 0.7071067811865474617 ) ) ;
#39349=CARTESIAN_POINT ( 'NONE',  ( 360.0000000000000000, 175.0000000000000284, -106.0000000000001990 ) ) ;
#39351=LINE ( 'NONE', #10863, #33727 ) ;
#39353=LINE ( 'NONE', #43932, #40690 ) ;
#39358=VERTEX_POINT ( 'NONE', #328 ) ;
#39360=CARTESIAN_POINT ( 'NONE',  ( 181.0000000000000000, 165.0000000000000000, -340.0000000000001705 ) ) ;
#39375=VECTOR ( 'NONE', #29585, 1000.000000000000000 ) ;
#39379=ORIENTED_EDGE ( 'NONE', *, *, #47745, .T. ) ;
#39381=CARTESIAN_POINT ( 'NONE',  ( 0.000000000000000000, 167.0000000000000000, -344.0000000000001705 ) ) ;
#39384=MECHANICAL_DESIGN_GEOMETRIC_PRESENTATION_REPRESENTATION('',(#2467),#28698);
#39387=VECTOR ( 'NONE', #13805, 1000.000000000000000 ) ;
#39388=EDGE_CURVE ( 'NONE', #37149, #13307, #20930, .T. ) ;
#39390=ORIENTED_EDGE ( 'NONE', *, *, #17073, .F. ) ;
#39391=CARTESIAN_POINT ( 'NONE',  ( 357.9999999999999432, -165.0000000000001137, -106.0000000000001990 ) ) ;
#39394=ORIENTED_EDGE ( 'NONE', *, *, #37900, .F. ) ;
#39397=CARTESIAN_POINT ( 'NONE',  ( 168.9999999999999716, 175.0000000000000284, -356.0000000000001705 ) ) ;
#39399=EDGE_CURVE ( 'NONE', #7818, #34262, #23911, .T. ) ;
#39400=PLANE ( 'NONE',  #6171 ) ;
#39408=ORIENTED_EDGE ( 'NONE', *, *, #4201, .T. ) ;
#39416=CIRCLE ( 'NONE', #70, 2.000000000000001776 ) ;
#39418=ORIENTED_EDGE ( 'NONE', *, *, #33616, .T. ) ;
#39421=PLANE ( 'NONE',  #18375 ) ;
#39424=VERTEX_POINT ( 'NONE', #6425 ) ;
#39434=DIRECTION ( 'NONE',  ( -1.587271980518778491E-16, 5.169878828456422968E-26, 1.000000000000000000 ) ) ;
#39443=DIRECTION ( 'NONE',  ( 1.000000000000000000, 0.000000000000000000, 0.000000000000000000 ) ) ;
#39451=CARTESIAN_POINT ( 'NONE',  ( 340.0000000000000568, 169.0000000000000000, 355.9999999999997726 ) ) ;
#39457=ORIENTED_EDGE ( 'NONE', *, *, #18103, .F. ) ;
#39463=DIRECTION ( 'NONE',  ( -1.000000000000000000, 0.000000000000000000, -2.958228394578794270E-31 ) ) ;
#39471=ORIENTED_EDGE ( 'NONE', *, *, #36410, .T. ) ;
#39472=VECTOR ( 'NONE', #30507, 1000.000000000000000 ) ;
#39478=LINE ( 'NONE', #15858, #49836 ) ;
#39481=ORIENTED_EDGE ( 'NONE', *, *, #48034, .T. ) ;
#39482=ORIENTED_EDGE ( 'NONE', *, *, #50701, .T. ) ;
#39484=CARTESIAN_POINT ( 'NONE',  ( 168.9999999999999716, -184.9999999999999716, -344.0000000000001137 ) ) ;
#39485=AXIS2_PLACEMENT_3D ( 'NONE', #4906, #1076, #827 ) ;
#39492=FACE_OUTER_BOUND ( 'NONE', #31371, .T. ) ;
#39497=CARTESIAN_POINT ( 'NONE',  ( 358.0000000000001137, 169.0000000000000000, 349.9999999999998863 ) ) ;
#39499=CARTESIAN_POINT ( 'NONE',  ( 167.0000000000000284, 165.0000000000000000, 355.9999999999998863 ) ) ;
#39500=CARTESIAN_POINT ( 'NONE',  ( 0.000000000000000000, 165.0000000000000000, -356.0000000000002274 ) ) ;
#39512=AXIS2_PLACEMENT_3D ( 'NONE', #40380, #8575, #12656 ) ;
#39517=ORIENTED_EDGE ( 'NONE', *, *, #20547, .F. ) ;
#39520=EDGE_CURVE ( 'NONE', #5419, #31711, #41829, .T. ) ;
#39524=CARTESIAN_POINT ( 'NONE',  ( 164.9999999999999716, -184.9999999999999716, -344.0000000000006253 ) ) ;
#39525=CARTESIAN_POINT ( 'NONE',  ( 339.9999999999999432, -166.6568542494925396, -341.6568542494925396 ) ) ;
#39528=LINE ( 'NONE', #773, #39003 ) ;
#39539=VERTEX_POINT ( 'NONE', #23341 ) ;
#39540=PLANE ( 'NONE',  #39338 ) ;
#39544=STYLED_ITEM('',(#50747),#38125);
#39546=FACE_OUTER_BOUND ( 'NONE', #15250, .T. ) ;
#39547=DIRECTION ( 'NONE',  ( -0.000000000000000000, -1.000000000000000000, -0.000000000000000000 ) ) ;
#39549=AXIS2_PLACEMENT_3D ( 'NONE', #32081, #46918, #35439 ) ;
#39551=DIRECTION ( 'NONE',  ( 0.000000000000000000, 0.000000000000000000, 1.000000000000000000 ) ) ;
#39555=EDGE_CURVE ( 'NONE', #47169, #35315, #19959, .T. ) ;
#39558=DIRECTION ( 'NONE',  ( -0.000000000000000000, -1.000000000000000000, -0.000000000000000000 ) ) ;
#39559=DIRECTION ( 'NONE',  ( -1.586032892321652236E-16, -1.000000000000000000, -6.853681917100419162E-49 ) ) ;
#39561=MANIFOLD_SOLID_BREP ( 'Square tube 20 X 20 X 2(1)[13]', #43305 ) ;
#39565=VECTOR ( 'NONE', #39347, 1000.000000000000114 ) ;
#39568=VERTEX_POINT ( 'NONE', #39014 ) ;
#39571=CARTESIAN_POINT ( 'NONE',  ( 339.9999999999999432, 169.0000000000001705, -344.0000000000002842 ) ) ;
#39579=ORIENTED_EDGE ( 'NONE', *, *, #24604, .F. ) ;
#39583=CARTESIAN_POINT ( 'NONE',  ( 165.0000000000000000, 2.775557561562891351E-14, -99.00000000000014211 ) ) ;
#39585=FACE_OUTER_BOUND ( 'NONE', #24766, .T. ) ;
#39586=PLANE ( 'NONE',  #12586 ) ;
#39596=ORIENTED_EDGE ( 'NONE', *, *, #45325, .T. ) ;
#39598=ORIENTED_EDGE ( 'NONE', *, *, #37821, .T. ) ;
#39600=EDGE_CURVE ( 'NONE', #11492, #20673, #22582, .T. ) ;
#39602=LINE ( 'NONE', #3931, #17329 ) ;
#39603=ORIENTED_EDGE ( 'NONE', *, *, #24576, .T. ) ;
#39605=AXIS2_PLACEMENT_3D ( 'NONE', #1013, #29216, #40018 ) ;
#39606=EDGE_LOOP ( 'NONE', ( #46539, #33467, #17863, #26706 ) ) ;
#39607=CARTESIAN_POINT ( 'NONE',  ( 183.0000000000000000, -93.49999999999998579, -350.0000000000001705 ) ) ;
#39609=VECTOR ( 'NONE', #29383, 1000.000000000000000 ) ;
#39610=DIRECTION ( 'NONE',  ( -0.000000000000000000, -1.000000000000000000, -0.000000000000000000 ) ) ;
#39616=ORIENTED_EDGE ( 'NONE', *, *, #13352, .T. ) ;
#39620=VECTOR ( 'NONE', #8449, 1000.000000000000000 ) ;
#39622=DIRECTION ( 'NONE',  ( -1.586032892321652482E-16, 0.000000000000000000, -1.000000000000000000 ) ) ;
#39623=ORIENTED_EDGE ( 'NONE', *, *, #1325, .T. ) ;
#39629=CARTESIAN_POINT ( 'NONE',  ( 344.0000000000000000, -165.0000000000001137, -94.00000000000019895 ) ) ;
#39636=DIRECTION ( 'NONE',  ( 1.000000000000000000, -1.586032892321652236E-16, -1.586032892321651989E-16 ) ) ;
#39637=MANIFOLD_SOLID_BREP ( 'Square tube 20 X 20 X 2(1)[2]', #8090 ) ;
#39640=FACE_OUTER_BOUND ( 'NONE', #41940, .T. ) ;
#39641=EDGE_CURVE ( 'NONE', #12244, #17553, #1273, .T. ) ;
#39642=ORIENTED_EDGE ( 'NONE', *, *, #37210, .T. ) ;
#39644=CARTESIAN_POINT ( 'NONE',  ( 169.0000000000000000, -174.9999999999999716, -97.00000000000014211 ) ) ;
#39655=CARTESIAN_POINT ( 'NONE',  ( 344.0000000000000000, -174.9999999999999716, 343.9999999999998295 ) ) ;
#39666=CARTESIAN_POINT ( 'NONE',  ( 350.0000000000000000, 181.0000000000000284, -356.0000000000002274 ) ) ;
#39671=EDGE_CURVE ( 'NONE', #5729, #37149, #8214, .T. ) ;
#39675=CARTESIAN_POINT ( 'NONE',  ( 183.0000000000000284, -174.9999999999999716, -99.00000000000014211 ) ) ;
#39681=EDGE_CURVE ( 'NONE', #47520, #8172, #16651, .T. ) ;
#39682=VECTOR ( 'NONE', #50503, 1000.000000000000000 ) ;
#39684=ORIENTED_EDGE ( 'NONE', *, *, #42110, .T. ) ;
#39685=EDGE_CURVE ( 'NONE', #10108, #45431, #7962, .T. ) ;
#39688=ADVANCED_FACE ( 'NONE', ( #19748 ), #47912, .F. ) ;
#39692=MECHANICAL_DESIGN_GEOMETRIC_PRESENTATION_REPRESENTATION('',(#23252),#4438);
#39693=FACE_OUTER_BOUND ( 'NONE', #5376, .T. ) ;
#39706=PLANE ( 'NONE',  #48557 ) ;
#39710=ORIENTED_EDGE ( 'NONE', *, *, #40387, .F. ) ;
#39712=FACE_OUTER_BOUND ( 'NONE', #5348, .T. ) ;
#39719=AXIS2_PLACEMENT_3D ( 'NONE', #10466, #26106, #37941 ) ;
#39723=VECTOR ( 'NONE', #23507, 1000.000000000000000 ) ;
#39726=CARTESIAN_POINT ( 'NONE',  ( 169.0000000000000000, -9.999999999999953815, -111.0000000000001563 ) ) ;
#39729=DIRECTION ( 'NONE',  ( 0.000000000000000000, -1.000000000000000000, 0.000000000000000000 ) ) ;
#39734=CARTESIAN_POINT ( 'NONE',  ( 168.9999999999999716, 6.000000000000060396, 339.9999999999998295 ) ) ;
#39742=CARTESIAN_POINT ( 'NONE',  ( 168.9999999999999716, -174.9999999999999716, -342.0000000000001137 ) ) ;
#39749=FACE_OUTER_BOUND ( 'NONE', #22039, .T. ) ;
#39756=LINE ( 'NONE', #20241, #17160 ) ;
#39773=VERTEX_POINT ( 'NONE', #6113 ) ;
#39779=CARTESIAN_POINT ( 'NONE',  ( 0.000000000000000000, -168.9999999999999432, -356.0000000000002274 ) ) ;
#39781=VECTOR ( 'NONE', #10822, 1000.000000000000000 ) ;
#39784=ADVANCED_FACE ( 'NONE', ( #17411 ), #14053, .T. ) ;
#39786=MECHANICAL_DESIGN_GEOMETRIC_PRESENTATION_REPRESENTATION('',(#11089),#8648);
#39787=ORIENTED_EDGE ( 'NONE', *, *, #44291, .F. ) ;
#39794=PLANE ( 'NONE',  #31698 ) ;
#39796=CIRCLE ( 'NONE', #20918, 4.000000000000003553 ) ;
#39797=LINE ( 'NONE', #291, #50443 ) ;
#39799=DIRECTION ( 'NONE',  ( -2.958228394578793832E-31, 0.000000000000000000, -1.000000000000000000 ) ) ;
#39807=ORIENTED_EDGE ( 'NONE', *, *, #50014, .T. ) ;
#39809=EDGE_CURVE ( 'NONE', #11132, #15809, #21014, .T. ) ;
#39816=MANIFOLD_SOLID_BREP ( 'Square tube 20 X 20 X 2(1)[3]', #15476 ) ;
#39817=PLANE ( 'NONE',  #33891 ) ;
#39819=CARTESIAN_POINT ( 'NONE',  ( 169.0000000000000000, -174.9999999999999716, -99.00000000000014211 ) ) ;
#39820=EDGE_LOOP ( 'NONE', ( #46656, #14721, #8381, #45398 ) ) ;
#39821=EDGE_CURVE ( 'NONE', #37052, #42864, #15079, .T. ) ;
#39825=LINE ( 'NONE', #8258, #37926 ) ;
#39829=ORIENTED_EDGE ( 'NONE', *, *, #45852, .F. ) ;
#39830=LINE ( 'NONE', #23654, #42807 ) ;
#39833=AXIS2_PLACEMENT_3D ( 'NONE', #9796, #45173, #10061 ) ;
#39834=ORIENTED_EDGE ( 'NONE', *, *, #21458, .F. ) ;
#39836=CARTESIAN_POINT ( 'NONE',  ( 339.9999999999999432, -168.9999999999999432, -358.0000000000002274 ) ) ;
#39840=AXIS2_PLACEMENT_3D ( 'NONE', #40437, #44007, #48077 ) ;
#39841=VERTEX_POINT ( 'NONE', #22271 ) ;
#39853=FACE_OUTER_BOUND ( 'NONE', #4344, .T. ) ;
#39857=VECTOR ( 'NONE', #10794, 1000.000000000000000 ) ;
#39858=CARTESIAN_POINT ( 'NONE',  ( 0.000000000000000000, -180.9999999999999716, -342.0000000000001705 ) ) ;
#39869=ORIENTED_EDGE ( 'NONE', *, *, #3918, .F. ) ;
#39871=DIRECTION ( 'NONE',  ( 0.000000000000000000, 2.537652627714643577E-15, 1.000000000000000000 ) ) ;
#39875=VERTEX_POINT ( 'NONE', #45827 ) ;
#39877=DIRECTION ( 'NONE',  ( 0.000000000000000000, 2.969158215481698263E-48, -1.000000000000000000 ) ) ;
#39882=DIRECTION ( 'NONE',  ( 1.000000000000000000, 0.000000000000000000, 0.000000000000000000 ) ) ;
#39884=DIRECTION ( 'NONE',  ( -0.000000000000000000, -1.000000000000000000, -0.000000000000000000 ) ) ;
#39889=PLANE ( 'NONE',  #37868 ) ;
#39892=CARTESIAN_POINT ( 'NONE',  ( 185.0000000000000000, 175.0000000000000284, -356.0000000000001705 ) ) ;
#39894=( GEOMETRIC_REPRESENTATION_CONTEXT ( 3 ) GLOBAL_UNCERTAINTY_ASSIGNED_CONTEXT ( ( #24594 ) ) GLOBAL_UNIT_ASSIGNED_CONTEXT ( ( #8368, #4508, #32481 ) ) REPRESENTATION_CONTEXT ( 'NONE', 'WORKASPACE' ) );
#39895=FACE_OUTER_BOUND ( 'NONE', #10452, .T. ) ;
#39898=DIRECTION ( 'NONE',  ( 0.000000000000000000, 1.000000000000000000, 0.000000000000000000 ) ) ;
#39902=CARTESIAN_POINT ( 'NONE',  ( 357.1715728752541850, 167.0000000000003411, -342.0000000000004547 ) ) ;
#39903=LINE ( 'NONE', #12182, #34869 ) ;
#39910=ORIENTED_EDGE ( 'NONE', *, *, #38526, .F. ) ;
#39919=VERTEX_POINT ( 'NONE', #34854 ) ;
#39945=DIRECTION ( 'NONE',  ( -1.586032892321652236E-16, -1.000000000000000000, -2.288264760618012091E-48 ) ) ;
#39951=ORIENTED_EDGE ( 'NONE', *, *, #48069, .F. ) ;
#39957=CARTESIAN_POINT ( 'NONE',  ( 350.0000000000000000, 167.0000000000000000, -344.0000000000001705 ) ) ;
#39982=LINE ( 'NONE', #35132, #26121 ) ;
#39983=ORIENTED_EDGE ( 'NONE', *, *, #8649, .F. ) ;
#39988=CARTESIAN_POINT ( 'NONE',  ( 349.9999999999999432, -168.9999999999999432, 343.9999999999997726 ) ) ;
#39989=ORIENTED_EDGE ( 'NONE', *, *, #34064, .T. ) ;
#39992=CARTESIAN_POINT ( 'NONE',  ( 0.000000000000000000, 165.2000000000000171, 359.7999999999997840 ) ) ;
#39994=EDGE_CURVE ( 'NONE', #29467, #41788, #20431, .T. ) ;
#39997=ADVANCED_FACE ( 'NONE', ( #958 ), #35369, .F. ) ;
#40004=DIRECTION ( 'NONE',  ( -4.758098676964957447E-16, -1.000000000000000000, 7.143884938411937192E-48 ) ) ;
#40011=EDGE_CURVE ( 'NONE', #18038, #34447, #31761, .T. ) ;
#40013=CARTESIAN_POINT ( 'NONE',  ( 185.0000000000000000, -268.5000000000000000, -339.9999999999998863 ) ) ;
#40014=CARTESIAN_POINT ( 'NONE',  ( 164.9999999999999716, -256.4999999999999432, -339.9999999999998863 ) ) ;
#40018=DIRECTION ( 'NONE',  ( 1.000000000000000000, 0.000000000000000000, 0.000000000000000000 ) ) ;
#40021=ORIENTED_EDGE ( 'NONE', *, *, #26632, .F. ) ;
#40023=ADVANCED_FACE ( 'NONE', ( #32756 ), #36886, .T. ) ;
#40024=ADVANCED_FACE ( 'NONE', ( #16856 ), #6049, .F. ) ;
#40025=CIRCLE ( 'NONE', #40816, 2.000000000000001776 ) ;
#40029=VERTEX_POINT ( 'NONE', #20695 ) ;
#40035=DIRECTION ( 'NONE',  ( 0.000000000000000000, -1.000000000000000000, 0.000000000000000000 ) ) ;
#40042=ORIENTED_EDGE ( 'NONE', *, *, #34666, .F. ) ;
#40047=LINE ( 'NONE', #20023, #9541 ) ;
#40055=CARTESIAN_POINT ( 'NONE',  ( -5.000000000000000000, 165.2000000000000171, 359.7999999999997840 ) ) ;
#40056=ORIENTED_EDGE ( 'NONE', *, *, #36574, .T. ) ;
#40057=ORIENTED_EDGE ( 'NONE', *, *, #4201, .F. ) ;
#40074=DIRECTION ( 'NONE',  ( 1.000000000000000000, 0.000000000000000000, 0.000000000000000000 ) ) ;
#40075=ORIENTED_EDGE ( 'NONE', *, *, #30391, .F. ) ;
#40081=ADVANCED_FACE ( 'NONE', ( #29400 ), #25303, .T. ) ;
#40095=VECTOR ( 'NONE', #5534, 1000.000000000000000 ) ;
#40096=EDGE_CURVE ( 'NONE', #6290, #26029, #50700, .T. ) ;
#40101=CARTESIAN_POINT ( 'NONE',  ( 350.0000000000001137, 169.0000000000000000, 357.9999999999997726 ) ) ;
#40104=VECTOR ( 'NONE', #16518, 1000.000000000000000 ) ;
#40109=AXIS2_PLACEMENT_3D ( 'NONE', #46460, #11351, #32125 ) ;
#40112=ORIENTED_EDGE ( 'NONE', *, *, #44350, .F. ) ;
#40127=PLANE ( 'NONE',  #39512 ) ;
#40130=CARTESIAN_POINT ( 'NONE',  ( 339.9999999999999432, 183.0000000000000284, -356.0000000000002274 ) ) ;
#40131=AXIS2_PLACEMENT_3D ( 'NONE', #33403, #48732, #13118 ) ;
#40134=VECTOR ( 'NONE', #16906, 1000.000000000000000 ) ;
#40137=DIRECTION ( 'NONE',  ( -1.586032892321652236E-16, -1.000000000000000000, -2.288264760618012091E-48 ) ) ;
#40150=ADVANCED_FACE ( 'NONE', ( #31458 ), #27347, .F. ) ;
#40155=ORIENTED_EDGE ( 'NONE', *, *, #42103, .F. ) ;
#40160=VECTOR ( 'NONE', #34591, 1000.000000000000000 ) ;
#40162=AXIS2_PLACEMENT_3D ( 'NONE', #39583, #39086, #3905 ) ;
#40164=DIRECTION ( 'NONE',  ( 1.333906992743555050E-23, -1.000000000000000000, 0.000000000000000000 ) ) ;
#40165=EDGE_LOOP ( 'NONE', ( #13576, #26318, #24512, #36342 ) ) ;
#40170=FACE_OUTER_BOUND ( 'NONE', #29492, .T. ) ;
#40178=FACE_OUTER_BOUND ( 'NONE', #5623, .T. ) ;
#40179=FACE_OUTER_BOUND ( 'NONE', #12427, .T. ) ;
#40182=CARTESIAN_POINT ( 'NONE',  ( -5.000000000000000000, -184.7999999999999545, 340.1999999999997044 ) ) ;
#40193=VECTOR ( 'NONE', #40323, 1000.000000000000000 ) ;
#40195=VERTEX_POINT ( 'NONE', #7343 ) ;
#40198=AXIS2_PLACEMENT_3D ( 'NONE', #39666, #43747, #24014 ) ;
#40204=ORIENTED_EDGE ( 'NONE', *, *, #36880, .F. ) ;
#40210=ORIENTED_EDGE ( 'NONE', *, *, #135, .F. ) ;
#40223=ORIENTED_EDGE ( 'NONE', *, *, #36494, .T. ) ;
#40228=EDGE_CURVE ( 'NONE', #29772, #37058, #7863, .T. ) ;
#40231=FACE_OUTER_BOUND ( 'NONE', #9699, .T. ) ;
#40237=LINE ( 'NONE', #8933, #16719 ) ;
#40238=CYLINDRICAL_SURFACE ( 'NONE', #37416, 2.000000000000001776 ) ;
#40257=ORIENTED_EDGE ( 'NONE', *, *, #4619, .F. ) ;
#40263=DIRECTION ( 'NONE',  ( -1.000000000000000000, 4.996003610813203446E-16, 1.586032878436834529E-16 ) ) ;
#40265=ORIENTED_EDGE ( 'NONE', *, *, #32471, .T. ) ;
#40269=ADVANCED_FACE ( 'NONE', ( #13882 ), #39421, .F. ) ;
#40274=CARTESIAN_POINT ( 'NONE',  ( 181.0000000000000284, -174.9999999999999716, -115.0000000000001563 ) ) ;
#40277=CARTESIAN_POINT ( 'NONE',  ( 350.0000000000001137, 167.0000000000000000, 355.9999999999997726 ) ) ;
#40279=CIRCLE ( 'NONE', #25544, 3.749999999999975575 ) ;
#40283=DIRECTION ( 'NONE',  ( 2.958228394578794708E-31, 0.000000000000000000, -1.000000000000000000 ) ) ;
#40285=DIRECTION ( 'NONE',  ( -0.000000000000000000, -0.000000000000000000, 1.000000000000000000 ) ) ;
#40286=CARTESIAN_POINT ( 'NONE',  ( 357.1715728752537871, -167.0000000000001137, -342.0000000000002842 ) ) ;
#40296=DIRECTION ( 'NONE',  ( -1.000000000000000000, 0.000000000000000000, 1.860490536778032451E-50 ) ) ;
#40299=EDGE_CURVE ( 'NONE', #3248, #5747, #47027, .T. ) ;
#40301=ADVANCED_FACE ( 'NONE', ( #12888 ), #20844, .F. ) ;
#40306=ADVANCED_FACE ( 'NONE', ( #9789 ), #32401, .T. ) ;
#40308=VECTOR ( 'NONE', #1879, 1000.000000000000000 ) ;
#40315=CARTESIAN_POINT ( 'NONE',  ( 350.0000000000000000, 165.0000000000000000, -344.0000000000001705 ) ) ;
#40322=EDGE_LOOP ( 'NONE', ( #23705, #11937, #2460, #44436 ) ) ;
#40323=DIRECTION ( 'NONE',  ( -1.000000000000000000, 0.000000000000000000, -7.793956916774525800E-48 ) ) ;
#40324=CARTESIAN_POINT ( 'NONE',  ( 168.9999999999999716, -254.5000000000000000, -114.9999999999999574 ) ) ;
#40338=ORIENTED_EDGE ( 'NONE', *, *, #18322, .T. ) ;
#40344=CIRCLE ( 'NONE', #41134, 2.000000000000001776 ) ;
#40349=CARTESIAN_POINT ( 'NONE',  ( 355.9999999999999432, -185.0000000000001421, 360.0000000000000000 ) ) ;
#40350=ADVANCED_FACE ( 'NONE', ( #28804, #44668 ), #21345, .T. ) ;
#40363=DIRECTION ( 'NONE',  ( -3.172065784643302499E-16, -1.000000000000000000, 2.537652627714642000E-15 ) ) ;
#40366=VERTEX_POINT ( 'NONE', #26721 ) ;
#40368=ORIENTED_EDGE ( 'NONE', *, *, #29300, .T. ) ;
#40372=PLANE ( 'NONE',  #47927 ) ;
#40377=AXIS2_PLACEMENT_3D ( 'NONE', #36143, #44060, #4810 ) ;
#40380=CARTESIAN_POINT ( 'NONE',  ( 183.0000000000000284, -174.9999999999999716, -111.0000000000001563 ) ) ;
#40383=DIRECTION ( 'NONE',  ( 1.000000000000000000, -4.758098676964957447E-16, 2.958228394578795584E-31 ) ) ;
#40384=DIRECTION ( 'NONE',  ( 0.000000000000000000, 1.000000000000000000, 1.544785076050074834E-48 ) ) ;
#40387=EDGE_CURVE ( 'NONE', #4113, #42347, #49254, .T. ) ;
#40388=PLANE ( 'NONE',  #45316 ) ;
#40413=VERTEX_POINT ( 'NONE', #14405 ) ;
#40423=CARTESIAN_POINT ( 'NONE',  ( 358.3431457505076310, 165.0000000000000000, -340.0000000000000568 ) ) ;
#40427=ORIENTED_EDGE ( 'NONE', *, *, #20011, .F. ) ;
#40435=EDGE_CURVE ( 'NONE', #15793, #30452, #38328, .T. ) ;
#40436=EDGE_LOOP ( 'NONE', ( #21927, #2079, #46610, #2913, #39297, #9542, #8739, #48804 ) ) ;
#40437=CARTESIAN_POINT ( 'NONE',  ( 181.0000000000000000, -272.5000000000000000, -98.99999999999990052 ) ) ;
#40440=FACE_OUTER_BOUND ( 'NONE', #15342, .T. ) ;
#40441=ADVANCED_FACE ( 'NONE', ( #39546 ), #7989, .T. ) ;
#40445=CARTESIAN_POINT ( 'NONE',  ( 344.0000000000000000, -169.0000000000001137, -349.9999999999998863 ) ) ;
#40449=MECHANICAL_DESIGN_GEOMETRIC_PRESENTATION_REPRESENTATION('',(#32214),#4404);
#40452=AXIS2_PLACEMENT_3D ( 'NONE', #10896, #19356, #35041 ) ;
#40453=DIRECTION ( 'NONE',  ( 1.000000000000000000, 0.000000000000000000, -1.586032892321652482E-16 ) ) ;
#40454=ORIENTED_EDGE ( 'NONE', *, *, #8276, .F. ) ;
#40458=EDGE_LOOP ( 'NONE', ( #83, #18631, #1088, #32987 ) ) ;
#40462=CARTESIAN_POINT ( 'NONE',  ( 357.1715728752537871, -183.0000000000001137, -358.0000000000003411 ) ) ;
#40465=EDGE_LOOP ( 'NONE', ( #32784, #24199, #37072, #13496 ) ) ;
#40467=CARTESIAN_POINT ( 'NONE',  ( 166.9999999999999716, -268.4999999999999432, -349.9999999999999432 ) ) ;
#40473=DIRECTION ( 'NONE',  ( 0.000000000000000000, 1.000000000000000000, 6.123233995736766036E-17 ) ) ;
#40476=ORIENTED_EDGE ( 'NONE', *, *, #12928, .F. ) ;
#40480=VERTEX_POINT ( 'NONE', #27980 ) ;
#40482=ORIENTED_EDGE ( 'NONE', *, *, #39671, .F. ) ;
#40488=LINE ( 'NONE', #5324, #50117 ) ;
#40491=FACE_BOUND ( 'NONE', #38972, .T. ) ;
#40493=FACE_OUTER_BOUND ( 'NONE', #24849, .T. ) ;
#40499=AXIS2_PLACEMENT_3D ( 'NONE', #10324, #11270, #5954 ) ;
#40511=VECTOR ( 'NONE', #211, 1000.000000000000000 ) ;
#40512=VERTEX_POINT ( 'NONE', #46683 ) ;
#40519=ORIENTED_EDGE ( 'NONE', *, *, #43322, .F. ) ;
#40522=CARTESIAN_POINT ( 'NONE',  ( 4.999999999999999112, 175.0000000000000284, 350.0000000000002274 ) ) ;
#40525=DIRECTION ( 'NONE',  ( -2.775557561562891351E-16, -0.7071067811865474617, 0.7071067811865475727 ) ) ;
#40547=DIRECTION ( 'NONE',  ( -1.000000000000000000, 0.000000000000000000, 0.000000000000000000 ) ) ;
#40548=CARTESIAN_POINT ( 'NONE',  ( 343.9999999999998863, -165.0000000000001137, -90.00000000000018474 ) ) ;
#40555=FACE_OUTER_BOUND ( 'NONE', #3774, .T. ) ;
#40561=ADVANCED_FACE ( 'NONE', ( #292 ), #16188, .T. ) ;
#40569=AXIS2_PLACEMENT_3D ( 'NONE', #27326, #31185, #11671 ) ;
#40573=VECTOR ( 'NONE', #36297, 1000.000000000000000 ) ;
#40580=VECTOR ( 'NONE', #34304, 1000.000000000000000 ) ;
#40586=DIRECTION ( 'NONE',  ( -3.172065745548403743E-16, -1.000000000000000000, 0.000000000000000000 ) ) ;
#40593=CIRCLE ( 'NONE', #18448, 2.000000000000001776 ) ;
#40599=EDGE_LOOP ( 'NONE', ( #7264, #27978, #42441, #6334 ) ) ;
#40603=FACE_OUTER_BOUND ( 'NONE', #23164, .T. ) ;
#40605=PLANE ( 'NONE',  #25925 ) ;
#40606=CARTESIAN_POINT ( 'NONE',  ( -5.000000000000000000, 184.8000000000000114, -359.8000000000002387 ) ) ;
#40608=VECTOR ( 'NONE', #23668, 1000.000000000000000 ) ;
#40612=VECTOR ( 'NONE', #8712, 1000.000000000000000 ) ;
#40618=ORIENTED_EDGE ( 'NONE', *, *, #18686, .F. ) ;
#40621=ORIENTED_EDGE ( 'NONE', *, *, #22812, .F. ) ;
#40622=DIRECTION ( 'NONE',  ( 0.000000000000000000, 0.000000000000000000, -1.000000000000000000 ) ) ;
#40626=ADVANCED_FACE ( 'NONE', ( #28745 ), #28491, .F. ) ;
#40629=AXIS2_PLACEMENT_3D ( 'NONE', #2286, #38228, #34612 ) ;
#40638=ORIENTED_EDGE ( 'NONE', *, *, #30354, .T. ) ;
#40639=DIRECTION ( 'NONE',  ( 1.000000000000000000, 0.000000000000000000, 0.000000000000000000 ) ) ;
#40641=LINE ( 'NONE', #44707, #831 ) ;
#40642=CARTESIAN_POINT ( 'NONE',  ( 165.0000000000000000, -174.9999999999999716, -99.00000000000014211 ) ) ;
#40646=VECTOR ( 'NONE', #19492, 1000.000000000000000 ) ;
#40649=EDGE_CURVE ( 'NONE', #17911, #11545, #23283, .T. ) ;
#40650=CIRCLE ( 'NONE', #3757, 4.000000000000003553 ) ;
#40651=CARTESIAN_POINT ( 'NONE',  ( 185.0000000000000568, 165.0000000000000000, 355.9999999999998863 ) ) ;
#40656=DIRECTION ( 'NONE',  ( 0.000000000000000000, -1.000000000000000000, 2.537652627714643577E-15 ) ) ;
#40661=EDGE_LOOP ( 'NONE', ( #36019, #5489, #1887, #48299 ) ) ;
#40682=ORIENTED_EDGE ( 'NONE', *, *, #39641, .F. ) ;
#40689=LINE ( 'NONE', #40931, #44554 ) ;
#40690=VECTOR ( 'NONE', #12384, 1000.000000000000000 ) ;
#40692=DIRECTION ( 'NONE',  ( 0.000000000000000000, 0.000000000000000000, 1.000000000000000000 ) ) ;
#40694=CARTESIAN_POINT ( 'NONE',  ( 359.9999999999999432, -181.0000000000001137, -356.0000000000003411 ) ) ;
#40696=VECTOR ( 'NONE', #47679, 1000.000000000000000 ) ;
#40699=CARTESIAN_POINT ( 'NONE',  ( 360.0000000000000000, -174.9999999999999147, 343.9999999999998295 ) ) ;
#40703=ORIENTED_EDGE ( 'NONE', *, *, #42406, .F. ) ;
#40720=VERTEX_POINT ( 'NONE', #42046 ) ;
#40725=EDGE_CURVE ( 'NONE', #19163, #34763, #21710, .T. ) ;
#40732=ORIENTED_EDGE ( 'NONE', *, *, #1831, .T. ) ;
#40734=DIRECTION ( 'NONE',  ( 0.000000000000000000, -0.000000000000000000, 1.000000000000000000 ) ) ;
#40743=DIRECTION ( 'NONE',  ( -3.172065784643302499E-16, -1.000000000000000000, 2.537652627714642000E-15 ) ) ;
#40753=ORIENTED_EDGE ( 'NONE', *, *, #873, .F. ) ;
#40755=CARTESIAN_POINT ( 'NONE',  ( 168.9999999999999716, 8.000000000000062172, -350.0000000000001705 ) ) ;
#40756=CARTESIAN_POINT ( 'NONE',  ( 5.551115123125782702E-14, -166.9999999999999432, 343.9999999999997726 ) ) ;
#40761=DIRECTION ( 'NONE',  ( 0.000000000000000000, 0.000000000000000000, -1.000000000000000000 ) ) ;
#40769=ORIENTED_EDGE ( 'NONE', *, *, #5854, .F. ) ;
#40774=ORIENTED_EDGE ( 'NONE', *, *, #29599, .T. ) ;
#40784=CARTESIAN_POINT ( 'NONE',  ( 0.000000000000000000, -184.9999999999999716, -344.0000000000001705 ) ) ;
#40785=CARTESIAN_POINT ( 'NONE',  ( 339.9999999999999432, 169.0000000000000000, -344.0000000000001137 ) ) ;
#40792=ORIENTED_EDGE ( 'NONE', *, *, #723, .F. ) ;
#40798=CARTESIAN_POINT ( 'NONE',  ( 344.0000000000000000, -174.9999999999999716, 343.9999999999998295 ) ) ;
#40805=FACE_OUTER_BOUND ( 'NONE', #20814, .T. ) ;
#40809=DIRECTION ( 'NONE',  ( 0.000000000000000000, 1.000000000000000000, 0.000000000000000000 ) ) ;
#40812=CARTESIAN_POINT ( 'NONE',  ( 0.000000000000000000, 175.0000000000000284, 350.0000000000002274 ) ) ;
#40816=AXIS2_PLACEMENT_3D ( 'NONE', #28687, #47638, #25343 ) ;
#40817=ORIENTED_EDGE ( 'NONE', *, *, #48078, .F. ) ;
#40818=DIRECTION ( 'NONE',  ( -4.758098676964957447E-16, -1.000000000000000000, 7.143884938411937192E-48 ) ) ;
#40823=ORIENTED_EDGE ( 'NONE', *, *, #36491, .T. ) ;
#40834=VERTEX_POINT ( 'NONE', #42793 ) ;
#40835=CARTESIAN_POINT ( 'NONE',  ( 181.0000000000001705, -184.9999999999999716, -115.0000000000001279 ) ) ;
#40842=CARTESIAN_POINT ( 'NONE',  ( 339.9999999999998863, -180.9999999999999716, 357.9999999999997726 ) ) ;
#40848=CIRCLE ( 'NONE', #19521, 3.749999999999975575 ) ;
#40851=DIRECTION ( 'NONE',  ( -3.172065784643302499E-16, -1.000000000000000000, 2.537652627714642000E-15 ) ) ;
#40855=CARTESIAN_POINT ( 'NONE',  ( 355.9999999999999432, -185.0000000000001421, -349.9999999999998863 ) ) ;
#40871=DIRECTION ( 'NONE',  ( 1.000000000000000000, 0.000000000000000000, 0.000000000000000000 ) ) ;
#40884=VECTOR ( 'NONE', #21673, 1000.000000000000000 ) ;
#40885=ORIENTED_EDGE ( 'NONE', *, *, #7409, .F. ) ;
#40886=VECTOR ( 'NONE', #5907, 1000.000000000000000 ) ;
#40893=ORIENTED_EDGE ( 'NONE', *, *, #13266, .T. ) ;
#40901=ORIENTED_EDGE ( 'NONE', *, *, #12166, .T. ) ;
#40905=FACE_OUTER_BOUND ( 'NONE', #20089, .T. ) ;
#40907=PLANE ( 'NONE',  #5917 ) ;
#40913=FACE_OUTER_BOUND ( 'NONE', #23862, .T. ) ;
#40923=CIRCLE ( 'NONE', #29452, 4.000000000000003553 ) ;
#40928=LINE ( 'NONE', #36608, #22013 ) ;
#40931=CARTESIAN_POINT ( 'NONE',  ( 168.9999999999999716, 8.000000000000062172, -340.0000000000001137 ) ) ;
#40933=AXIS2_PLACEMENT_3D ( 'NONE', #44050, #29183, #47874 ) ;
#40936=CARTESIAN_POINT ( 'NONE',  ( 340.0000000000000568, 169.0000000000000000, 357.9999999999997726 ) ) ;
#40937=CARTESIAN_POINT ( 'NONE',  ( 0.000000000000000000, -175.0000000000000284, -350.0000000000002274 ) ) ;
#40947=CARTESIAN_POINT ( 'NONE',  ( 360.0000000000000568, 3.000000000000085709, 177.9999999999998295 ) ) ;
#40948=EDGE_CURVE ( 'NONE', #7451, #37196, #36666, .T. ) ;
#40955=DIRECTION ( 'NONE',  ( -1.000000000000000000, 0.000000000000000000, -7.793956916774525800E-48 ) ) ;
#40960=LINE ( 'NONE', #33517, #43909 ) ;
#40962=AXIS2_PLACEMENT_3D ( 'NONE', #14813, #11232, #50158 ) ;
#40963=CIRCLE ( 'NONE', #22134, 2.000000000000001776 ) ;
#40964=VERTEX_POINT ( 'NONE', #16370 ) ;
#40965=EDGE_CURVE ( 'NONE', #34447, #9708, #10223, .T. ) ;
#40973=CARTESIAN_POINT ( 'NONE',  ( 166.9999999999999716, -168.9999999999999147, -340.0000000000001137 ) ) ;
#40977=DIRECTION ( 'NONE',  ( -1.000000000000000000, 0.000000000000000000, 0.000000000000000000 ) ) ;
#40980=ORIENTED_EDGE ( 'NONE', *, *, #11822, .T. ) ;
#40982=DIRECTION ( 'NONE',  ( 0.000000000000000000, -1.000000000000000000, 0.000000000000000000 ) ) ;
#40984=EDGE_LOOP ( 'NONE', ( #43157, #9865, #18404, #38695 ) ) ;
#40993=CARTESIAN_POINT ( 'NONE',  ( 183.0000000000000284, -168.9999999999999432, -115.0000000000001847 ) ) ;
#40999=DIRECTION ( 'NONE',  ( 0.000000000000000000, 0.000000000000000000, 1.000000000000000000 ) ) ;
#41004=LINE ( 'NONE', #41752, #10278 ) ;
#41005=VECTOR ( 'NONE', #20491, 1000.000000000000000 ) ;
#41014=CARTESIAN_POINT ( 'NONE',  ( 343.9999999999999432, 174.9999999999996589, -356.0000000000003411 ) ) ;
#41022=DIRECTION ( 'NONE',  ( 1.000000000000000000, 0.000000000000000000, 0.000000000000000000 ) ) ;
#41030=CARTESIAN_POINT ( 'NONE',  ( 339.9999999999999432, -180.9999999999999716, -342.0000000000001705 ) ) ;
#41031=ORIENTED_EDGE ( 'NONE', *, *, #18623, .T. ) ;
#41033=AXIS2_PLACEMENT_3D ( 'NONE', #31507, #39463, #19937 ) ;
#41036=FACE_OUTER_BOUND ( 'NONE', #35139, .T. ) ;
#41042=DIRECTION ( 'NONE',  ( -1.000000000000000000, 0.000000000000000000, -1.612977847700450206E-50 ) ) ;
#41044=VERTEX_POINT ( 'NONE', #9679 ) ;
#41054=ORIENTED_EDGE ( 'NONE', *, *, #11067, .T. ) ;
#41062=CARTESIAN_POINT ( 'NONE',  ( 166.9999999999999716, -174.9999999999999716, -344.0000000000001137 ) ) ;
#41068=EDGE_CURVE ( 'NONE', #25245, #30746, #32355, .T. ) ;
#41069=EDGE_LOOP ( 'NONE', ( #37014, #48522, #21598, #19525 ) ) ;
#41074=EDGE_CURVE ( 'NONE', #8464, #7855, #6339, .T. ) ;
#41081=ORIENTED_EDGE ( 'NONE', *, *, #29564, .T. ) ;
#41085=CARTESIAN_POINT ( 'NONE',  ( 0.000000000000000000, -184.9999999999999716, -356.0000000000002274 ) ) ;
#41088=ORIENTED_EDGE ( 'NONE', *, *, #44744, .T. ) ;
#41093=DIRECTION ( 'NONE',  ( -1.586032880504786307E-16, 1.654361225106055350E-24, -1.000000000000000000 ) ) ;
#41097=VECTOR ( 'NONE', #41564, 1000.000000000000000 ) ;
#41099=ORIENTED_EDGE ( 'NONE', *, *, #1749, .F. ) ;
#41100=LINE ( 'NONE', #40842, #7979 ) ;
#41107=ORIENTED_EDGE ( 'NONE', *, *, #46575, .T. ) ;
#41111=CARTESIAN_POINT ( 'NONE',  ( 360.0000000000000000, -166.6568542494923406, 341.6568542494921417 ) ) ;
#41112=ORIENTED_EDGE ( 'NONE', *, *, #21310, .F. ) ;
#41117=CARTESIAN_POINT ( 'NONE',  ( 350.0000000000000000, 167.0000000000000000, -344.0000000000001705 ) ) ;
#41122=CARTESIAN_POINT ( 'NONE',  ( 0.000000000000000000, -168.9999999999999432, -358.0000000000002274 ) ) ;
#41125=FACE_OUTER_BOUND ( 'NONE', #673, .T. ) ;
#41133=DIRECTION ( 'NONE',  ( -1.000000000000000000, 0.000000000000000000, 0.000000000000000000 ) ) ;
#41134=AXIS2_PLACEMENT_3D ( 'NONE', #21392, #1906, #7208 ) ;
#41141=DIRECTION ( 'NONE',  ( -5.551115123125781470E-17, 0.7071067811865474617, -0.7071067811865474617 ) ) ;
#41150=ORIENTED_EDGE ( 'NONE', *, *, #12107, .T. ) ;
#41153=CIRCLE ( 'NONE', #19870, 2.000000000000001776 ) ;
#41156=ORIENTED_EDGE ( 'NONE', *, *, #36491, .F. ) ;
#41157=ORIENTED_EDGE ( 'NONE', *, *, #47123, .T. ) ;
#41162=ORIENTED_EDGE ( 'NONE', *, *, #33065, .F. ) ;
#41168=DIRECTION ( 'NONE',  ( 0.000000000000000000, 1.000000000000000000, 0.000000000000000000 ) ) ;
#41175=LINE ( 'NONE', #1442, #24040 ) ;
#41179=DIRECTION ( 'NONE',  ( 1.000000000000000000, 0.000000000000000000, -2.958228394578793832E-31 ) ) ;
#41181=CARTESIAN_POINT ( 'NONE',  ( 181.0000000000000000, 165.0000000000000000, -358.0000000000001705 ) ) ;
#41186=ORIENTED_EDGE ( 'NONE', *, *, #1454, .T. ) ;
#41192=CARTESIAN_POINT ( 'NONE',  ( 164.9999999999999716, -184.9999999999999716, -356.0000000000014211 ) ) ;
#41207=ORIENTED_EDGE ( 'NONE', *, *, #3877, .T. ) ;
#41216=PLANE ( 'NONE',  #3003 ) ;
#41222=EDGE_CURVE ( 'NONE', #22458, #25314, #26848, .T. ) ;
#41232=LINE ( 'NONE', #32797, #50248 ) ;
#41234=CIRCLE ( 'NONE', #19917, 4.000000000000003553 ) ;
#41251=DIRECTION ( 'NONE',  ( -1.000000000000000000, 0.000000000000000000, 1.860490536778032451E-50 ) ) ;
#41253=DIRECTION ( 'NONE',  ( 1.860490536778032451E-50, 0.000000000000000000, 1.000000000000000000 ) ) ;
#41259=EDGE_LOOP ( 'NONE', ( #35017, #18664, #35025, #14059 ) ) ;
#41264=AXIS2_PLACEMENT_3D ( 'NONE', #6682, #11042, #30547 ) ;
#41267=CIRCLE ( 'NONE', #42071, 2.000000000000001776 ) ;
#41274=DIRECTION ( 'NONE',  ( -0.000000000000000000, 1.000000000000000000, 0.000000000000000000 ) ) ;
#41281=CARTESIAN_POINT ( 'NONE',  ( 169.0000000000000000, -174.9999999999999716, -111.0000000000001563 ) ) ;
#41282=EDGE_LOOP ( 'NONE', ( #11363, #9911, #34331, #7861, #40210, #27923, #44634, #879 ) ) ;
#41283=ORIENTED_EDGE ( 'NONE', *, *, #20547, .T. ) ;
#41289=ORIENTED_EDGE ( 'NONE', *, *, #23022, .T. ) ;
#41291=CARTESIAN_POINT ( 'NONE',  ( 0.000000000000000000, 169.0000000000000000, -356.0000000000002274 ) ) ;
#41300=CARTESIAN_POINT ( 'NONE',  ( 165.0000000000000000, -174.9999999999999716, -111.0000000000001563 ) ) ;
#41310=CARTESIAN_POINT ( 'NONE',  ( 181.0000000000000000, -254.4999999999999432, -349.9999999999999432 ) ) ;
#41311=FACE_OUTER_BOUND ( 'NONE', #11634, .T. ) ;
#41313=PLANE ( 'NONE',  #14875 ) ;
#41315=DIRECTION ( 'NONE',  ( 0.000000000000000000, 1.000000000000000000, -2.537652627714642000E-15 ) ) ;
#41319=CARTESIAN_POINT ( 'NONE',  ( 356.0000000000002842, 165.0000000000000000, -110.0000000000002132 ) ) ;
#41320=ORIENTED_EDGE ( 'NONE', *, *, #31861, .F. ) ;
#41330=VECTOR ( 'NONE', #13969, 1000.000000000000000 ) ;
#41338=ORIENTED_EDGE ( 'NONE', *, *, #9817, .T. ) ;
#41339=VERTEX_POINT ( 'NONE', #8862 ) ;
#41343=EDGE_CURVE ( 'NONE', #39358, #39539, #6521, .T. ) ;
#41351=AXIS2_PLACEMENT_3D ( 'NONE', #41486, #30184, #5830 ) ;
#41360=ORIENTED_EDGE ( 'NONE', *, *, #1922, .T. ) ;
#41365=ADVANCED_FACE ( 'NONE', ( #33989 ), #41426, .F. ) ;
#41380=DIRECTION ( 'NONE',  ( 0.000000000000000000, 0.000000000000000000, -1.000000000000000000 ) ) ;
#41383=ORIENTED_EDGE ( 'NONE', *, *, #33534, .T. ) ;
#41384=VECTOR ( 'NONE', #44708, 1000.000000000000000 ) ;
#41408=VECTOR ( 'NONE', #22000, 1000.000000000000000 ) ;
#41416=( GEOMETRIC_REPRESENTATION_CONTEXT ( 3 ) GLOBAL_UNCERTAINTY_ASSIGNED_CONTEXT ( ( #31119 ) ) GLOBAL_UNIT_ASSIGNED_CONTEXT ( ( #19591, #3944, #4209 ) ) REPRESENTATION_CONTEXT ( 'NONE', 'WORKASPACE' ) );
#41418=VECTOR ( 'NONE', #37157, 1000.000000000000000 ) ;
#41426=PLANE ( 'NONE',  #26630 ) ;
#41431=DIRECTION ( 'NONE',  ( -1.000000000000000000, 0.000000000000000000, 0.000000000000000000 ) ) ;
#41436=DIRECTION ( 'NONE',  ( 0.000000000000000000, 1.000000000000000000, 0.000000000000000000 ) ) ;
#41440=CARTESIAN_POINT ( 'NONE',  ( 185.0000000000000000, -81.49999999999997158, -350.0000000000001705 ) ) ;
#41460=LINE ( 'NONE', #41961, #16055 ) ;
#41463=ORIENTED_EDGE ( 'NONE', *, *, #36405, .F. ) ;
#41468=VERTEX_POINT ( 'NONE', #14211 ) ;
#41469=FACE_OUTER_BOUND ( 'NONE', #22709, .T. ) ;
#41473=LINE ( 'NONE', #10926, #43959 ) ;
#41477=ORIENTED_EDGE ( 'NONE', *, *, #5754, .T. ) ;
#41481=ADVANCED_FACE ( 'NONE', ( #37098 ), #13715, .F. ) ;
#41486=CARTESIAN_POINT ( 'NONE',  ( 181.0000000000000000, -168.9999999999999432, -340.0000000000001137 ) ) ;
#41489=CIRCLE ( 'NONE', #22624, 4.000000000000003553 ) ;
#41490=DIRECTION ( 'NONE',  ( 0.000000000000000000, 1.000000000000000000, 0.000000000000000000 ) ) ;
#41497=DIRECTION ( 'NONE',  ( 0.000000000000000000, -1.000000000000000000, -3.186989995019654210E-49 ) ) ;
#41501=ORIENTED_EDGE ( 'NONE', *, *, #5889, .F. ) ;
#41502=DIRECTION ( 'NONE',  ( -0.000000000000000000, 1.000000000000000000, 0.000000000000000000 ) ) ;
#41507=EDGE_CURVE ( 'NONE', #35844, #38360, #34762, .T. ) ;
#41511=VECTOR ( 'NONE', #41780, 1000.000000000000000 ) ;
#41513=ORIENTED_EDGE ( 'NONE', *, *, #2147, .T. ) ;
#41516=CARTESIAN_POINT ( 'NONE',  ( 168.9999999999999716, 10.00000000000006395, -340.0000000000001137 ) ) ;
#41526=LINE ( 'NONE', #5870, #27791 ) ;
#41528=CARTESIAN_POINT ( 'NONE',  ( 341.9999999999999432, 167.8284271247462982, -342.8284271247464972 ) ) ;
#41534=CARTESIAN_POINT ( 'NONE',  ( 181.0000000000000568, 175.0000000000000284, 341.9999999999998863 ) ) ;
#41536=EDGE_LOOP ( 'NONE', ( #17457, #32523, #41150, #9609, #29653, #41915, #10032, #49074 ) ) ;
#41546=EDGE_CURVE ( 'NONE', #43135, #11587, #9446, .T. ) ;
#41551=CIRCLE ( 'NONE', #48056, 3.749999999999975575 ) ;
#41557=ORIENTED_EDGE ( 'NONE', *, *, #35712, .T. ) ;
#41558=LINE ( 'NONE', #2301, #30632 ) ;
#41560=ADVANCED_FACE ( 'NONE', ( #19076 ), #50338, .T. ) ;
#41562=CYLINDRICAL_SURFACE ( 'NONE', #6006, 2.000000000000001776 ) ;
#41564=DIRECTION ( 'NONE',  ( -1.000000000000000000, 0.000000000000000000, 1.860490536778032451E-50 ) ) ;
#41572=ADVANCED_FACE ( 'NONE', ( #8316 ), #31921, .T. ) ;
#41575=VERTEX_POINT ( 'NONE', #32665 ) ;
#41579=EDGE_CURVE ( 'NONE', #23455, #15608, #9064, .T. ) ;
#41591=ORIENTED_EDGE ( 'NONE', *, *, #32601, .F. ) ;
#41598=LINE ( 'NONE', #29043, #10063 ) ;
#41599=EDGE_LOOP ( 'NONE', ( #14832, #5949, #18613, #33838 ) ) ;
#41612=CARTESIAN_POINT ( 'NONE',  ( 339.9999999999999432, 185.0000000000000284, -344.0000000000001137 ) ) ;
#41621=CARTESIAN_POINT ( 'NONE',  ( 340.0000000000000568, 172.0000000000000000, 346.9999999999998863 ) ) ;
#41625=DIRECTION ( 'NONE',  ( 1.000000000000000000, -1.331116318405244905E-23, -4.755310728521421461E-16 ) ) ;
#41627=EDGE_LOOP ( 'NONE', ( #21660, #3873, #2190, #34808 ) ) ;
#41628=LINE ( 'NONE', #26235, #40308 ) ;
#41629=CARTESIAN_POINT ( 'NONE',  ( 168.9999999999999716, -182.9999999999999716, -115.0000000000001279 ) ) ;
#41632=CARTESIAN_POINT ( 'NONE',  ( 344.0000000000000000, -174.9999999999999432, 341.9999999999998295 ) ) ;
#41634=ORIENTED_EDGE ( 'NONE', *, *, #13144, .T. ) ;
#41635=DIRECTION ( 'NONE',  ( 0.000000000000000000, 0.000000000000000000, -1.000000000000000000 ) ) ;
#41640=EDGE_CURVE ( 'NONE', #23492, #891, #39796, .T. ) ;
#41648=DIRECTION ( 'NONE',  ( 0.000000000000000000, 1.000000000000000000, 7.004339610132985974E-48 ) ) ;
#41662=EDGE_LOOP ( 'NONE', ( #19307, #28056, #30443, #27131 ) ) ;
#41665=AXIS2_PLACEMENT_3D ( 'NONE', #45425, #21601, #44919 ) ;
#41667=FACE_OUTER_BOUND ( 'NONE', #7598, .T. ) ;
#41669=ORIENTED_EDGE ( 'NONE', *, *, #28887, .T. ) ;
#41675=EDGE_CURVE ( 'NONE', #8483, #31718, #6225, .T. ) ;
#41676=DIRECTION ( 'NONE',  ( 0.000000000000000000, 0.000000000000000000, -1.000000000000000000 ) ) ;
#41678=FACE_OUTER_BOUND ( 'NONE', #3127, .T. ) ;
#41681=DIRECTION ( 'NONE',  ( 0.000000000000000000, -1.000000000000000000, -3.186989995019654210E-49 ) ) ;
#41683=ORIENTED_EDGE ( 'NONE', *, *, #8751, .F. ) ;
#41686=CARTESIAN_POINT ( 'NONE',  ( 339.9999999999999432, 169.0000000000000000, -356.0000000000002274 ) ) ;
#41688=VECTOR ( 'NONE', #30653, 1000.000000000000000 ) ;
#41692=EDGE_CURVE ( 'NONE', #37196, #36547, #13401, .T. ) ;
#41696=AXIS2_PLACEMENT_3D ( 'NONE', #46099, #6385, #10994 ) ;
#41700=EDGE_CURVE ( 'NONE', #218, #23671, #15208, .T. ) ;
#41707=EDGE_CURVE ( 'NONE', #6226, #48323, #6460, .T. ) ;
#41708=CARTESIAN_POINT ( 'NONE',  ( 342.8284271247461561, -167.0000000000001137, -342.0000000000002842 ) ) ;
#41709=DIRECTION ( 'NONE',  ( 0.000000000000000000, -1.000000000000000000, -0.000000000000000000 ) ) ;
#41713=DIRECTION ( 'NONE',  ( -1.000000000000000000, 0.000000000000000000, -2.958228394578794270E-31 ) ) ;
#41722=DIRECTION ( 'NONE',  ( 1.000000000000000000, 0.000000000000000000, -1.586032892321651989E-16 ) ) ;
#41725=CIRCLE ( 'NONE', #27824, 2.000000000000001776 ) ;
#41726=DIRECTION ( 'NONE',  ( 0.000000000000000000, -1.000000000000000000, -3.186989995019654210E-49 ) ) ;
#41732=AXIS2_PLACEMENT_3D ( 'NONE', #33316, #13782, #33061 ) ;
#41740=DIRECTION ( 'NONE',  ( -1.000000000000000000, 0.000000000000000000, 0.000000000000000000 ) ) ;
#41749=ORIENTED_EDGE ( 'NONE', *, *, #49764, .F. ) ;
#41752=CARTESIAN_POINT ( 'NONE',  ( 4.999999999999999112, 175.0000000000000284, 346.2500000000002274 ) ) ;
#41753=VECTOR ( 'NONE', #25433, 1000.000000000000000 ) ;
#41754=AXIS2_PLACEMENT_3D ( 'NONE', #36163, #8718, #24366 ) ;
#41755=ORIENTED_EDGE ( 'NONE', *, *, #39600, .F. ) ;
#41756=LINE ( 'NONE', #2252, #26202 ) ;
#41759=CARTESIAN_POINT ( 'NONE',  ( 350.0000000000000000, -180.9999999999999716, -356.0000000000002274 ) ) ;
#41767=VERTEX_POINT ( 'NONE', #33435 ) ;
#41780=DIRECTION ( 'NONE',  ( 6.203854594147707562E-25, -2.067951531382569187E-25, 1.000000000000000000 ) ) ;
#41788=VERTEX_POINT ( 'NONE', #2365 ) ;
#41789=VECTOR ( 'NONE', #50441, 1000.000000000000000 ) ;
#41793=DIRECTION ( 'NONE',  ( 1.000000000000000000, 0.000000000000000000, 0.000000000000000000 ) ) ;
#41794=EDGE_CURVE ( 'NONE', #32061, #25893, #48769, .T. ) ;
#41805=AXIS2_PLACEMENT_3D ( 'NONE', #24871, #40525, #5363 ) ;
#41810=ORIENTED_EDGE ( 'NONE', *, *, #20109, .T. ) ;
#41813=CARTESIAN_POINT ( 'NONE',  ( 339.9999999999998863, -180.9999999999999716, 355.9999999999997726 ) ) ;
#41824=ORIENTED_EDGE ( 'NONE', *, *, #3883, .T. ) ;
#41829=LINE ( 'NONE', #49732, #26523 ) ;
#41835=ORIENTED_EDGE ( 'NONE', *, *, #9110, .F. ) ;
#41837=CARTESIAN_POINT ( 'NONE',  ( 0.000000000000000000, 169.0000000000000000, 355.9999999999997726 ) ) ;
#41842=VECTOR ( 'NONE', #18120, 1000.000000000000000 ) ;
#41843=EDGE_LOOP ( 'NONE', ( #10546, #20335, #25008, #23487 ) ) ;
#41846=CARTESIAN_POINT ( 'NONE',  ( 0.000000000000000000, 175.0000000000000284, -350.0000000000002274 ) ) ;
#41847=ORIENTED_EDGE ( 'NONE', *, *, #39399, .F. ) ;
#41849=DIRECTION ( 'NONE',  ( -1.000000000000000000, 0.000000000000000000, -1.612977847700450206E-50 ) ) ;
#41852=CARTESIAN_POINT ( 'NONE',  ( 166.9999999999999716, -81.49999999999997158, -340.0000000000001137 ) ) ;
#41863=ORIENTED_EDGE ( 'NONE', *, *, #49039, .T. ) ;
#41874=DIRECTION ( 'NONE',  ( -0.000000000000000000, -0.000000000000000000, 1.000000000000000000 ) ) ;
#41877=ORIENTED_EDGE ( 'NONE', *, *, #28938, .F. ) ;
#41889=CARTESIAN_POINT ( 'NONE',  ( 350.0000000000000000, 165.0000000000000000, -360.0000000000002274 ) ) ;
#41897=CARTESIAN_POINT ( 'NONE',  ( 181.0000000000000000, -174.9999999999999716, -360.0000000000001705 ) ) ;
#41902=VERTEX_POINT ( 'NONE', #15620 ) ;
#41905=CARTESIAN_POINT ( 'NONE',  ( 339.9999999999998863, -168.9999999999999432, 343.9999999999997726 ) ) ;
#41906=AXIS2_PLACEMENT_3D ( 'NONE', #16891, #28680, #25843 ) ;
#41912=EDGE_CURVE ( 'NONE', #8645, #35844, #31547, .T. ) ;
#41915=ORIENTED_EDGE ( 'NONE', *, *, #17102, .T. ) ;
#41918=CARTESIAN_POINT ( 'NONE',  ( 181.0000000000000284, -272.5000000000000000, -112.9999999999999005 ) ) ;
#41920=EDGE_CURVE ( 'NONE', #1975, #14871, #4816, .T. ) ;
#41926=EDGE_CURVE ( 'NONE', #19760, #9972, #40593, .T. ) ;
#41933=ORIENTED_EDGE ( 'NONE', *, *, #40649, .F. ) ;
#41940=EDGE_LOOP ( 'NONE', ( #24925, #28857, #34548, #16361 ) ) ;
#41946=CARTESIAN_POINT ( 'NONE',  ( 181.0000000000000000, 6.000000000000060396, -350.0000000000001705 ) ) ;
#41948=CARTESIAN_POINT ( 'NONE',  ( 164.9999999999999716, -81.49999999999998579, -340.0000000000001137 ) ) ;
#41950=LINE ( 'NONE', #10401, #27 ) ;
#41959=ORIENTED_EDGE ( 'NONE', *, *, #15123, .T. ) ;
#41961=CARTESIAN_POINT ( 'NONE',  ( 349.9999999999999432, -168.9999999999999432, 359.9999999999997726 ) ) ;
#41963=DIRECTION ( 'NONE',  ( 0.000000000000000000, 1.000000000000000000, 0.000000000000000000 ) ) ;
#41964=ORIENTED_EDGE ( 'NONE', *, *, #3857, .T. ) ;
#41967=CARTESIAN_POINT ( 'NONE',  ( 344.0000000000000568, 167.0000000000000000, 341.9999999999998295 ) ) ;
#41970=ORIENTED_EDGE ( 'NONE', *, *, #47028, .F. ) ;
#41974=DIRECTION ( 'NONE',  ( -4.996003610813203446E-16, -1.000000000000000000, 0.000000000000000000 ) ) ;
#41979=CIRCLE ( 'NONE', #14955, 2.000000000000001776 ) ;
#41981=CARTESIAN_POINT ( 'NONE',  ( 355.9999999999999432, -174.9999999999999432, 357.9999999999998295 ) ) ;
#41988=ORIENTED_EDGE ( 'NONE', *, *, #9185, .F. ) ;
#41992=CYLINDRICAL_SURFACE ( 'NONE', #46029, 2.000000000000001776 ) ;
#41994=CARTESIAN_POINT ( 'NONE',  ( 181.0000000000000284, -9.999999999999953815, -111.0000000000001563 ) ) ;
#42004=FACE_OUTER_BOUND ( 'NONE', #3451, .T. ) ;
#42009=DIRECTION ( 'NONE',  ( -1.000000000000000000, 0.000000000000000000, 0.000000000000000000 ) ) ;
#42020=EDGE_LOOP ( 'NONE', ( #23207, #28464, #25803, #19287 ) ) ;
#42021=EDGE_LOOP ( 'NONE', ( #37491, #14167, #50024, #41157 ) ) ;
#42025=DIRECTION ( 'NONE',  ( -1.000000000000000000, 0.000000000000000000, -7.793956916774525800E-48 ) ) ;
#42028=CYLINDRICAL_SURFACE ( 'NONE', #17387, 4.000000000000003553 ) ;
#42032=DIRECTION ( 'NONE',  ( 0.000000000000000000, 1.000000000000000000, 3.186989995019654210E-49 ) ) ;
#42036=CARTESIAN_POINT ( 'NONE',  ( 358.0000000000001137, 169.0000000000000000, 343.9999999999998863 ) ) ;
#42037=CARTESIAN_POINT ( 'NONE',  ( 339.9999999999999432, 169.0000000000000000, -344.0000000000001705 ) ) ;
#42038=VECTOR ( 'NONE', #34021, 1000.000000000000000 ) ;
#42040=ORIENTED_EDGE ( 'NONE', *, *, #49933, .T. ) ;
#42043=PLANE ( 'NONE',  #20106 ) ;
#42046=CARTESIAN_POINT ( 'NONE',  ( 185.0000000000000000, -268.5000000000000000, -114.9999999999999289 ) ) ;
#42049=LINE ( 'NONE', #14857, #39472 ) ;
#42061=ORIENTED_EDGE ( 'NONE', *, *, #23022, .F. ) ;
#42066=ORIENTED_EDGE ( 'NONE', *, *, #48951, .T. ) ;
#42070=CARTESIAN_POINT ( 'NONE',  ( 339.9999999999998295, -183.3431457505078015, -358.3431457505079152 ) ) ;
#42071=AXIS2_PLACEMENT_3D ( 'NONE', #36155, #44074, #12529 ) ;
#42072=DIRECTION ( 'NONE',  ( -1.000000000000000000, 0.000000000000000000, 0.000000000000000000 ) ) ;
#42080=ORIENTED_EDGE ( 'NONE', *, *, #41920, .T. ) ;
#42082=DIRECTION ( 'NONE',  ( 3.172065745548403743E-16, 1.000000000000000000, 0.000000000000000000 ) ) ;
#42086=CARTESIAN_POINT ( 'NONE',  ( 181.0000000000000000, -272.4999999999999432, -357.9999999999999432 ) ) ;
#42090=CARTESIAN_POINT ( 'NONE',  ( 185.0000000000000000, -272.5000000000000000, -111.0000000000001563 ) ) ;
#42095=CARTESIAN_POINT ( 'NONE',  ( 165.0000000000000000, 6.000000000000060396, 339.9999999999998863 ) ) ;
#42099=VECTOR ( 'NONE', #10535, 1000.000000000000000 ) ;
#42103=EDGE_CURVE ( 'NONE', #29723, #13307, #45310, .T. ) ;
#42110=EDGE_CURVE ( 'NONE', #31887, #27106, #18633, .T. ) ;
#42114=LINE ( 'NONE', #15186, #50371 ) ;
#42132=ORIENTED_EDGE ( 'NONE', *, *, #28133, .T. ) ;
#42136=ORIENTED_EDGE ( 'NONE', *, *, #48777, .F. ) ;
#42138=AXIS2_PLACEMENT_3D ( 'NONE', #35764, #25638, #847 ) ;
#42139=CARTESIAN_POINT ( 'NONE',  ( 355.9999999999998863, -165.0000000000001137, -108.0000000000002132 ) ) ;
#42144=ORIENTED_EDGE ( 'NONE', *, *, #22554, .T. ) ;
#42148=DIRECTION ( 'NONE',  ( -0.000000000000000000, -6.123233995736766036E-17, 1.000000000000000000 ) ) ;
#42154=ORIENTED_EDGE ( 'NONE', *, *, #25813, .T. ) ;
#42164=EDGE_CURVE ( 'NONE', #39568, #42500, #12219, .T. ) ;
#42168=( NAMED_UNIT ( * ) SI_UNIT ( $, .STERADIAN. ) SOLID_ANGLE_UNIT ( ) );
#42171=DIRECTION ( 'NONE',  ( 0.000000000000000000, -2.969158215481698263E-48, 1.000000000000000000 ) ) ;
#42184=DIRECTION ( 'NONE',  ( 0.000000000000000000, 1.000000000000000000, 3.186989995019654210E-49 ) ) ;
#42192=EDGE_CURVE ( 'NONE', #34493, #11678, #38190, .T. ) ;
#42199=CIRCLE ( 'NONE', #12684, 4.000000000000003553 ) ;
#42200=ADVANCED_FACE ( 'NONE', ( #50413 ), #181, .T. ) ;
#42207=EDGE_CURVE ( 'NONE', #11313, #42347, #18882, .T. ) ;
#42209=VERTEX_POINT ( 'NONE', #8383 ) ;
#42220=AXIS2_PLACEMENT_3D ( 'NONE', #3298, #236, #18944 ) ;
#42226=VECTOR ( 'NONE', #21877, 1000.000000000000000 ) ;
#42228=DIRECTION ( 'NONE',  ( 0.000000000000000000, -1.000000000000000000, 0.000000000000000000 ) ) ;
#42236=LINE ( 'NONE', #42986, #44241 ) ;
#42240=ORIENTED_EDGE ( 'NONE', *, *, #10586, .T. ) ;
#42246=AXIS2_PLACEMENT_3D ( 'NONE', #12942, #12198, #24008 ) ;
#42251=AXIS2_PLACEMENT_3D ( 'NONE', #48266, #16763, #29068 ) ;
#42255=VECTOR ( 'NONE', #3525, 1000.000000000000000 ) ;
#42256=FACE_BOUND ( 'NONE', #38334, .T. ) ;
#42260=CIRCLE ( 'NONE', #39840, 4.000000000000003553 ) ;
#42261=CARTESIAN_POINT ( 'NONE',  ( 185.0000000000000284, -174.9999999999999716, -111.0000000000001563 ) ) ;
#42263=ORIENTED_EDGE ( 'NONE', *, *, #17143, .T. ) ;
#42265=ADVANCED_FACE ( 'NONE', ( #35594 ), #428, .F. ) ;
#42268=ORIENTED_EDGE ( 'NONE', *, *, #31986, .T. ) ;
#42269=CARTESIAN_POINT ( 'NONE',  ( 168.9999999999999716, 165.0000000000000000, -340.0000000000001705 ) ) ;
#42270=CARTESIAN_POINT ( 'NONE',  ( 185.0000000000000000, -164.9999999999999432, -344.0000000000001137 ) ) ;
#42278=EDGE_CURVE ( 'NONE', #41788, #37196, #42260, .T. ) ;
#42279=AXIS2_PLACEMENT_3D ( 'NONE', #44843, #17422, #45781 ) ;
#42283=AXIS2_PLACEMENT_3D ( 'NONE', #853, #28545, #355 ) ;
#42287=EDGE_LOOP ( 'NONE', ( #26254, #2779, #1758, #14537 ) ) ;
#42290=LINE ( 'NONE', #49185, #19326 ) ;
#42293=CARTESIAN_POINT ( 'NONE',  ( 168.9999999999999716, 175.0000000000000284, -342.0000000000001137 ) ) ;
#42294=CARTESIAN_POINT ( 'NONE',  ( 355.9999999999999432, -183.0000000000000000, 357.9999999999998295 ) ) ;
#42305=CARTESIAN_POINT ( 'NONE',  ( 181.0000000000000284, -9.999999999999953815, -115.0000000000001563 ) ) ;
#42307=DIRECTION ( 'NONE',  ( 0.000000000000000000, -1.000000000000000000, -0.000000000000000000 ) ) ;
#42313=DIRECTION ( 'NONE',  ( 0.000000000000000000, 0.000000000000000000, 1.000000000000000000 ) ) ;
#42315=CARTESIAN_POINT ( 'NONE',  ( 339.9999999999998863, -182.9999999999999716, 355.9999999999997726 ) ) ;
#42318=EDGE_LOOP ( 'NONE', ( #22605, #23669, #28557, #1391 ) ) ;
#42321=DIRECTION ( 'NONE',  ( 1.132880637372608740E-16, 4.718402560806925739E-50, 1.000000000000000000 ) ) ;
#42326=ORIENTED_EDGE ( 'NONE', *, *, #12660, .T. ) ;
#42327=CARTESIAN_POINT ( 'NONE',  ( 358.0000000000000568, 175.0000000000000284, -94.00000000000019895 ) ) ;
#42331=ORIENTED_EDGE ( 'NONE', *, *, #47261, .T. ) ;
#42332=CARTESIAN_POINT ( 'NONE',  ( 164.9999999999999716, 6.000000000000060396, -350.0000000000001705 ) ) ;
#42336=FACE_OUTER_BOUND ( 'NONE', #49877, .T. ) ;
#42346=DIRECTION ( 'NONE',  ( 0.000000000000000000, 6.123233995736766036E-17, -1.000000000000000000 ) ) ;
#42347=VERTEX_POINT ( 'NONE', #13221 ) ;
#42349=CARTESIAN_POINT ( 'NONE',  ( 185.0000000000000568, 175.0000000000000284, 355.9999999999998863 ) ) ;
#42359=CARTESIAN_POINT ( 'NONE',  ( 339.9999999999999432, 167.0000000000000000, -356.0000000000002274 ) ) ;
#42363=EDGE_LOOP ( 'NONE', ( #262, #30004, #38520, #10536 ) ) ;
#42367=CARTESIAN_POINT ( 'NONE',  ( 164.9999999999999716, -164.9999999999999432, 355.9999999999998863 ) ) ;
#42368=DIRECTION ( 'NONE',  ( 0.000000000000000000, 1.000000000000000000, -2.537652627714643577E-15 ) ) ;
#42369=CARTESIAN_POINT ( 'NONE',  ( 169.0000000000000000, -174.9999999999999716, -111.0000000000001563 ) ) ;
#42374=ORIENTED_EDGE ( 'NONE', *, *, #48789, .F. ) ;
#42376=DIRECTION ( 'NONE',  ( 0.000000000000000000, 0.000000000000000000, -1.000000000000000000 ) ) ;
#42378=VECTOR ( 'NONE', #16160, 1000.000000000000000 ) ;
#42388=CARTESIAN_POINT ( 'NONE',  ( 181.0000000000000000, -93.49999999999998579, -340.0000000000001137 ) ) ;
#42389=VERTEX_POINT ( 'NONE', #32733 ) ;
#42395=DIRECTION ( 'NONE',  ( -1.586032892321652236E-16, -1.000000000000000000, -2.288264760618012091E-48 ) ) ;
#42402=ORIENTED_EDGE ( 'NONE', *, *, #37480, .F. ) ;
#42404=ORIENTED_EDGE ( 'NONE', *, *, #8393, .T. ) ;
#42406=EDGE_CURVE ( 'NONE', #38030, #19831, #25042, .T. ) ;
#42424=DIRECTION ( 'NONE',  ( 1.000000000000000000, -4.758098676964957447E-16, 1.642146637880645005E-47 ) ) ;
#42429=EDGE_CURVE ( 'NONE', #15426, #28175, #3734, .T. ) ;
#42435=FACE_OUTER_BOUND ( 'NONE', #26062, .T. ) ;
#42437=DIRECTION ( 'NONE',  ( 0.000000000000000000, 1.000000000000000000, 0.000000000000000000 ) ) ;
#42439=PLANE ( 'NONE',  #40452 ) ;
#42441=ORIENTED_EDGE ( 'NONE', *, *, #13978, .T. ) ;
#42442=DIRECTION ( 'NONE',  ( 4.755310728521421461E-16, 0.000000000000000000, 1.000000000000000000 ) ) ;
#42447=VECTOR ( 'NONE', #10196, 1000.000000000000000 ) ;
#42450=CARTESIAN_POINT ( 'NONE',  ( 0.000000000000000000, -184.7999999999999545, 359.7999999999997840 ) ) ;
#42451=CARTESIAN_POINT ( 'NONE',  ( 181.0000000000000284, -174.9999999999999716, -115.0000000000001563 ) ) ;
#42456=EDGE_CURVE ( 'NONE', #16943, #19122, #36553, .T. ) ;
#42466=DIRECTION ( 'NONE',  ( -3.172065784643302499E-16, -1.000000000000000000, 2.537652627714642000E-15 ) ) ;
#42469=DIRECTION ( 'NONE',  ( 0.000000000000000000, 0.000000000000000000, -1.000000000000000000 ) ) ;
#42477=CARTESIAN_POINT ( 'NONE',  ( -5.000000000000000000, -165.1999999999999602, -359.8000000000002387 ) ) ;
#42485=LINE ( 'NONE', #18628, #35059 ) ;
#42489=CARTESIAN_POINT ( 'NONE',  ( 341.9999999999999432, -165.0000000000001137, -94.00000000000019895 ) ) ;
#42491=CARTESIAN_POINT ( 'NONE',  ( 349.9999999999999432, -168.9999999999999432, 339.9999999999997726 ) ) ;
#42496=CARTESIAN_POINT ( 'NONE',  ( 183.0000000000000284, -9.999999999999953815, -111.0000000000001563 ) ) ;
#42499=CYLINDRICAL_SURFACE ( 'NONE', #27364, 4.000000000000003553 ) ;
#42500=VERTEX_POINT ( 'NONE', #42941 ) ;
#42507=PLANE ( 'NONE',  #37675 ) ;
#42509=CARTESIAN_POINT ( 'NONE',  ( 185.0000000000000000, -5.999999999999950262, -350.0000000000001705 ) ) ;
#42514=ORIENTED_EDGE ( 'NONE', *, *, #32223, .F. ) ;
#42516=CYLINDRICAL_SURFACE ( 'NONE', #41033, 4.000000000000003553 ) ;
#42517=AXIS2_PLACEMENT_3D ( 'NONE', #9373, #12955, #33252 ) ;
#42518=AXIS2_PLACEMENT_3D ( 'NONE', #12852, #8011, #36479 ) ;
#42520=DIRECTION ( 'NONE',  ( -1.612977847700450206E-50, 0.000000000000000000, -1.000000000000000000 ) ) ;
#42521=CARTESIAN_POINT ( 'NONE',  ( 340.0000000000000568, 181.0000000000000284, 357.9999999999997726 ) ) ;
#42523=AXIS2_PLACEMENT_3D ( 'NONE', #16451, #32358, #32873 ) ;
#42524=VECTOR ( 'NONE', #35386, 1000.000000000000000 ) ;
#42529=CARTESIAN_POINT ( 'NONE',  ( 356.0000000000000000, -165.0000000000001137, -340.0000000000002842 ) ) ;
#42532=ORIENTED_EDGE ( 'NONE', *, *, #2988, .F. ) ;
#42540=LINE ( 'NONE', #12265, #45488 ) ;
#42541=VERTEX_POINT ( 'NONE', #39381 ) ;
#42547=CYLINDRICAL_SURFACE ( 'NONE', #42220, 4.000000000000003553 ) ;
#42571=VERTEX_POINT ( 'NONE', #31424 ) ;
#42573=ORIENTED_EDGE ( 'NONE', *, *, #37821, .F. ) ;
#42576=ORIENTED_EDGE ( 'NONE', *, *, #39681, .T. ) ;
#42580=DIRECTION ( 'NONE',  ( 0.000000000000000000, -2.537652627714642000E-15, -1.000000000000000000 ) ) ;
#42581=ORIENTED_EDGE ( 'NONE', *, *, #22240, .F. ) ;
#42585=VERTEX_POINT ( 'NONE', #11917 ) ;
#42586=ORIENTED_EDGE ( 'NONE', *, *, #38526, .T. ) ;
#42587=CYLINDRICAL_SURFACE ( 'NONE', #22634, 4.000000000000003553 ) ;
#42588=AXIS2_PLACEMENT_3D ( 'NONE', #34923, #27961, #43598 ) ;
#42596=EDGE_LOOP ( 'NONE', ( #6788, #50068, #30609, #1965 ) ) ;
#42597=PLANE ( 'NONE',  #2438 ) ;
#42604=VECTOR ( 'NONE', #39336, 1000.000000000000000 ) ;
#42605=CARTESIAN_POINT ( 'NONE',  ( 183.0000000000000568, 165.0000000000000000, 355.9999999999998863 ) ) ;
#42616=ADVANCED_FACE ( 'NONE', ( #28065 ), #39889, .T. ) ;
#42618=FACE_OUTER_BOUND ( 'NONE', #45650, .T. ) ;
#42627=CIRCLE ( 'NONE', #21323, 2.000000000000001776 ) ;
#42634=ORIENTED_EDGE ( 'NONE', *, *, #26501, .F. ) ;
#42639=AXIS2_PLACEMENT_3D ( 'NONE', #1757, #17399, #33066 ) ;
#42655=ORIENTED_EDGE ( 'NONE', *, *, #23388, .T. ) ;
#42657=LINE ( 'NONE', #8543, #19357 ) ;
#42664=CIRCLE ( 'NONE', #19750, 2.000000000000001776 ) ;
#42665=FACE_OUTER_BOUND ( 'NONE', #8295, .T. ) ;
#42670=DIRECTION ( 'NONE',  ( 9.711650524620651178E-33, -1.223873602809432483E-48, 1.000000000000000000 ) ) ;
#42680=LINE ( 'NONE', #5707, #32691 ) ;
#42681=DIRECTION ( 'NONE',  ( -4.758098676964957447E-16, -1.000000000000000000, 7.143884938411937192E-48 ) ) ;
#42682=LINE ( 'NONE', #3431, #44591 ) ;
#42685=ADVANCED_FACE ( 'NONE', ( #8826 ), #40127, .T. ) ;
#42693=DIRECTION ( 'NONE',  ( 3.363195139050033768E-16, 0.7071067811865474617, 0.7071067811865475727 ) ) ;
#42696=VERTEX_POINT ( 'NONE', #28568 ) ;
#42698=DIRECTION ( 'NONE',  ( -1.000000000000000000, 0.000000000000000000, -4.758098658057970186E-16 ) ) ;
#42702=AXIS2_PLACEMENT_3D ( 'NONE', #34984, #27263, #39082 ) ;
#42703=ORIENTED_EDGE ( 'NONE', *, *, #2638, .T. ) ;
#42706=ORIENTED_EDGE ( 'NONE', *, *, #10529, .F. ) ;
#42707=EDGE_LOOP ( 'NONE', ( #22192, #14976, #31931, #20120, #25823, #13204, #30861, #45152 ) ) ;
#42711=ORIENTED_EDGE ( 'NONE', *, *, #29133, .T. ) ;
#42714=LINE ( 'NONE', #18610, #25082 ) ;
#42718=CARTESIAN_POINT ( 'NONE',  ( 356.0000000000000000, -174.9999999999999147, 343.9999999999998295 ) ) ;
#42723=PLANE ( 'NONE',  #27900 ) ;
#42725=AXIS2_PLACEMENT_3D ( 'NONE', #9055, #24710, #12386 ) ;
#42726=VECTOR ( 'NONE', #19904, 1000.000000000000000 ) ;
#42727=CARTESIAN_POINT ( 'NONE',  ( 360.0000000000000000, 174.9999999999996589, -344.0000000000002842 ) ) ;
#42732=CARTESIAN_POINT ( 'NONE',  ( 169.0000000000000000, -9.999999999999953815, -99.00000000000014211 ) ) ;
#42733=DIRECTION ( 'NONE',  ( 0.000000000000000000, -1.000000000000000000, 0.000000000000000000 ) ) ;
#42750=( NAMED_UNIT ( * ) SI_UNIT ( $, .STERADIAN. ) SOLID_ANGLE_UNIT ( ) );
#42757=VECTOR ( 'NONE', #9735, 1000.000000000000000 ) ;
#42760=EDGE_CURVE ( 'NONE', #13377, #38138, #37067, .T. ) ;
#42761=EDGE_CURVE ( 'NONE', #25084, #3248, #16770, .T. ) ;
#42769=AXIS2_PLACEMENT_3D ( 'NONE', #42844, #12311, #50506 ) ;
#42770=DIRECTION ( 'NONE',  ( 0.000000000000000000, 0.000000000000000000, 1.000000000000000000 ) ) ;
#42772=UNCERTAINTY_MEASURE_WITH_UNIT (LENGTH_MEASURE( 1.000000000000000082E-05 ), #21041, 'distance_accuracy_value', 'NONE');
#42774=EDGE_CURVE ( 'NONE', #44239, #13377, #29573, .T. ) ;
#42776=ORIENTED_EDGE ( 'NONE', *, *, #8900, .T. ) ;
#42777=DIRECTION ( 'NONE',  ( 0.000000000000000000, 2.969158215481698263E-48, -1.000000000000000000 ) ) ;
#42779=( BOUNDED_CURVE ( )  B_SPLINE_CURVE ( 3, ( #33216, #21135, #39902, #32193 ),
 .UNSPECIFIED., .F., .F. ) 
 B_SPLINE_CURVE_WITH_KNOTS ( ( 4, 4 ),
 ( 1.570796326794896780, 3.141592653589460493 ),
 .UNSPECIFIED. ) 
 CURVE ( )  GEOMETRIC_REPRESENTATION_ITEM ( )  RATIONAL_B_SPLINE_CURVE ( ( 1.000000000000000000, 0.8047378541244434302, 0.8047378541244434302, 1.000000000000000000 ) ) 
 REPRESENTATION_ITEM ( '' )  );
#42780=EDGE_LOOP ( 'NONE', ( #47238, #48286, #28982, #1841, #6281, #18661, #17537, #47051 ) ) ;
#42789=CARTESIAN_POINT ( 'NONE',  ( 168.9999999999999716, 175.0000000000000284, -358.0000000000001705 ) ) ;
#42790=ORIENTED_EDGE ( 'NONE', *, *, #49084, .F. ) ;
#42793=CARTESIAN_POINT ( 'NONE',  ( 339.9999999999999432, 181.0000000000000284, -358.0000000000002274 ) ) ;
#42796=EDGE_CURVE ( 'NONE', #47173, #23694, #41628, .T. ) ;
#42806=CARTESIAN_POINT ( 'NONE',  ( -5.000000000000000000, -184.7999999999999545, -359.8000000000002387 ) ) ;
#42807=VECTOR ( 'NONE', #43640, 1000.000000000000000 ) ;
#42814=VERTEX_POINT ( 'NONE', #2132 ) ;
#42815=DIRECTION ( 'NONE',  ( -1.586032880504786307E-16, 1.654361225106055350E-24, -1.000000000000000000 ) ) ;
#42816=EDGE_CURVE ( 'NONE', #18177, #21391, #6707, .T. ) ;
#42821=ORIENTED_EDGE ( 'NONE', *, *, #17960, .T. ) ;
#42823=LINE ( 'NONE', #26934, #32761 ) ;
#42826=DIRECTION ( 'NONE',  ( -4.759647537211363479E-16, 5.772796816983493182E-42, -1.000000000000000000 ) ) ;
#42827=VECTOR ( 'NONE', #43925, 1000.000000000000000 ) ;
#42831=EDGE_CURVE ( 'NONE', #34859, #19251, #30092, .T. ) ;
#42837=CARTESIAN_POINT ( 'NONE',  ( 183.0000000000000000, -184.9999999999999716, -344.0000000000003979 ) ) ;
#42839=CARTESIAN_POINT ( 'NONE',  ( 0.000000000000000000, 165.2000000000000171, -340.2000000000001592 ) ) ;
#42844=CARTESIAN_POINT ( 'NONE',  ( 169.0000000000000000, -9.999999999999953815, -99.00000000000014211 ) ) ;
#42849=DIRECTION ( 'NONE',  ( -4.755310728521421461E-16, 0.000000000000000000, -1.000000000000000000 ) ) ;
#42852=ADVANCED_FACE ( 'NONE', ( #33690 ), #49276, .T. ) ;
#42853=DIRECTION ( 'NONE',  ( -0.000000000000000000, -1.544785076050074834E-48, -1.000000000000000000 ) ) ;
#42860=EDGE_CURVE ( 'NONE', #20632, #28535, #46447, .T. ) ;
#42864=VERTEX_POINT ( 'NONE', #39307 ) ;
#42867=CARTESIAN_POINT ( 'NONE',  ( 181.0000000000000000, -184.9999999999999716, -340.0000000000001705 ) ) ;
#42870=VECTOR ( 'NONE', #34324, 1000.000000000000000 ) ;
#42871=DIRECTION ( 'NONE',  ( -3.172065784643302499E-16, -1.000000000000000000, 2.537652627714642000E-15 ) ) ;
#42873=ORIENTED_EDGE ( 'NONE', *, *, #7338, .F. ) ;
#42875=CIRCLE ( 'NONE', #12556, 2.000000000000001776 ) ;
#42882=AXIS2_PLACEMENT_3D ( 'NONE', #29581, #3894, #30860 ) ;
#42883=DIRECTION ( 'NONE',  ( 1.000000000000000000, 0.000000000000000000, 0.000000000000000000 ) ) ;
#42888=CARTESIAN_POINT ( 'NONE',  ( 181.0000000000000000, -164.9999999999999432, 355.9999999999998863 ) ) ;
#42890=ORIENTED_EDGE ( 'NONE', *, *, #42761, .T. ) ;
#42897=LINE ( 'NONE', #27530, #21360 ) ;
#42898=DIRECTION ( 'NONE',  ( 0.000000000000000000, -0.000000000000000000, 1.000000000000000000 ) ) ;
#42906=ADVANCED_FACE ( 'NONE', ( #45946 ), #43148, .F. ) ;
#42909=DIRECTION ( 'NONE',  ( -1.586032892321652236E-16, -1.000000000000000000, -2.288264760618012091E-48 ) ) ;
#42911=AXIS2_PLACEMENT_3D ( 'NONE', #8281, #36246, #35489 ) ;
#42915=VECTOR ( 'NONE', #1998, 1000.000000000000000 ) ;
#42921=CIRCLE ( 'NONE', #46994, 2.000000000000001776 ) ;
#42925=ORIENTED_EDGE ( 'NONE', *, *, #35137, .F. ) ;
#42926=CARTESIAN_POINT ( 'NONE',  ( 339.9999999999999432, -182.9999999999999716, -344.0000000000001705 ) ) ;
#42927=DIRECTION ( 'NONE',  ( 3.172065745548403743E-16, 1.000000000000000000, 0.000000000000000000 ) ) ;
#42929=FACE_OUTER_BOUND ( 'NONE', #40984, .T. ) ;
#42931=CARTESIAN_POINT ( 'NONE',  ( 181.0000000000000000, -270.4999999999999432, -349.9999999999999432 ) ) ;
#42933=DIRECTION ( 'NONE',  ( -1.586032880504786307E-16, 1.654361225106055350E-24, -1.000000000000000000 ) ) ;
#42936=FACE_BOUND ( 'NONE', #3262, .T. ) ;
#42937=VECTOR ( 'NONE', #49263, 1000.000000000000000 ) ;
#42941=CARTESIAN_POINT ( 'NONE',  ( 181.0000000000000000, -270.5000000000000000, -114.9999999999999147 ) ) ;
#42946=CARTESIAN_POINT ( 'NONE',  ( -5.000000000000000000, -184.7999999999999545, 340.1999999999997044 ) ) ;
#42947=AXIS2_PLACEMENT_3D ( 'NONE', #38960, #8414, #23553 ) ;
#42950=CIRCLE ( 'NONE', #20838, 2.000000000000001776 ) ;
#42953=LINE ( 'NONE', #18835, #7467 ) ;
#42954=AXIS2_PLACEMENT_3D ( 'NONE', #47437, #31340, #15934 ) ;
#42956=DIRECTION ( 'NONE',  ( 0.000000000000000000, -2.969158215481698263E-48, 1.000000000000000000 ) ) ;
#42958=DIRECTION ( 'NONE',  ( 4.379057701015053347E-47, -1.000000000000000000, 2.537652627714642000E-15 ) ) ;
#42961=ORIENTED_EDGE ( 'NONE', *, *, #46197, .T. ) ;
#42964=VECTOR ( 'NONE', #53, 1000.000000000000000 ) ;
#42972=VECTOR ( 'NONE', #46628, 1000.000000000000000 ) ;
#42983=CIRCLE ( 'NONE', #42138, 4.000000000000003553 ) ;
#42984=ORIENTED_EDGE ( 'NONE', *, *, #34567, .T. ) ;
#42985=ORIENTED_EDGE ( 'NONE', *, *, #36494, .F. ) ;
#42986=CARTESIAN_POINT ( 'NONE',  ( 355.9999999999998295, -165.0000000000001137, -108.0000000000002132 ) ) ;
#42990=EDGE_LOOP ( 'NONE', ( #39983, #38444, #42821, #12790 ) ) ;
#42992=AXIS2_PLACEMENT_3D ( 'NONE', #41291, #22545, #45361 ) ;
#42998=DIRECTION ( 'NONE',  ( 0.000000000000000000, 5.664403186863042467E-17, 1.000000000000000000 ) ) ;
#42999=CARTESIAN_POINT ( 'NONE',  ( 339.9999999999999432, -168.9999999999999432, -340.0000000000001705 ) ) ;
#43002=CARTESIAN_POINT ( 'NONE',  ( 339.9999999999998863, -183.3431457505077731, -358.3431457505079720 ) ) ;
#43007=AXIS2_PLACEMENT_3D ( 'NONE', #13608, #29264, #44880 ) ;
#43013=FACE_OUTER_BOUND ( 'NONE', #5002, .T. ) ;
#43016=VECTOR ( 'NONE', #13916, 1000.000000000000000 ) ;
#43022=CARTESIAN_POINT ( 'NONE',  ( 185.0000000000000284, -174.9999999999999716, -99.00000000000014211 ) ) ;
#43038=EDGE_LOOP ( 'NONE', ( #12445, #15353, #20455, #33789, #48477, #35233, #37036, #14335 ) ) ;
#43047=AXIS2_PLACEMENT_3D ( 'NONE', #5709, #8819, #36030 ) ;
#43059=AXIS2_PLACEMENT_3D ( 'NONE', #30135, #17820, #10122 ) ;
#43068=ORIENTED_EDGE ( 'NONE', *, *, #5417, .T. ) ;
#43072=EDGE_CURVE ( 'NONE', #2551, #11678, #43381, .T. ) ;
#43088=EDGE_LOOP ( 'NONE', ( #32982, #15957, #21163, #16548 ) ) ;
#43089=FACE_OUTER_BOUND ( 'NONE', #21885, .T. ) ;
#43090=CARTESIAN_POINT ( 'NONE',  ( 0.000000000000000000, 181.0000000000000284, 355.9999999999997726 ) ) ;
#43091=VECTOR ( 'NONE', #46885, 1000.000000000000000 ) ;
#43095=ORIENTED_EDGE ( 'NONE', *, *, #42192, .T. ) ;
#43098=EDGE_CURVE ( 'NONE', #48433, #31642, #8513, .T. ) ;
#43103=( GEOMETRIC_REPRESENTATION_CONTEXT ( 3 ) GLOBAL_UNCERTAINTY_ASSIGNED_CONTEXT ( ( #32303 ) ) GLOBAL_UNIT_ASSIGNED_CONTEXT ( ( #49817, #35019, #42168 ) ) REPRESENTATION_CONTEXT ( 'NONE', 'WORKASPACE' ) );
#43107=EDGE_CURVE ( 'NONE', #29740, #8815, #13727, .T. ) ;
#43113=AXIS2_PLACEMENT_3D ( 'NONE', #35619, #31255, #6939 ) ;
#43117=LINE ( 'NONE', #16182, #44174 ) ;
#43118=ORIENTED_EDGE ( 'NONE', *, *, #12430, .F. ) ;
#43123=CARTESIAN_POINT ( 'NONE',  ( 344.0000000000000000, -166.9999999999999716, 341.9999999999998295 ) ) ;
#43126=AXIS2_PLACEMENT_3D ( 'NONE', #7791, #26771, #19315 ) ;
#43127=VECTOR ( 'NONE', #40285, 1000.000000000000000 ) ;
#43128=ORIENTED_EDGE ( 'NONE', *, *, #498, .T. ) ;
#43132=LINE ( 'NONE', #557, #10336 ) ;
#43135=VERTEX_POINT ( 'NONE', #31868 ) ;
#43138=VECTOR ( 'NONE', #27479, 1000.000000000000000 ) ;
#43146=VERTEX_POINT ( 'NONE', #4891 ) ;
#43148=CYLINDRICAL_SURFACE ( 'NONE', #18969, 2.000000000000001776 ) ;
#43151=DIRECTION ( 'NONE',  ( 0.000000000000000000, 5.664403186863042467E-17, 1.000000000000000000 ) ) ;
#43153=VECTOR ( 'NONE', #38071, 1000.000000000000000 ) ;
#43157=ORIENTED_EDGE ( 'NONE', *, *, #24604, .T. ) ;
#43158=CARTESIAN_POINT ( 'NONE',  ( 356.0000000000000000, -165.0000000000001137, -94.00000000000019895 ) ) ;
#43160=CARTESIAN_POINT ( 'NONE',  ( 183.0000000000000568, 165.0000000000000000, 343.9999999999998863 ) ) ;
#43166=EDGE_CURVE ( 'NONE', #46434, #18177, #37493, .T. ) ;
#43170=FACE_OUTER_BOUND ( 'NONE', #35822, .T. ) ;
#43178=CYLINDRICAL_SURFACE ( 'NONE', #47190, 4.000000000000003553 ) ;
#43190=EDGE_LOOP ( 'NONE', ( #33885, #43666, #12679, #7632 ) ) ;
#43191=LINE ( 'NONE', #39607, #18128 ) ;
#43197=ORIENTED_EDGE ( 'NONE', *, *, #8013, .F. ) ;
#43204=ADVANCED_FACE ( 'NONE', ( #9501 ), #41313, .T. ) ;
#43205=DIRECTION ( 'NONE',  ( 0.000000000000000000, -1.000000000000000000, -3.186989995019654210E-49 ) ) ;
#43206=VERTEX_POINT ( 'NONE', #2557 ) ;
#43207=ORIENTED_EDGE ( 'NONE', *, *, #45651, .T. ) ;
#43218=EDGE_CURVE ( 'NONE', #4051, #2864, #32096, .T. ) ;
#43224=ORIENTED_EDGE ( 'NONE', *, *, #23670, .T. ) ;
#43226=CARTESIAN_POINT ( 'NONE',  ( 183.0000000000000000, -5.999999999999950262, -340.0000000000001137 ) ) ;
#43227=DIRECTION ( 'NONE',  ( 0.000000000000000000, 1.000000000000000000, 6.123233995736766036E-17 ) ) ;
#43230=ORIENTED_EDGE ( 'NONE', *, *, #14345, .T. ) ;
#43231=DIRECTION ( 'NONE',  ( -1.000000000000000000, 0.000000000000000000, 1.860490536778032451E-50 ) ) ;
#43233=CARTESIAN_POINT ( 'NONE',  ( 356.0000000000000568, 175.0000000000000284, -94.00000000000019895 ) ) ;
#43234=ORIENTED_EDGE ( 'NONE', *, *, #14058, .T. ) ;
#43236=ORIENTED_EDGE ( 'NONE', *, *, #6051, .F. ) ;
#43248=CARTESIAN_POINT ( 'NONE',  ( 344.0000000000000000, 175.0000000000000284, -92.00000000000019895 ) ) ;
#43249=ORIENTED_EDGE ( 'NONE', *, *, #14051, .T. ) ;
#43250=ORIENTED_EDGE ( 'NONE', *, *, #46773, .T. ) ;
#43263=DIRECTION ( 'NONE',  ( -1.000000000000000000, 0.000000000000000000, -2.958228394578794270E-31 ) ) ;
#43269=PLANE ( 'NONE',  #44990 ) ;
#43273=ORIENTED_EDGE ( 'NONE', *, *, #5454, .T. ) ;
#43274=PLANE ( 'NONE',  #36070 ) ;
#43277=DIRECTION ( 'NONE',  ( 0.000000000000000000, -1.000000000000000000, 2.969158215481698263E-48 ) ) ;
#43287=CARTESIAN_POINT ( 'NONE',  ( 350.0000000000000000, -180.9999999999999716, -356.0000000000002274 ) ) ;
#43288=CARTESIAN_POINT ( 'NONE',  ( 167.0000000000000000, -9.999999999999953815, -99.00000000000014211 ) ) ;
#43292=CARTESIAN_POINT ( 'NONE',  ( -5.000000000000000000, -165.1999999999999602, 359.7999999999997840 ) ) ;
#43294=DIRECTION ( 'NONE',  ( -3.172065784643302499E-16, -1.000000000000000000, 2.537652627714642000E-15 ) ) ;
#43296=VECTOR ( 'NONE', #2926, 1000.000000000000000 ) ;
#43300=ORIENTED_EDGE ( 'NONE', *, *, #48868, .F. ) ;
#43305=CLOSED_SHELL ( 'NONE', ( #15803, #21453, #31243, #50594, #29771, #42265, #50541, #49033, #2763, #29134, #30855, #5154, #16602, #12640, #12973, #26172, #36735, #16754 ) ) ;
#43322=EDGE_CURVE ( 'NONE', #38973, #2035, #6657, .T. ) ;
#43325=CARTESIAN_POINT ( 'NONE',  ( 0.000000000000000000, 167.0000000000000000, -356.0000000000002274 ) ) ;
#43339=VECTOR ( 'NONE', #795, 1000.000000000000000 ) ;
#43344=CARTESIAN_POINT ( 'NONE',  ( 181.0000000000000000, -164.9999999999999432, -344.0000000000001137 ) ) ;
#43351=DIRECTION ( 'NONE',  ( -1.586032880504786307E-16, 1.654361225106055350E-24, -1.000000000000000000 ) ) ;
#43352=FACE_OUTER_BOUND ( 'NONE', #30900, .T. ) ;
#43356=LINE ( 'NONE', #43610, #15509 ) ;
#43357=VERTEX_POINT ( 'NONE', #31041 ) ;
#43359=CARTESIAN_POINT ( 'NONE',  ( 185.0000000000000000, -164.9999999999999432, -356.0000000000001705 ) ) ;
#43362=VECTOR ( 'NONE', #31628, 1000.000000000000000 ) ;
#43365=CARTESIAN_POINT ( 'NONE',  ( 339.9999999999999432, -180.9999999999999716, -356.0000000000002274 ) ) ;
#43366=CIRCLE ( 'NONE', #8993, 2.000000000000001776 ) ;
#43368=CYLINDRICAL_SURFACE ( 'NONE', #21226, 4.000000000000003553 ) ;
#43376=CARTESIAN_POINT ( 'NONE',  ( 169.0000000000000000, 2.775557561562891351E-14, -113.0000000000001563 ) ) ;
#43381=LINE ( 'NONE', #20796, #16536 ) ;
#43382=EDGE_CURVE ( 'NONE', #35493, #7132, #34639, .T. ) ;
#43383=PRODUCT ( 'frame_Default<As Machined>', 'frame_Default<As Machined>', '', ( #1809 ) ) ;
#43385=DIRECTION ( 'NONE',  ( -0.000000000000000000, 3.186989995019654210E-49, 1.000000000000000000 ) ) ;
#43386=ADVANCED_FACE ( 'NONE', ( #11282 ), #27186, .F. ) ;
#43407=DIRECTION ( 'NONE',  ( 1.000000000000000000, 0.000000000000000000, 0.000000000000000000 ) ) ;
#43411=ORIENTED_EDGE ( 'NONE', *, *, #45252, .T. ) ;
#43412=EDGE_CURVE ( 'NONE', #12301, #4003, #25534, .T. ) ;
#43423=VERTEX_POINT ( 'NONE', #13761 ) ;
#43438=CARTESIAN_POINT ( 'NONE',  ( 357.1715728752537871, 167.0000000000001990, -342.0000000000002842 ) ) ;
#43439=CIRCLE ( 'NONE', #47515, 3.749999999999975575 ) ;
#43440=ORIENTED_EDGE ( 'NONE', *, *, #3053, .T. ) ;
#43441=EDGE_CURVE ( 'NONE', #46863, #18038, #18155, .T. ) ;
#43443=VECTOR ( 'NONE', #1647, 1000.000000000000000 ) ;
#43445=CARTESIAN_POINT ( 'NONE',  ( 168.9999999999999716, -272.4999999999999432, -339.9999999999998863 ) ) ;
#43446=FACE_OUTER_BOUND ( 'NONE', #19554, .T. ) ;
#43450=EDGE_CURVE ( 'NONE', #14373, #17870, #2720, .T. ) ;
#43456=DIRECTION ( 'NONE',  ( 0.000000000000000000, 0.000000000000000000, 1.000000000000000000 ) ) ;
#43457=VECTOR ( 'NONE', #50189, 1000.000000000000000 ) ;
#43458=( GEOMETRIC_REPRESENTATION_CONTEXT ( 3 ) GLOBAL_UNCERTAINTY_ASSIGNED_CONTEXT ( ( #6056 ) ) GLOBAL_UNIT_ASSIGNED_CONTEXT ( ( #3542, #19455, #15107 ) ) REPRESENTATION_CONTEXT ( 'NONE', 'WORKASPACE' ) );
#43462=FACE_OUTER_BOUND ( 'NONE', #18400, .T. ) ;
#43464=EDGE_CURVE ( 'NONE', #6873, #10796, #129, .T. ) ;
#43470=CARTESIAN_POINT ( 'NONE',  ( 339.9999999999999432, 181.0000000000000284, -360.0000000000002274 ) ) ;
#43471=CARTESIAN_POINT ( 'NONE',  ( 349.9999999999999432, -182.9999999999999716, 355.9999999999997726 ) ) ;
#43472=ORIENTED_EDGE ( 'NONE', *, *, #10456, .T. ) ;
#43473=ORIENTED_EDGE ( 'NONE', *, *, #16861, .F. ) ;
#43474=LINE ( 'NONE', #4481, #20956 ) ;
#43476=AXIS2_PLACEMENT_3D ( 'NONE', #13498, #25308, #41963 ) ;
#43478=AXIS2_PLACEMENT_3D ( 'NONE', #35488, #35753, #19549 ) ;
#43479=EDGE_CURVE ( 'NONE', #13504, #37058, #45548, .T. ) ;
#43482=DIRECTION ( 'NONE',  ( -1.586032892321652236E-16, -1.000000000000000000, -6.853681917100419162E-49 ) ) ;
#43484=DIRECTION ( 'NONE',  ( 1.333906992743555050E-23, -1.000000000000000000, 0.000000000000000000 ) ) ;
#43487=ORIENTED_EDGE ( 'NONE', *, *, #29891, .T. ) ;
#43489=ADVANCED_FACE ( 'NONE', ( #18363 ), #34045, .T. ) ;
#43490=VECTOR ( 'NONE', #32818, 1000.000000000000000 ) ;
#43491=EDGE_CURVE ( 'NONE', #30540, #750, #13511, .T. ) ;
#43495=ORIENTED_EDGE ( 'NONE', *, *, #15770, .T. ) ;
#43513=CARTESIAN_POINT ( 'NONE',  ( 344.0000000000000000, -167.0000000000001137, -342.0000000000002842 ) ) ;
#43518=CARTESIAN_POINT ( 'NONE',  ( 181.0000000000000568, 175.0000000000000284, 341.9999999999998863 ) ) ;
#43525=ORIENTED_EDGE ( 'NONE', *, *, #1171, .F. ) ;
#43538=EDGE_CURVE ( 'NONE', #25566, #25084, #45731, .T. ) ;
#43539=ORIENTED_EDGE ( 'NONE', *, *, #4469, .T. ) ;
#43545=EDGE_CURVE ( 'NONE', #14195, #43608, #15481, .T. ) ;
#43546=LINE ( 'NONE', #8417, #8775 ) ;
#43548=DIRECTION ( 'NONE',  ( 3.364279341222519273E-16, -0.7071067811865474617, 0.7071067811865476838 ) ) ;
#43560=EDGE_CURVE ( 'NONE', #43960, #34142, #38087, .T. ) ;
#43568=CARTESIAN_POINT ( 'NONE',  ( 357.9999999999999432, -180.9999999999999716, 355.9999999999998295 ) ) ;
#43570=FACE_BOUND ( 'NONE', #9361, .T. ) ;
#43572=( NAMED_UNIT ( * ) SI_UNIT ( $, .STERADIAN. ) SOLID_ANGLE_UNIT ( ) );
#43578=LINE ( 'NONE', #36872, #39620 ) ;
#43581=ADVANCED_FACE ( 'NONE', ( #42665 ), #23177, .T. ) ;
#43583=CARTESIAN_POINT ( 'NONE',  ( 181.0000000000000568, 165.0000000000000000, 339.9999999999997726 ) ) ;
#43598=DIRECTION ( 'NONE',  ( 0.000000000000000000, 1.000000000000000000, 0.000000000000000000 ) ) ;
#43608=VERTEX_POINT ( 'NONE', #27290 ) ;
#43610=CARTESIAN_POINT ( 'NONE',  ( 339.9999999999999432, -165.0000000000001137, -349.9999999999998863 ) ) ;
#43611=AXIS2_PLACEMENT_3D ( 'NONE', #28372, #25522, #5010 ) ;
#43621=AXIS2_PLACEMENT_3D ( 'NONE', #19763, #31329, #47671 ) ;
#43623=LINE ( 'NONE', #1552, #43339 ) ;
#43624=LINE ( 'NONE', #11839, #32468 ) ;
#43627=ORIENTED_EDGE ( 'NONE', *, *, #3439, .F. ) ;
#43629=FACE_OUTER_BOUND ( 'NONE', #31851, .T. ) ;
#43640=DIRECTION ( 'NONE',  ( 3.172065745548403743E-16, 1.000000000000000000, 0.000000000000000000 ) ) ;
#43644=FACE_OUTER_BOUND ( 'NONE', #100, .T. ) ;
#43654=ORIENTED_EDGE ( 'NONE', *, *, #13, .F. ) ;
#43656=DIRECTION ( 'NONE',  ( 0.000000000000000000, 1.000000000000000000, 6.123233995736766036E-17 ) ) ;
#43662=ORIENTED_EDGE ( 'NONE', *, *, #38628, .T. ) ;
#43666=ORIENTED_EDGE ( 'NONE', *, *, #28513, .T. ) ;
#43668=EDGE_CURVE ( 'NONE', #16142, #5465, #39602, .T. ) ;
#43669=EDGE_CURVE ( 'NONE', #34532, #6290, #31910, .T. ) ;
#43677=DIRECTION ( 'NONE',  ( -1.000000000000000000, 0.000000000000000000, 0.000000000000000000 ) ) ;
#43679=EDGE_CURVE ( 'NONE', #4741, #16142, #28295, .T. ) ;
#43680=CARTESIAN_POINT ( 'NONE',  ( 164.9999999999999716, 175.0000000000000284, -340.0000000000001137 ) ) ;
#43681=ADVANCED_FACE ( 'NONE', ( #16244 ), #47502, .F. ) ;
#43697=VERTEX_POINT ( 'NONE', #35254 ) ;
#43699=CARTESIAN_POINT ( 'NONE',  ( 350.0000000000000000, -180.9999999999999716, -340.0000000000001705 ) ) ;
#43708=VECTOR ( 'NONE', #16509, 1000.000000000000000 ) ;
#43713=LINE ( 'NONE', #35540, #46671 ) ;
#43720=DIRECTION ( 'NONE',  ( 0.000000000000000000, 1.000000000000000000, -2.537652627714643577E-15 ) ) ;
#43723=VERTEX_POINT ( 'NONE', #12145 ) ;
#43727=VECTOR ( 'NONE', #47383, 1000.000000000000000 ) ;
#43736=ORIENTED_EDGE ( 'NONE', *, *, #41920, .F. ) ;
#43737=ORIENTED_EDGE ( 'NONE', *, *, #17196, .T. ) ;
#43743=VECTOR ( 'NONE', #49395, 1000.000000000000000 ) ;
#43744=CARTESIAN_POINT ( 'NONE',  ( 4.999999999999999112, 175.0000000000000284, -353.7500000000001705 ) ) ;
#43745=ORIENTED_EDGE ( 'NONE', *, *, #4642, .F. ) ;
#43747=DIRECTION ( 'NONE',  ( -1.000000000000000000, 0.000000000000000000, 1.860490536778032451E-50 ) ) ;
#43753=LINE ( 'NONE', #39675, #49317 ) ;
#43776=EDGE_CURVE ( 'NONE', #31636, #29723, #17254, .T. ) ;
#43780=CARTESIAN_POINT ( 'NONE',  ( 166.9999999999999716, 6.000000000000060396, -350.0000000000001705 ) ) ;
#43785=ORIENTED_EDGE ( 'NONE', *, *, #44013, .T. ) ;
#43788=CARTESIAN_POINT ( 'NONE',  ( 342.0000000000000000, 165.0000000000000000, -94.00000000000019895 ) ) ;
#43799=CARTESIAN_POINT ( 'NONE',  ( 167.0000000000000000, -174.9999999999999716, -99.00000000000014211 ) ) ;
#43803=CARTESIAN_POINT ( 'NONE',  ( 168.9999999999999716, -164.9999999999999432, -340.0000000000001137 ) ) ;
#43804=EDGE_LOOP ( 'NONE', ( #8396, #1411, #39394, #42711 ) ) ;
#43809=FACE_OUTER_BOUND ( 'NONE', #5980, .T. ) ;
#43819=CIRCLE ( 'NONE', #21693, 4.000000000000003553 ) ;
#43823=CARTESIAN_POINT ( 'NONE',  ( 341.9999999999999432, 171.9999999999999432, -347.0000000000000568 ) ) ;
#43828=VERTEX_POINT ( 'NONE', #14406 ) ;
#43832=CARTESIAN_POINT ( 'NONE',  ( 349.9999999999999432, -164.9999999999999432, 343.9999999999997726 ) ) ;
#43834=CARTESIAN_POINT ( 'NONE',  ( 5.551115123125782702E-14, -180.9999999999999716, 357.9999999999997726 ) ) ;
#43835=ADVANCED_FACE ( 'NONE', ( #22612, #50259 ), #45926, .T. ) ;
#43841=ORIENTED_EDGE ( 'NONE', *, *, #23991, .T. ) ;
#43848=DIRECTION ( 'NONE',  ( -3.172065784643302499E-16, -1.000000000000000000, 2.537652627714642000E-15 ) ) ;
#43861=ORIENTED_EDGE ( 'NONE', *, *, #16208, .F. ) ;
#43869=LINE ( 'NONE', #5120, #44211 ) ;
#43873=VECTOR ( 'NONE', #28936, 1000.000000000000000 ) ;
#43878=LINE ( 'NONE', #12325, #28832 ) ;
#43887=DIRECTION ( 'NONE',  ( -1.000000000000000000, 0.000000000000000000, 0.000000000000000000 ) ) ;
#43889=DIRECTION ( 'NONE',  ( -1.000000000000000000, 0.000000000000000000, 0.000000000000000000 ) ) ;
#43890=VECTOR ( 'NONE', #28360, 1000.000000000000000 ) ;
#43892=ORIENTED_EDGE ( 'NONE', *, *, #17121, .F. ) ;
#43898=ORIENTED_EDGE ( 'NONE', *, *, #17978, .F. ) ;
#43900=ORIENTED_EDGE ( 'NONE', *, *, #40948, .F. ) ;
#43907=DIRECTION ( 'NONE',  ( 1.000000000000000000, 0.000000000000000000, -1.860490536778032451E-50 ) ) ;
#43909=VECTOR ( 'NONE', #5806, 1000.000000000000000 ) ;
#43914=CARTESIAN_POINT ( 'NONE',  ( 358.0000000000001137, 181.0000000000000284, 349.9999999999998295 ) ) ;
#43920=VECTOR ( 'NONE', #42082, 1000.000000000000000 ) ;
#43923=DIRECTION ( 'NONE',  ( 1.132880637372608740E-16, 4.718402560806925739E-50, 1.000000000000000000 ) ) ;
#43924=DIRECTION ( 'NONE',  ( 0.000000000000000000, -1.000000000000000000, 0.000000000000000000 ) ) ;
#43925=DIRECTION ( 'NONE',  ( 3.172065745548403743E-16, 1.000000000000000000, 0.000000000000000000 ) ) ;
#43926=VECTOR ( 'NONE', #13765, 1000.000000000000000 ) ;
#43932=CARTESIAN_POINT ( 'NONE',  ( 339.9999999999998863, -168.9999999999999432, 341.9999999999997726 ) ) ;
#43933=DIRECTION ( 'NONE',  ( -2.874857526315639190E-31, 1.000000000000000000, -2.537652627714642000E-15 ) ) ;
#43937=MECHANICAL_DESIGN_GEOMETRIC_PRESENTATION_REPRESENTATION('',(#6273),#26740);
#43941=CARTESIAN_POINT ( 'NONE',  ( 350.0000000000000000, -164.9999999999999432, -340.0000000000001705 ) ) ;
#43944=VERTEX_POINT ( 'NONE', #14916 ) ;
#43945=VECTOR ( 'NONE', #22338, 1000.000000000000000 ) ;
#43949=PLANE ( 'NONE',  #3895 ) ;
#43954=VERTEX_POINT ( 'NONE', #15171 ) ;
#43958=CARTESIAN_POINT ( 'NONE',  ( 164.9999999999999716, -9.999999999999953815, -111.0000000000001563 ) ) ;
#43959=VECTOR ( 'NONE', #41726, 1000.000000000000000 ) ;
#43960=VERTEX_POINT ( 'NONE', #42605 ) ;
#43961=DIRECTION ( 'NONE',  ( 1.000000000000000000, 0.000000000000000000, 0.000000000000000000 ) ) ;
#43962=VERTEX_POINT ( 'NONE', #22108 ) ;
#43964=LINE ( 'NONE', #20631, #44348 ) ;
#43965=EDGE_LOOP ( 'NONE', ( #3232, #11379, #5175, #41863 ) ) ;
#43967=CARTESIAN_POINT ( 'NONE',  ( 355.9999999999999432, -183.0000000000001137, -358.0000000000003411 ) ) ;
#43973=DIRECTION ( 'NONE',  ( 0.000000000000000000, 0.000000000000000000, 1.000000000000000000 ) ) ;
#43977=ORIENTED_EDGE ( 'NONE', *, *, #19975, .T. ) ;
#43979=DIRECTION ( 'NONE',  ( -1.586032892321652236E-16, -1.000000000000000000, -0.000000000000000000 ) ) ;
#43980=FACE_OUTER_BOUND ( 'NONE', #5151, .T. ) ;
#43989=EDGE_CURVE ( 'NONE', #18739, #7906, #2624, .T. ) ;
#43991=AXIS2_PLACEMENT_3D ( 'NONE', #24838, #20468, #1493 ) ;
#44000=CARTESIAN_POINT ( 'NONE',  ( 358.0000000000001137, 178.0000000000000284, 352.9999999999998295 ) ) ;
#44003=CARTESIAN_POINT ( 'NONE',  ( 344.0000000000000000, -174.9999999999999432, 339.9999999999998295 ) ) ;
#44007=DIRECTION ( 'NONE',  ( 0.000000000000000000, -1.000000000000000000, 0.000000000000000000 ) ) ;
#44011=EDGE_CURVE ( 'NONE', #7115, #40366, #23107, .T. ) ;
#44013=EDGE_CURVE ( 'NONE', #20947, #23039, #16438, .T. ) ;
#44015=CARTESIAN_POINT ( 'NONE',  ( 350.0000000000000000, -168.9999999999999432, -358.0000000000002274 ) ) ;
#44016=ADVANCED_FACE ( 'NONE', ( #790 ), #15673, .F. ) ;
#44017=PLANE ( 'NONE',  #33230 ) ;
#44019=EDGE_CURVE ( 'NONE', #21569, #1107, #8496, .T. ) ;
#44035=DIRECTION ( 'NONE',  ( 0.000000000000000000, 1.000000000000000000, -2.537652627714643577E-15 ) ) ;
#44038=ORIENTED_EDGE ( 'NONE', *, *, #37137, .T. ) ;
#44041=ORIENTED_EDGE ( 'NONE', *, *, #48428, .T. ) ;
#44044=DIRECTION ( 'NONE',  ( -4.758098676964957447E-16, -1.000000000000000000, 7.143884938411937192E-48 ) ) ;
#44046=EDGE_CURVE ( 'NONE', #21569, #47711, #43878, .T. ) ;
#44049=LINE ( 'NONE', #44796, #48026 ) ;
#44050=CARTESIAN_POINT ( 'NONE',  ( 350.0000000000001137, 181.0000000000000284, 339.9999999999997726 ) ) ;
#44053=ORIENTED_EDGE ( 'NONE', *, *, #48069, .T. ) ;
#44055=EDGE_CURVE ( 'NONE', #34812, #34800, #23627, .T. ) ;
#44060=DIRECTION ( 'NONE',  ( 0.000000000000000000, -2.537652627714643577E-15, -1.000000000000000000 ) ) ;
#44071=UNCERTAINTY_MEASURE_WITH_UNIT (LENGTH_MEASURE( 1.000000000000000082E-05 ), #19723, 'distance_accuracy_value', 'NONE');
#44074=DIRECTION ( 'NONE',  ( 0.000000000000000000, 2.537652627714642000E-15, 1.000000000000000000 ) ) ;
#44076=CARTESIAN_POINT ( 'NONE',  ( 181.0000000000000284, -168.9999999999999432, -115.0000000000001847 ) ) ;
#44080=CARTESIAN_POINT ( 'NONE',  ( 167.0000000000000000, -174.9999999999999716, -99.00000000000014211 ) ) ;
#44085=DIRECTION ( 'NONE',  ( -1.000000000000000000, 0.000000000000000000, -7.793956916774525800E-48 ) ) ;
#44086=ADVANCED_FACE ( 'NONE', ( #20535 ), #23884, .F. ) ;
#44098=LINE ( 'NONE', #33091, #48797 ) ;
#44099=CYLINDRICAL_SURFACE ( 'NONE', #33809, 2.000000000000001776 ) ;
#44110=EDGE_CURVE ( 'NONE', #21871, #13960, #44861, .T. ) ;
#44111=DIRECTION ( 'NONE',  ( 0.000000000000000000, -1.000000000000000000, 5.664403186863042467E-17 ) ) ;
#44114=DIRECTION ( 'NONE',  ( -1.586032880504786307E-16, 1.654361225106055350E-24, -1.000000000000000000 ) ) ;
#44123=EDGE_CURVE ( 'NONE', #7917, #6960, #9237, .T. ) ;
#44128=AXIS2_PLACEMENT_3D ( 'NONE', #1933, #21416, #13471 ) ;
#44129=CARTESIAN_POINT ( 'NONE',  ( 355.9999999999998863, -165.0000000000001137, -90.00000000000018474 ) ) ;
#44138=( BOUNDED_CURVE ( )  B_SPLINE_CURVE ( 3, ( #25936, #17465, #33140, #49223 ),
 .UNSPECIFIED., .F., .F. ) 
 B_SPLINE_CURVE_WITH_KNOTS ( ( 4, 4 ),
 ( 1.570796326794889675, 3.141592653589793116 ),
 .UNSPECIFIED. ) 
 CURVE ( )  GEOMETRIC_REPRESENTATION_ITEM ( )  RATIONAL_B_SPLINE_CURVE ( ( 1.000000000000000000, 0.8047378541243634942, 0.8047378541243634942, 1.000000000000000000 ) ) 
 REPRESENTATION_ITEM ( '' )  );
#44139=CARTESIAN_POINT ( 'NONE',  ( 358.3431457505076310, -165.0000000000001137, -340.0000000000003979 ) ) ;
#44146=FACE_OUTER_BOUND ( 'NONE', #26634, .T. ) ;
#44147=EDGE_LOOP ( 'NONE', ( #26793, #30003, #13542, #20722 ) ) ;
#44148=CARTESIAN_POINT ( 'NONE',  ( 185.0000000000000284, -174.9999999999999716, -111.0000000000001563 ) ) ;
#44151=FACE_OUTER_BOUND ( 'NONE', #46419, .T. ) ;
#44152=ORIENTED_EDGE ( 'NONE', *, *, #46638, .F. ) ;
#44161=ORIENTED_EDGE ( 'NONE', *, *, #43545, .T. ) ;
#44164=VECTOR ( 'NONE', #24794, 1000.000000000000000 ) ;
#44168=ADVANCED_FACE ( 'NONE', ( #28989 ), #36977, .T. ) ;
#44169=CARTESIAN_POINT ( 'NONE',  ( 356.0000000000000000, -167.0000000000001137, 341.9999999999999432 ) ) ;
#44174=VECTOR ( 'NONE', #27476, 1000.000000000000000 ) ;
#44175=LINE ( 'NONE', #12883, #2161 ) ;
#44176=CARTESIAN_POINT ( 'NONE',  ( 358.0000000000001137, 169.0000000000000000, 343.9999999999998863 ) ) ;
#44181=CARTESIAN_POINT ( 'NONE',  ( 358.0000000000000000, -174.9999999999999432, 343.9999999999998295 ) ) ;
#44182=ORIENTED_EDGE ( 'NONE', *, *, #17336, .F. ) ;
#44188=CARTESIAN_POINT ( 'NONE',  ( 358.0000000000000000, 167.8284271247463550, -342.8284271247465540 ) ) ;
#44194=FACE_BOUND ( 'NONE', #13131, .T. ) ;
#44197=DIRECTION ( 'NONE',  ( 0.000000000000000000, -1.000000000000000000, 0.000000000000000000 ) ) ;
#44200=CARTESIAN_POINT ( 'NONE',  ( 343.9999999999999432, 174.9999999999996589, -358.0000000000003411 ) ) ;
#44201=LINE ( 'NONE', #9078, #34019 ) ;
#44202=AXIS2_PLACEMENT_3D ( 'NONE', #40522, #21019, #48418 ) ;
#44211=VECTOR ( 'NONE', #48686, 1000.000000000000000 ) ;
#44225=EDGE_LOOP ( 'NONE', ( #22501, #46827, #44719, #4787 ) ) ;
#44226=DIRECTION ( 'NONE',  ( 0.000000000000000000, 1.000000000000000000, 0.000000000000000000 ) ) ;
#44227=DIRECTION ( 'NONE',  ( 0.000000000000000000, -1.000000000000000000, 0.000000000000000000 ) ) ;
#44229=DIRECTION ( 'NONE',  ( 0.000000000000000000, 5.664403186863042467E-17, 1.000000000000000000 ) ) ;
#44235=VECTOR ( 'NONE', #32190, 1000.000000000000000 ) ;
#44239=VERTEX_POINT ( 'NONE', #42305 ) ;
#44241=VECTOR ( 'NONE', #11446, 1000.000000000000000 ) ;
#44253=CARTESIAN_POINT ( 'NONE',  ( 181.0000000000000284, -174.9999999999999716, -95.00000000000014211 ) ) ;
#44257=DIRECTION ( 'NONE',  ( -1.000000000000000000, 0.000000000000000000, 1.860490536778032451E-50 ) ) ;
#44276=VERTEX_POINT ( 'NONE', #26906 ) ;
#44280=LINE ( 'NONE', #25068, #19671 ) ;
#44283=VERTEX_POINT ( 'NONE', #45621 ) ;
#44287=CYLINDRICAL_SURFACE ( 'NONE', #8612, 4.000000000000003553 ) ;
#44288=CARTESIAN_POINT ( 'NONE',  ( 181.0000000000000000, -164.9999999999999432, -360.0000000000002274 ) ) ;
#44291=EDGE_CURVE ( 'NONE', #13960, #28737, #3544, .T. ) ;
#44294=ORIENTED_EDGE ( 'NONE', *, *, #21343, .T. ) ;
#44299=CARTESIAN_POINT ( 'NONE',  ( 0.000000000000000000, -164.9999999999999432, -344.0000000000001705 ) ) ;
#44300=VERTEX_POINT ( 'NONE', #30257 ) ;
#44315=CARTESIAN_POINT ( 'NONE',  ( 360.0000000000001137, 181.0000000000000284, 349.9999999999998295 ) ) ;
#44320=DIRECTION ( 'NONE',  ( -1.000000000000000000, 0.000000000000000000, 0.000000000000000000 ) ) ;
#44333=CARTESIAN_POINT ( 'NONE',  ( 164.9999999999999716, -256.5000000000000000, -114.9999999999999432 ) ) ;
#44337=ORIENTED_EDGE ( 'NONE', *, *, #36982, .F. ) ;
#44348=VECTOR ( 'NONE', #39898, 1000.000000000000000 ) ;
#44350=EDGE_CURVE ( 'NONE', #2419, #39109, #3435, .T. ) ;
#44354=EDGE_LOOP ( 'NONE', ( #22518, #39471, #10920, #4035 ) ) ;
#44371=CARTESIAN_POINT ( 'NONE',  ( 168.9999999999998579, -184.9999999999999716, -340.0000000000001137 ) ) ;
#44375=VERTEX_POINT ( 'NONE', #23828 ) ;
#44376=CARTESIAN_POINT ( 'NONE',  ( 165.0000000000000000, 2.775557561562891351E-14, -115.0000000000001563 ) ) ;
#44377=DIRECTION ( 'NONE',  ( 0.000000000000000000, 1.000000000000000000, 0.000000000000000000 ) ) ;
#44378=VECTOR ( 'NONE', #36035, 1000.000000000000000 ) ;
#44390=EDGE_CURVE ( 'NONE', #55, #33080, #2420, .T. ) ;
#44393=ORIENTED_EDGE ( 'NONE', *, *, #22169, .F. ) ;
#44400=EDGE_CURVE ( 'NONE', #24759, #34532, #13513, .T. ) ;
#44401=LINE ( 'NONE', #35992, #22028 ) ;
#44404=CARTESIAN_POINT ( 'NONE',  ( 344.0000000000000000, -165.0000000000001137, -340.0000000000002842 ) ) ;
#44407=CARTESIAN_POINT ( 'NONE',  ( 358.0000000000000000, -169.0000000000001137, 344.0000000000000000 ) ) ;
#44410=ORIENTED_EDGE ( 'NONE', *, *, #18171, .T. ) ;
#44413=ADVANCED_FACE ( 'NONE', ( #10118 ), #28677, .F. ) ;
#44436=ORIENTED_EDGE ( 'NONE', *, *, #33705, .T. ) ;
#44442=LINE ( 'NONE', #13670, #25657 ) ;
#44449=CARTESIAN_POINT ( 'NONE',  ( -5.000000000000000000, -175.0000000000000284, 346.2500000000002274 ) ) ;
#44453=CARTESIAN_POINT ( 'NONE',  ( 168.9999999999999716, -79.49999999999997158, -350.0000000000001705 ) ) ;
#44471=EDGE_LOOP ( 'NONE', ( #47409, #48469, #44724, #46492 ) ) ;
#44490=EDGE_LOOP ( 'NONE', ( #16119, #49128, #13503, #31116 ) ) ;
#44506=CIRCLE ( 'NONE', #25714, 2.000000000000001776 ) ;
#44507=DIRECTION ( 'NONE',  ( -0.000000000000000000, -0.000000000000000000, 1.000000000000000000 ) ) ;
#44512=ORIENTED_EDGE ( 'NONE', *, *, #43464, .F. ) ;
#44516=EDGE_CURVE ( 'NONE', #16304, #46031, #24582, .T. ) ;
#44518=CYLINDRICAL_SURFACE ( 'NONE', #20086, 2.000000000000001776 ) ;
#44527=LINE ( 'NONE', #16606, #347 ) ;
#44535=ORIENTED_EDGE ( 'NONE', *, *, #8060, .F. ) ;
#44539=AXIS2_PLACEMENT_3D ( 'NONE', #9945, #2996, #15060 ) ;
#44554=VECTOR ( 'NONE', #48580, 1000.000000000000000 ) ;
#44557=DIRECTION ( 'NONE',  ( -1.000000000000000000, 0.000000000000000000, 0.000000000000000000 ) ) ;
#44559=LINE ( 'NONE', #9191, #50694 ) ;
#44570=FACE_OUTER_BOUND ( 'NONE', #47015, .T. ) ;
#44583=CARTESIAN_POINT ( 'NONE',  ( 342.0000000000000568, 167.8284271247462129, 342.8284271247459287 ) ) ;
#44587=CARTESIAN_POINT ( 'NONE',  ( 169.0000000000000000, -180.9999999999999716, -115.0000000000001279 ) ) ;
#44589=DIRECTION ( 'NONE',  ( -1.000000000000000000, 0.000000000000000000, 1.860490536778032451E-50 ) ) ;
#44591=VECTOR ( 'NONE', #39127, 1000.000000000000000 ) ;
#44601=ADVANCED_FACE ( 'NONE', ( #19337 ), #3162, .F. ) ;
#44609=ORIENTED_EDGE ( 'NONE', *, *, #23584, .F. ) ;
#44612=LINE ( 'NONE', #9241, #2168 ) ;
#44620=CARTESIAN_POINT ( 'NONE',  ( 339.9999999999999432, -174.9999999999999432, 343.9999999999998295 ) ) ;
#44628=EDGE_CURVE ( 'NONE', #7447, #37534, #23140, .T. ) ;
#44629=DIRECTION ( 'NONE',  ( 1.333906992743555050E-23, -1.000000000000000000, 0.000000000000000000 ) ) ;
#44634=ORIENTED_EDGE ( 'NONE', *, *, #24300, .F. ) ;
#44636=DIRECTION ( 'NONE',  ( -1.000000000000000000, 0.000000000000000000, 0.000000000000000000 ) ) ;
#44637=AXIS2_PLACEMENT_3D ( 'NONE', #43832, #4824, #28200 ) ;
#44641=CARTESIAN_POINT ( 'NONE',  ( 340.0000000000000568, 167.0000000000000000, 355.9999999999997726 ) ) ;
#44649=CARTESIAN_POINT ( 'NONE',  ( 181.0000000000000000, -7.999999999999952038, 339.9999999999998295 ) ) ;
#44654=ORIENTED_EDGE ( 'NONE', *, *, #12308, .T. ) ;
#44661=ADVANCED_FACE ( 'NONE', ( #42929 ), #7808, .F. ) ;
#44666=CARTESIAN_POINT ( 'NONE',  ( 343.9999999999999432, -185.0000000000000284, 359.9999999999998295 ) ) ;
#44668=FACE_OUTER_BOUND ( 'NONE', #13098, .T. ) ;
#44676=VECTOR ( 'NONE', #22972, 1000.000000000000000 ) ;
#44677=DIRECTION ( 'NONE',  ( 0.000000000000000000, 0.000000000000000000, 1.000000000000000000 ) ) ;
#44680=CARTESIAN_POINT ( 'NONE',  ( 355.9999999999999432, -183.0000000000001421, -358.0000000000003411 ) ) ;
#44688=ORIENTED_EDGE ( 'NONE', *, *, #50355, .F. ) ;
#44703=ORIENTED_EDGE ( 'NONE', *, *, #40649, .T. ) ;
#44704=ADVANCED_FACE ( 'NONE', ( #23951 ), #24718, .F. ) ;
#44705=CARTESIAN_POINT ( 'NONE',  ( 165.0000000000000000, -93.50000000000005684, -115.0000000000001563 ) ) ;
#44707=CARTESIAN_POINT ( 'NONE',  ( 341.9999999999999432, -171.9999999999999147, 346.9999999999998295 ) ) ;
#44708=DIRECTION ( 'NONE',  ( -1.586032880504786307E-16, 1.654361225106055350E-24, -1.000000000000000000 ) ) ;
#44719=ORIENTED_EDGE ( 'NONE', *, *, #13274, .T. ) ;
#44724=ORIENTED_EDGE ( 'NONE', *, *, #4675, .F. ) ;
#44732=VERTEX_POINT ( 'NONE', #8562 ) ;
#44738=EDGE_CURVE ( 'NONE', #2035, #19349, #18749, .T. ) ;
#44740=VERTEX_POINT ( 'NONE', #19836 ) ;
#44741=ORIENTED_EDGE ( 'NONE', *, *, #16836, .F. ) ;
#44744=EDGE_CURVE ( 'NONE', #37129, #38973, #2723, .T. ) ;
#44754=DIRECTION ( 'NONE',  ( 0.000000000000000000, -2.265761274745217480E-16, 1.000000000000000000 ) ) ;
#44763=DIRECTION ( 'NONE',  ( -1.000000000000000000, -0.000000000000000000, -0.000000000000000000 ) ) ;
#44767=CARTESIAN_POINT ( 'NONE',  ( 164.9999999999999716, -164.9999999999999432, -356.0000000000001705 ) ) ;
#44770=VECTOR ( 'NONE', #7916, 1000.000000000000000 ) ;
#44771=EDGE_LOOP ( 'NONE', ( #39869, #23696, #32887, #18900 ) ) ;
#44772=PLANE ( 'NONE',  #27302 ) ;
#44776=DIRECTION ( 'NONE',  ( 0.000000000000000000, 0.000000000000000000, 1.000000000000000000 ) ) ;
#44779=ORIENTED_EDGE ( 'NONE', *, *, #31009, .F. ) ;
#44788=ORIENTED_EDGE ( 'NONE', *, *, #28012, .T. ) ;
#44796=CARTESIAN_POINT ( 'NONE',  ( 341.9999999999999432, 175.0000000000000284, -106.0000000000001990 ) ) ;
#44798=CARTESIAN_POINT ( 'NONE',  ( 0.000000000000000000, 181.0000000000000284, 339.9999999999997726 ) ) ;
#44805=ORIENTED_EDGE ( 'NONE', *, *, #8468, .F. ) ;
#44810=ADVANCED_FACE ( 'NONE', ( #14147 ), #22116, .T. ) ;
#44813=CYLINDRICAL_SURFACE ( 'NONE', #36416, 3.749999999999975575 ) ;
#44822=LINE ( 'NONE', #13537, #25362 ) ;
#44841=ORIENTED_EDGE ( 'NONE', *, *, #43479, .T. ) ;
#44842=CARTESIAN_POINT ( 'NONE',  ( 355.9999999999999432, 183.0000000000002558, -358.0000000000003411 ) ) ;
#44843=CARTESIAN_POINT ( 'NONE',  ( 339.9999999999999432, -180.9999999999999716, -344.0000000000001705 ) ) ;
#44844=DIRECTION ( 'NONE',  ( 1.132880637372608740E-16, 4.718402560806925739E-50, 1.000000000000000000 ) ) ;
#44845=CARTESIAN_POINT ( 'NONE',  ( 164.9999999999999716, -272.5000000000000000, -110.9999999999999005 ) ) ;
#44847=DIRECTION ( 'NONE',  ( 0.000000000000000000, 5.664403186863042467E-17, 1.000000000000000000 ) ) ;
#44849=VECTOR ( 'NONE', #1123, 1000.000000000000000 ) ;
#44850=LINE ( 'NONE', #36450, #43127 ) ;
#44851=PLANE ( 'NONE',  #7303 ) ;
#44852=ORIENTED_EDGE ( 'NONE', *, *, #15821, .T. ) ;
#44854=VERTEX_POINT ( 'NONE', #2600 ) ;
#44861=LINE ( 'NONE', #17928, #42757 ) ;
#44863=DIRECTION ( 'NONE',  ( 0.000000000000000000, 0.000000000000000000, -1.000000000000000000 ) ) ;
#44872=CARTESIAN_POINT ( 'NONE',  ( 339.9999999999999432, -166.9999999999999432, -356.0000000000002274 ) ) ;
#44880=DIRECTION ( 'NONE',  ( 0.000000000000000000, 0.000000000000000000, -1.000000000000000000 ) ) ;
#44881=DIRECTION ( 'NONE',  ( 0.000000000000000000, 0.000000000000000000, 1.000000000000000000 ) ) ;
#44882=EDGE_CURVE ( 'NONE', #27106, #30474, #25266, .T. ) ;
#44896=CARTESIAN_POINT ( 'NONE',  ( 341.6568542494924259, 165.0000000000000000, 339.9999999999998295 ) ) ;
#44900=ORIENTED_EDGE ( 'NONE', *, *, #7616, .F. ) ;
#44906=ORIENTED_EDGE ( 'NONE', *, *, #12856, .F. ) ;
#44909=ORIENTED_EDGE ( 'NONE', *, *, #21122, .T. ) ;
#44910=CARTESIAN_POINT ( 'NONE',  ( 167.0000000000000000, -174.9999999999999716, -111.0000000000001563 ) ) ;
#44911=CARTESIAN_POINT ( 'NONE',  ( 185.0000000000000000, -184.9999999999999716, -344.0000000000001137 ) ) ;
#44919=DIRECTION ( 'NONE',  ( 1.000000000000000000, 0.000000000000000000, 0.000000000000000000 ) ) ;
#44925=EDGE_LOOP ( 'NONE', ( #26617, #45066, #20852, #28753 ) ) ;
#44927=DIRECTION ( 'NONE',  ( -1.000000000000000000, 0.000000000000000000, -1.612977847700450206E-50 ) ) ;
#44932=CARTESIAN_POINT ( 'NONE',  ( 0.000000000000000000, -168.9999999999999432, -340.0000000000001705 ) ) ;
#44936=CARTESIAN_POINT ( 'NONE',  ( 181.0000000000000000, -272.5000000000000000, -94.99999999999988631 ) ) ;
#44944=CYLINDRICAL_SURFACE ( 'NONE', #19603, 4.000000000000003553 ) ;
#44945=EDGE_LOOP ( 'NONE', ( #12314, #12565, #40338, #23774 ) ) ;
#44953=EDGE_CURVE ( 'NONE', #3827, #19026, #36295, .T. ) ;
#44960=EDGE_CURVE ( 'NONE', #1207, #47828, #34438, .T. ) ;
#44962=EDGE_CURVE ( 'NONE', #8293, #50401, #2847, .T. ) ;
#44964=CIRCLE ( 'NONE', #3184, 2.000000000000001776 ) ;
#44967=CARTESIAN_POINT ( 'NONE',  ( 185.0000000000000000, -268.4999999999999432, -339.9999999999998863 ) ) ;
#44968=VECTOR ( 'NONE', #14573, 1000.000000000000000 ) ;
#44972=CARTESIAN_POINT ( 'NONE',  ( 183.0000000000000000, -268.4999999999999432, -349.9999999999999432 ) ) ;
#44974=CARTESIAN_POINT ( 'NONE',  ( -5.000000000000000000, 0.000000000000000000, 0.000000000000000000 ) ) ;
#44976=EDGE_LOOP ( 'NONE', ( #34561, #10683, #16215, #14397 ) ) ;
#44984=ORIENTED_EDGE ( 'NONE', *, *, #8618, .T. ) ;
#44986=LINE ( 'NONE', #18064, #1136 ) ;
#44989=FACE_OUTER_BOUND ( 'NONE', #27467, .T. ) ;
#44990=AXIS2_PLACEMENT_3D ( 'NONE', #27888, #4772, #49347 ) ;
#44997=DIRECTION ( 'NONE',  ( 1.000000000000000000, 0.000000000000000000, 0.000000000000000000 ) ) ;
#44999=VECTOR ( 'NONE', #27158, 1000.000000000000000 ) ;
#45008=DIRECTION ( 'NONE',  ( 0.000000000000000000, 1.000000000000000000, 0.000000000000000000 ) ) ;
#45013=( BOUNDED_CURVE ( )  B_SPLINE_CURVE ( 3, ( #36585, #9107, #12692, #24764 ),
 .UNSPECIFIED., .F., .F. ) 
 B_SPLINE_CURVE_WITH_KNOTS ( ( 4, 4 ),
 ( 0.000000000000000000, 1.570796326794889675 ),
 .UNSPECIFIED. ) 
 CURVE ( )  GEOMETRIC_REPRESENTATION_ITEM ( )  RATIONAL_B_SPLINE_CURVE ( ( 1.000000000000000000, 0.8047378541243667138, 0.8047378541243667138, 1.000000000000000000 ) ) 
 REPRESENTATION_ITEM ( '' )  );
#45015=EDGE_CURVE ( 'NONE', #34498, #38360, #5137, .T. ) ;
#45016=CARTESIAN_POINT ( 'NONE',  ( 340.0000000000000568, 181.0000000000000853, 355.9999999999998295 ) ) ;
#45019=( BOUNDED_CURVE ( )  B_SPLINE_CURVE ( 3, ( #3030, #18680, #14841, #27662 ),
 .UNSPECIFIED., .F., .F. ) 
 B_SPLINE_CURVE_WITH_KNOTS ( ( 4, 4 ),
 ( 3.140184917367548361E-16, 1.570796326794882791 ),
 .UNSPECIFIED. ) 
 CURVE ( )  GEOMETRIC_REPRESENTATION_ITEM ( )  RATIONAL_B_SPLINE_CURVE ( ( 1.000000000000000000, 0.8047378541243681571, 0.8047378541243681571, 1.000000000000000000 ) ) 
 REPRESENTATION_ITEM ( '' )  );
#45020=ADVANCED_FACE ( 'NONE', ( #36213 ), #558, .F. ) ;
#45022=DIRECTION ( 'NONE',  ( -3.172065784643302499E-16, -1.000000000000000000, 2.537652627714642000E-15 ) ) ;
#45023=ORIENTED_EDGE ( 'NONE', *, *, #45325, .F. ) ;
#45035=VERTEX_POINT ( 'NONE', #47196 ) ;
#45037=ORIENTED_EDGE ( 'NONE', *, *, #39685, .F. ) ;
#45042=AXIS2_PLACEMENT_3D ( 'NONE', #29347, #6493, #2392 ) ;
#45047=EDGE_LOOP ( 'NONE', ( #48321, #18432, #11952, #30218 ) ) ;
#45048=ORIENTED_EDGE ( 'NONE', *, *, #16201, .T. ) ;
#45065=CARTESIAN_POINT ( 'NONE',  ( -5.000000000000000000, 165.2000000000000171, 340.1999999999997044 ) ) ;
#45066=ORIENTED_EDGE ( 'NONE', *, *, #47160, .T. ) ;
#45069=MECHANICAL_DESIGN_GEOMETRIC_PRESENTATION_REPRESENTATION('',(#16428),#43458);
#45076=CARTESIAN_POINT ( 'NONE',  ( 349.9999999999999432, -164.9999999999999432, 343.9999999999997726 ) ) ;
#45078=LINE ( 'NONE', #9957, #33728 ) ;
#45080=CYLINDRICAL_SURFACE ( 'NONE', #37964, 4.000000000000003553 ) ;
#45085=ORIENTED_EDGE ( 'NONE', *, *, #8346, .F. ) ;
#45089=EDGE_CURVE ( 'NONE', #37129, #48972, #45372, .T. ) ;
#45098=ORIENTED_EDGE ( 'NONE', *, *, #17772, .T. ) ;
#45099=CARTESIAN_POINT ( 'NONE',  ( -5.000000000000000000, 165.2000000000000171, -359.8000000000002387 ) ) ;
#45102=ORIENTED_EDGE ( 'NONE', *, *, #14505, .F. ) ;
#45103=CARTESIAN_POINT ( 'NONE',  ( 181.0000000000000000, -174.9999999999999716, -356.0000000000001705 ) ) ;
#45108=CARTESIAN_POINT ( 'NONE',  ( 183.0000000000000000, -272.5000000000000000, -111.0000000000001563 ) ) ;
#45121=EDGE_CURVE ( 'NONE', #1398, #48718, #1554, .T. ) ;
#45122=EDGE_LOOP ( 'NONE', ( #27358, #43785, #1140, #5251 ) ) ;
#45132=DIRECTION ( 'NONE',  ( 0.000000000000000000, 0.000000000000000000, 1.000000000000000000 ) ) ;
#45135=CARTESIAN_POINT ( 'NONE',  ( 357.1715728752539576, 183.0000000000000284, 357.9999999999998295 ) ) ;
#45138=ORIENTED_EDGE ( 'NONE', *, *, #43669, .T. ) ;
#45141=AXIS2_PLACEMENT_3D ( 'NONE', #42509, #3253, #37939 ) ;
#45152=ORIENTED_EDGE ( 'NONE', *, *, #47785, .T. ) ;
#45156=ORIENTED_EDGE ( 'NONE', *, *, #43382, .F. ) ;
#45163=CARTESIAN_POINT ( 'NONE',  ( 340.0000000000001137, 166.6568542494924259, 341.6568542494921417 ) ) ;
#45170=AXIS2_PLACEMENT_3D ( 'NONE', #49334, #2680, #18318 ) ;
#45172=VERTEX_POINT ( 'NONE', #16955 ) ;
#45173=DIRECTION ( 'NONE',  ( 1.000000000000000000, 0.000000000000000000, -7.793956916774525800E-48 ) ) ;
#45177=CIRCLE ( 'NONE', #36224, 4.000000000000003553 ) ;
#45181=ORIENTED_EDGE ( 'NONE', *, *, #767, .T. ) ;
#45186=DIRECTION ( 'NONE',  ( 0.000000000000000000, -2.537652627714643577E-15, -1.000000000000000000 ) ) ;
#45192=DIRECTION ( 'NONE',  ( 1.000000000000000000, -5.326388832052271710E-25, 1.587271980518778491E-16 ) ) ;
#45196=DIRECTION ( 'NONE',  ( 0.000000000000000000, -1.000000000000000000, -3.186989995019654210E-49 ) ) ;
#45198=LINE ( 'NONE', #49031, #43016 ) ;
#45203=ORIENTED_EDGE ( 'NONE', *, *, #25993, .F. ) ;
#45209=ORIENTED_EDGE ( 'NONE', *, *, #6700, .F. ) ;
#45210=FACE_OUTER_BOUND ( 'NONE', #36116, .T. ) ;
#45215=EDGE_LOOP ( 'NONE', ( #26116, #15121, #45854, #46986 ) ) ;
#45221=CARTESIAN_POINT ( 'NONE',  ( 350.0000000000000000, 183.0000000000000284, -356.0000000000002274 ) ) ;
#45227=PLANE ( 'NONE',  #33924 ) ;
#45229=STYLED_ITEM('',(#50747),#5610);
#45235=DIRECTION ( 'NONE',  ( -0.000000000000000000, -1.000000000000000000, 2.537652627714643577E-15 ) ) ;
#45245=FACE_OUTER_BOUND ( 'NONE', #47939, .T. ) ;
#45248=VECTOR ( 'NONE', #44589, 1000.000000000000000 ) ;
#45252=EDGE_CURVE ( 'NONE', #42696, #34995, #14860, .T. ) ;
#45253=CARTESIAN_POINT ( 'NONE',  ( 339.9999999999998863, -180.9999999999999716, 357.9999999999997726 ) ) ;
#45257=CARTESIAN_POINT ( 'NONE',  ( 181.0000000000000284, -174.9999999999999716, -113.0000000000001563 ) ) ;
#45264=ORIENTED_EDGE ( 'NONE', *, *, #45999, .T. ) ;
#45273=AXIS2_PLACEMENT_3D ( 'NONE', #16632, #8187, #11778 ) ;
#45283=CYLINDRICAL_SURFACE ( 'NONE', #14268, 2.000000000000001776 ) ;
#45286=ORIENTED_EDGE ( 'NONE', *, *, #14596, .F. ) ;
#45288=LINE ( 'NONE', #10170, #26620 ) ;
#45292=CARTESIAN_POINT ( 'NONE',  ( 169.0000000000000000, 2.775557561562891351E-14, -111.0000000000001563 ) ) ;
#45304=LINE ( 'NONE', #37915, #28452 ) ;
#45307=CARTESIAN_POINT ( 'NONE',  ( 185.0000000000000000, -272.4999999999999432, -355.9999999999999432 ) ) ;
#45310=LINE ( 'NONE', #2493, #27521 ) ;
#45316=AXIS2_PLACEMENT_3D ( 'NONE', #39892, #8829, #35803 ) ;
#45325=EDGE_CURVE ( 'NONE', #25314, #13960, #28102, .T. ) ;
#45327=DIRECTION ( 'NONE',  ( 0.000000000000000000, 0.000000000000000000, 1.000000000000000000 ) ) ;
#45335=CARTESIAN_POINT ( 'NONE',  ( 360.0000000000000568, 169.0000000000000284, 343.9999999999998863 ) ) ;
#45337=CARTESIAN_POINT ( 'NONE',  ( 350.0000000000000000, -180.9999999999999716, -344.0000000000001705 ) ) ;
#45340=ORIENTED_EDGE ( 'NONE', *, *, #20861, .F. ) ;
#45349=AXIS2_PLACEMENT_3D ( 'NONE', #34895, #4081, #11276 ) ;
#45360=ORIENTED_EDGE ( 'NONE', *, *, #20861, .T. ) ;
#45361=DIRECTION ( 'NONE',  ( 1.860490536778032451E-50, 0.000000000000000000, -1.000000000000000000 ) ) ;
#45364=EDGE_CURVE ( 'NONE', #11132, #28586, #46913, .T. ) ;
#45369=CARTESIAN_POINT ( 'NONE',  ( 168.9999999999999716, -272.4999999999999432, -339.9999999999998863 ) ) ;
#45372=LINE ( 'NONE', #29755, #13325 ) ;
#45378=CIRCLE ( 'NONE', #12623, 2.000000000000001776 ) ;
#45381=EDGE_LOOP ( 'NONE', ( #5250, #43472, #8563, #19361, #27695, #28901, #44852, #3664 ) ) ;
#45384=DIRECTION ( 'NONE',  ( 1.000000000000000000, -4.758098676964957447E-16, 2.958228394578795584E-31 ) ) ;
#45386=DIRECTION ( 'NONE',  ( 0.000000000000000000, 0.000000000000000000, -1.000000000000000000 ) ) ;
#45389=DIRECTION ( 'NONE',  ( 9.711650524620651178E-33, -1.223873602809432483E-48, 1.000000000000000000 ) ) ;
#45390=VERTEX_POINT ( 'NONE', #42806 ) ;
#45398=ORIENTED_EDGE ( 'NONE', *, *, #27122, .T. ) ;
#45402=DIRECTION ( 'NONE',  ( 5.473822126268816076E-48, -1.000000000000000000, -1.654361225106055350E-24 ) ) ;
#45405=LINE ( 'NONE', #49236, #20492 ) ;
#45414=CARTESIAN_POINT ( 'NONE',  ( 357.9999999999999432, -181.0000000000000568, -356.0000000000002842 ) ) ;
#45423=VERTEX_POINT ( 'NONE', #36674 ) ;
#45425=CARTESIAN_POINT ( 'NONE',  ( 181.0000000000000000, -81.49999999999995737, -115.0000000000001563 ) ) ;
#45431=VERTEX_POINT ( 'NONE', #29441 ) ;
#45441=CARTESIAN_POINT ( 'NONE',  ( 0.000000000000000000, 169.0000000000000000, 355.9999999999997726 ) ) ;
#45446=CARTESIAN_POINT ( 'NONE',  ( 168.9999999999999716, 8.000000000000062172, -340.0000000000001137 ) ) ;
#45447=CIRCLE ( 'NONE', #12736, 4.000000000000003553 ) ;
#45450=VECTOR ( 'NONE', #34350, 1000.000000000000000 ) ;
#45452=EDGE_LOOP ( 'NONE', ( #43977, #29335, #37702, #10355 ) ) ;
#45460=ORIENTED_EDGE ( 'NONE', *, *, #10307, .F. ) ;
#45466=ORIENTED_EDGE ( 'NONE', *, *, #30867, .T. ) ;
#45473=DIRECTION ( 'NONE',  ( 0.000000000000000000, 0.000000000000000000, 1.000000000000000000 ) ) ;
#45475=DIRECTION ( 'NONE',  ( 0.000000000000000000, 0.000000000000000000, 1.000000000000000000 ) ) ;
#45477=ORIENTED_EDGE ( 'NONE', *, *, #39052, .F. ) ;
#45479=EDGE_LOOP ( 'NONE', ( #1007, #47936, #15607, #11117 ) ) ;
#45481=( BOUNDED_CURVE ( )  B_SPLINE_CURVE ( 3, ( #1368, #11900, #24465, #48007 ),
 .UNSPECIFIED., .F., .F. ) 
 B_SPLINE_CURVE_WITH_KNOTS ( ( 4, 4 ),
 ( 4.710277376051282359E-16, 1.570796326794896780 ),
 .UNSPECIFIED. ) 
 CURVE ( )  GEOMETRIC_REPRESENTATION_ITEM ( )  RATIONAL_B_SPLINE_CURVE ( ( 1.000000000000000000, 0.8047378541243650485, 0.8047378541243650485, 1.000000000000000000 ) ) 
 REPRESENTATION_ITEM ( '' )  );
#45486=AXIS2_PLACEMENT_3D ( 'NONE', #31923, #7813, #35026 ) ;
#45488=VECTOR ( 'NONE', #15367, 1000.000000000000000 ) ;
#45491=DIRECTION ( 'NONE',  ( 1.000000000000000000, 0.000000000000000000, 0.000000000000000000 ) ) ;
#45514=VECTOR ( 'NONE', #27287, 1000.000000000000000 ) ;
#45519=VECTOR ( 'NONE', #2134, 1000.000000000000000 ) ;
#45522=ORIENTED_EDGE ( 'NONE', *, *, #45121, .F. ) ;
#45529=EDGE_CURVE ( 'NONE', #9207, #10844, #6092, .T. ) ;
#45533=CARTESIAN_POINT ( 'NONE',  ( 181.0000000000000284, -272.5000000000000000, -96.99999999999988631 ) ) ;
#45537=LINE ( 'NONE', #22468, #28208 ) ;
#45545=EDGE_LOOP ( 'NONE', ( #10528, #40732, #9860, #3963 ) ) ;
#45548=LINE ( 'NONE', #10427, #3394 ) ;
#45551=ORIENTED_EDGE ( 'NONE', *, *, #5098, .F. ) ;
#45554=CARTESIAN_POINT ( 'NONE',  ( 341.9999999999999432, -180.9999999999999716, 355.9999999999998295 ) ) ;
#45564=AXIS2_PLACEMENT_3D ( 'NONE', #27984, #28248, #8755 ) ;
#45579=CARTESIAN_POINT ( 'NONE',  ( 181.0000000000000568, 175.0000000000000284, 343.9999999999998863 ) ) ;
#45588=CARTESIAN_POINT ( 'NONE',  ( 343.9999999999993747, 183.0000000000000568, 357.9999999999998295 ) ) ;
#45592=EDGE_CURVE ( 'NONE', #38490, #8483, #6595, .T. ) ;
#45595=DIRECTION ( 'NONE',  ( 0.000000000000000000, 0.000000000000000000, 1.000000000000000000 ) ) ;
#45610=ORIENTED_EDGE ( 'NONE', *, *, #13294, .T. ) ;
#45613=VERTEX_POINT ( 'NONE', #49888 ) ;
#45617=CARTESIAN_POINT ( 'NONE',  ( 341.9999999999999432, -181.0000000000001421, 356.0000000000000568 ) ) ;
#45618=ORIENTED_EDGE ( 'NONE', *, *, #296, .F. ) ;
#45621=CARTESIAN_POINT ( 'NONE',  ( -5.000000000000000000, -184.7999999999999545, -340.2000000000001592 ) ) ;
#45627=CARTESIAN_POINT ( 'NONE',  ( 5.551115123125782702E-14, -180.9999999999999716, 355.9999999999997726 ) ) ;
#45648=VERTEX_POINT ( 'NONE', #6346 ) ;
#45650=EDGE_LOOP ( 'NONE', ( #13279, #46206, #39910, #6357 ) ) ;
#45651=EDGE_CURVE ( 'NONE', #15590, #16798, #30194, .T. ) ;
#45653=EDGE_CURVE ( 'NONE', #44283, #1426, #26356, .T. ) ;
#45655=DIRECTION ( 'NONE',  ( 1.000000000000000000, 0.000000000000000000, 1.586032872232979935E-16 ) ) ;
#45689=CARTESIAN_POINT ( 'NONE',  ( 164.9999999999999716, 165.0000000000000000, -356.0000000000001705 ) ) ;
#45700=DIRECTION ( 'NONE',  ( 0.000000000000000000, -1.000000000000000000, -3.186989995019654210E-49 ) ) ;
#45701=ORIENTED_EDGE ( 'NONE', *, *, #49158, .F. ) ;
#45704=CARTESIAN_POINT ( 'NONE',  ( 168.9999999999999716, 10.00000000000006395, 339.9999999999998295 ) ) ;
#45708=CARTESIAN_POINT ( 'NONE',  ( 181.0000000000000000, 6.000000000000060396, -340.0000000000001137 ) ) ;
#45718=ADVANCED_FACE ( 'NONE', ( #12466 ), #30978, .F. ) ;
#45721=ORIENTED_EDGE ( 'NONE', *, *, #26476, .F. ) ;
#45731=LINE ( 'NONE', #15240, #34551 ) ;
#45737=EDGE_LOOP ( 'NONE', ( #9141, #31198, #34856, #6666 ) ) ;
#45740=DIRECTION ( 'NONE',  ( -1.000000000000000000, 0.000000000000000000, -2.958228394578794270E-31 ) ) ;
#45746=CARTESIAN_POINT ( 'NONE',  ( -5.000000000000000000, 184.8000000000000114, 359.7999999999997840 ) ) ;
#45747=ORIENTED_EDGE ( 'NONE', *, *, #4090, .T. ) ;
#45748=CARTESIAN_POINT ( 'NONE',  ( -5.000000000000000000, -175.0000000000000284, -350.0000000000002274 ) ) ;
#45752=LINE ( 'NONE', #3702, #14413 ) ;
#45754=VECTOR ( 'NONE', #18315, 1000.000000000000000 ) ;
#45758=CARTESIAN_POINT ( 'NONE',  ( 181.0000000000000000, -9.999999999999953815, -340.0000000000001137 ) ) ;
#45781=DIRECTION ( 'NONE',  ( 0.000000000000000000, 1.000000000000000000, 0.000000000000000000 ) ) ;
#45782=ORIENTED_EDGE ( 'NONE', *, *, #37641, .F. ) ;
#45796=DIRECTION ( 'NONE',  ( 0.000000000000000000, 1.000000000000000000, 6.123233995736766036E-17 ) ) ;
#45805=ORIENTED_EDGE ( 'NONE', *, *, #40011, .T. ) ;
#45808=DIRECTION ( 'NONE',  ( 0.000000000000000000, 1.000000000000000000, 0.000000000000000000 ) ) ;
#45810=LINE ( 'NONE', #19418, #11600 ) ;
#45815=FACE_BOUND ( 'NONE', #47263, .T. ) ;
#45818=DIRECTION ( 'NONE',  ( -1.000000000000000000, 0.000000000000000000, -7.793956916774525800E-48 ) ) ;
#45822=LINE ( 'NONE', #10215, #12348 ) ;
#45823=LINE ( 'NONE', #41516, #24036 ) ;
#45827=CARTESIAN_POINT ( 'NONE',  ( 185.0000000000000568, 165.0000000000000000, 343.9999999999998863 ) ) ;
#45832=EDGE_CURVE ( 'NONE', #25388, #31636, #46899, .T. ) ;
#45833=ORIENTED_EDGE ( 'NONE', *, *, #29028, .F. ) ;
#45844=CARTESIAN_POINT ( 'NONE',  ( 166.9999999999999716, 6.000000000000060396, -340.0000000000001137 ) ) ;
#45852=EDGE_CURVE ( 'NONE', #38055, #28373, #41175, .T. ) ;
#45854=ORIENTED_EDGE ( 'NONE', *, *, #7628, .F. ) ;
#45855=AXIS2_PLACEMENT_3D ( 'NONE', #43287, #47353, #42770 ) ;
#45876=ADVANCED_FACE ( 'NONE', ( #36868 ), #36351, .T. ) ;
#45880=EDGE_CURVE ( 'NONE', #48770, #4014, #9634, .T. ) ;
#45881=DIRECTION ( 'NONE',  ( 1.000000000000000000, 6.344131455081961406E-16, -4.759647537211363479E-16 ) ) ;
#45883=EDGE_CURVE ( 'NONE', #40029, #38840, #7665, .T. ) ;
#45887=EDGE_LOOP ( 'NONE', ( #471, #21217, #26977, #18979 ) ) ;
#45892=CARTESIAN_POINT ( 'NONE',  ( 181.0000000000000000, -95.49999999999997158, -115.0000000000001563 ) ) ;
#45898=AXIS2_PLACEMENT_3D ( 'NONE', #46972, #27528, #15971 ) ;
#45915=ORIENTED_EDGE ( 'NONE', *, *, #44960, .F. ) ;
#45925=LINE ( 'NONE', #10806, #15621 ) ;
#45926=PLANE ( 'NONE',  #48449 ) ;
#45928=ADVANCED_FACE ( 'NONE', ( #42435 ), #49587, .F. ) ;
#45936=CARTESIAN_POINT ( 'NONE',  ( -5.000000000000000000, 165.2000000000000171, -340.2000000000001592 ) ) ;
#45940=EDGE_CURVE ( 'NONE', #39919, #19835, #3174, .T. ) ;
#45946=FACE_OUTER_BOUND ( 'NONE', #4721, .T. ) ;
#45958=DIRECTION ( 'NONE',  ( 1.000000000000000000, 0.000000000000000000, -1.860490536778032451E-50 ) ) ;
#45959=LINE ( 'NONE', #48796, #32932 ) ;
#45965=CARTESIAN_POINT ( 'NONE',  ( 344.0000000000000000, 165.0000000000000000, -92.00000000000019895 ) ) ;
#45967=VECTOR ( 'NONE', #606, 1000.000000000000000 ) ;
#45971=CARTESIAN_POINT ( 'NONE',  ( 167.0000000000000000, -174.9999999999999716, -99.00000000000014211 ) ) ;
#45973=VERTEX_POINT ( 'NONE', #45253 ) ;
#45974=LINE ( 'NONE', #18795, #29042 ) ;
#45977=ORIENTED_EDGE ( 'NONE', *, *, #49753, .F. ) ;
#45978=DIRECTION ( 'NONE',  ( 0.000000000000000000, -2.537652627714642000E-15, -1.000000000000000000 ) ) ;
#45981=VECTOR ( 'NONE', #32444, 1000.000000000000000 ) ;
#45993=( NAMED_UNIT ( * ) SI_UNIT ( $, .STERADIAN. ) SOLID_ANGLE_UNIT ( ) );
#45995=FACE_BOUND ( 'NONE', #12620, .T. ) ;
#45998=CARTESIAN_POINT ( 'NONE',  ( 185.0000000000000000, 6.000000000000060396, -350.0000000000001705 ) ) ;
#45999=EDGE_CURVE ( 'NONE', #49298, #22581, #35515, .T. ) ;
#46009=FACE_OUTER_BOUND ( 'NONE', #5515, .T. ) ;
#46012=DIRECTION ( 'NONE',  ( 0.000000000000000000, -2.265761274745217480E-16, 1.000000000000000000 ) ) ;
#46015=CARTESIAN_POINT ( 'NONE',  ( 169.0000000000000000, -174.9999999999999716, -99.00000000000014211 ) ) ;
#46016=ORIENTED_EDGE ( 'NONE', *, *, #12928, .T. ) ;
#46017=DIRECTION ( 'NONE',  ( 7.793956916774525800E-48, 0.000000000000000000, 1.000000000000000000 ) ) ;
#46021=EDGE_LOOP ( 'NONE', ( #16970, #49436, #23036, #644 ) ) ;
#46022=EDGE_LOOP ( 'NONE', ( #10832, #36173, #10213, #19225, #36905, #27208, #3582, #1363 ) ) ;
#46025=VERTEX_POINT ( 'NONE', #30399 ) ;
#46029=AXIS2_PLACEMENT_3D ( 'NONE', #14277, #27109, #6845 ) ;
#46030=ORIENTED_EDGE ( 'NONE', *, *, #10135, .F. ) ;
#46031=VERTEX_POINT ( 'NONE', #1315 ) ;
#46033=EDGE_LOOP ( 'NONE', ( #40257, #31387, #15734, #27910 ) ) ;
#46039=DIRECTION ( 'NONE',  ( 1.860490536778032451E-50, 0.000000000000000000, -1.000000000000000000 ) ) ;
#46042=VERTEX_POINT ( 'NONE', #16692 ) ;
#46047=VERTEX_POINT ( 'NONE', #1056 ) ;
#46050=CARTESIAN_POINT ( 'NONE',  ( 185.0000000000000284, -168.9999999999999432, -115.0000000000001705 ) ) ;
#46051=( BOUNDED_CURVE ( )  B_SPLINE_CURVE ( 3, ( #37952, #17672, #37205, #44842 ),
 .UNSPECIFIED., .F., .F. ) 
 B_SPLINE_CURVE_WITH_KNOTS ( ( 4, 4 ),
 ( 1.570796326794903663, 3.141592653589793116 ),
 .UNSPECIFIED. ) 
 CURVE ( )  GEOMETRIC_REPRESENTATION_ITEM ( )  RATIONAL_B_SPLINE_CURVE ( ( 1.000000000000000000, 0.8047378541243667138, 0.8047378541243667138, 1.000000000000000000 ) ) 
 REPRESENTATION_ITEM ( '' )  );
#46054=ORIENTED_EDGE ( 'NONE', *, *, #46643, .T. ) ;
#46065=EDGE_CURVE ( 'NONE', #34142, #913, #42875, .T. ) ;
#46070=( GEOMETRIC_REPRESENTATION_CONTEXT ( 3 ) GLOBAL_UNCERTAINTY_ASSIGNED_CONTEXT ( ( #7605 ) ) GLOBAL_UNIT_ASSIGNED_CONTEXT ( ( #22635, #38812, #50031 ) ) REPRESENTATION_CONTEXT ( 'NONE', 'WORKASPACE' ) );
#46074=CARTESIAN_POINT ( 'NONE',  ( 340.0000000000000000, 183.3431457505076878, 358.3431457505073467 ) ) ;
#46078=CARTESIAN_POINT ( 'NONE',  ( 340.0000000000000568, 181.0000000000000284, 349.9999999999998295 ) ) ;
#46079=CARTESIAN_POINT ( 'NONE',  ( 355.9999999999999432, -183.0000000000001421, -358.0000000000003411 ) ) ;
#46080=VERTEX_POINT ( 'NONE', #48207 ) ;
#46087=CARTESIAN_POINT ( 'NONE',  ( 0.000000000000000000, 184.8000000000000114, 340.1999999999997044 ) ) ;
#46089=DIRECTION ( 'NONE',  ( 1.000000000000000000, 0.000000000000000000, 0.000000000000000000 ) ) ;
#46094=CARTESIAN_POINT ( 'NONE',  ( 185.0000000000000000, -268.4999999999993747, -114.9999999999999147 ) ) ;
#46095=CYLINDRICAL_SURFACE ( 'NONE', #20131, 2.000000000000001776 ) ;
#46099=CARTESIAN_POINT ( 'NONE',  ( 185.0000000000000284, 2.775557561562891351E-14, -111.0000000000001563 ) ) ;
#46109=( NAMED_UNIT ( * ) SI_UNIT ( $, .STERADIAN. ) SOLID_ANGLE_UNIT ( ) );
#46112=CARTESIAN_POINT ( 'NONE',  ( 339.9999999999999432, -166.6568542494925396, -341.6568542494925396 ) ) ;
#46113=CIRCLE ( 'NONE', #28143, 2.000000000000001776 ) ;
#46122=ORIENTED_EDGE ( 'NONE', *, *, #4179, .T. ) ;
#46123=CARTESIAN_POINT ( 'NONE',  ( 344.0000000000000000, 167.0000000000001990, -342.0000000000002842 ) ) ;
#46125=CARTESIAN_POINT ( 'NONE',  ( 181.0000000000000000, -270.4999999999999432, -339.9999999999998863 ) ) ;
#46129=ORIENTED_EDGE ( 'NONE', *, *, #887, .T. ) ;
#46134=AXIS2_PLACEMENT_3D ( 'NONE', #38737, #50476, #10756 ) ;
#46136=EDGE_CURVE ( 'NONE', #48233, #4709, #20762, .T. ) ;
#46137=EDGE_CURVE ( 'NONE', #18735, #33080, #41234, .T. ) ;
#46141=AXIS2_PLACEMENT_3D ( 'NONE', #42888, #29648, #10150 ) ;
#46150=CARTESIAN_POINT ( 'NONE',  ( 5.551115123125782702E-14, -168.9999999999999432, 341.9999999999997726 ) ) ;
#46159=VECTOR ( 'NONE', #14273, 1000.000000000000000 ) ;
#46162=DIRECTION ( 'NONE',  ( 0.000000000000000000, -1.000000000000000000, -3.186989995019654210E-49 ) ) ;
#46163=VERTEX_POINT ( 'NONE', #47700 ) ;
#46165=ADVANCED_FACE ( 'NONE', ( #24163 ), #39817, .F. ) ;
#46167=ORIENTED_EDGE ( 'NONE', *, *, #35294, .F. ) ;
#46176=AXIS2_PLACEMENT_3D ( 'NONE', #47718, #23659, #27764 ) ;
#46177=CARTESIAN_POINT ( 'NONE',  ( 0.000000000000000000, 169.0000000000000000, -344.0000000000001705 ) ) ;
#46188=( NAMED_UNIT ( * ) SI_UNIT ( $, .STERADIAN. ) SOLID_ANGLE_UNIT ( ) );
#46197=EDGE_CURVE ( 'NONE', #45172, #28471, #32876, .T. ) ;
#46206=ORIENTED_EDGE ( 'NONE', *, *, #49039, .F. ) ;
#46209=ORIENTED_EDGE ( 'NONE', *, *, #8080, .T. ) ;
#46214=DIRECTION ( 'NONE',  ( -1.586032880504786307E-16, 1.654361225106055350E-24, -1.000000000000000000 ) ) ;
#46215=VECTOR ( 'NONE', #5032, 1000.000000000000000 ) ;
#46216=( BOUNDED_CURVE ( )  B_SPLINE_CURVE ( 3, ( #45617, #26395, #26141, #14849 ),
 .UNSPECIFIED., .F., .F. ) 
 B_SPLINE_CURVE_WITH_KNOTS ( ( 4, 4 ),
 ( 4.712388980384662140, 6.283185307179586232 ),
 .UNSPECIFIED. ) 
 CURVE ( )  GEOMETRIC_REPRESENTATION_ITEM ( )  RATIONAL_B_SPLINE_CURVE ( ( 1.000000000000000000, 0.8047378541243583872, 0.8047378541243583872, 1.000000000000000000 ) ) 
 REPRESENTATION_ITEM ( '' )  );
#46217=EDGE_LOOP ( 'NONE', ( #32317, #38640, #38207, #43118 ) ) ;
#46218=ORIENTED_EDGE ( 'NONE', *, *, #28383, .F. ) ;
#46222=DIRECTION ( 'NONE',  ( 0.000000000000000000, -1.000000000000000000, 0.000000000000000000 ) ) ;
#46229=CARTESIAN_POINT ( 'NONE',  ( 339.9999999999999432, 167.0000000000000000, -344.0000000000001705 ) ) ;
#46232=EDGE_CURVE ( 'NONE', #46936, #27142, #14098, .T. ) ;
#46241=ORIENTED_EDGE ( 'NONE', *, *, #737, .F. ) ;
#46242=VECTOR ( 'NONE', #29080, 1000.000000000000000 ) ;
#46243=CARTESIAN_POINT ( 'NONE',  ( 0.000000000000000000, 169.0000000000000000, -360.0000000000002274 ) ) ;
#46254=AXIS2_PLACEMENT_3D ( 'NONE', #6065, #40473, #17363 ) ;
#46256=VERTEX_POINT ( 'NONE', #46391 ) ;
#46263=EDGE_CURVE ( 'NONE', #29971, #17736, #38244, .T. ) ;
#46265=CARTESIAN_POINT ( 'NONE',  ( 169.0000000000000000, -174.9999999999999716, -113.0000000000001563 ) ) ;
#46273=AXIS2_PLACEMENT_3D ( 'NONE', #370, #47267, #35029 ) ;
#46281=ORIENTED_EDGE ( 'NONE', *, *, #33426, .F. ) ;
#46284=CARTESIAN_POINT ( 'NONE',  ( 355.9999999999999432, -174.9999999999999432, 359.9999999999998295 ) ) ;
#46286=CIRCLE ( 'NONE', #2092, 2.000000000000001776 ) ;
#46287=ORIENTED_EDGE ( 'NONE', *, *, #33705, .F. ) ;
#46299=DIRECTION ( 'NONE',  ( 1.000000000000000000, 0.000000000000000000, 0.000000000000000000 ) ) ;
#46302=EDGE_LOOP ( 'NONE', ( #4109, #12464, #12304, #24865 ) ) ;
#46305=CARTESIAN_POINT ( 'NONE',  ( 185.0000000000000568, 175.0000000000000284, 343.9999999999998863 ) ) ;
#46307=ADVANCED_FACE ( 'NONE', ( #6918 ), #23062, .T. ) ;
#46310=ORIENTED_EDGE ( 'NONE', *, *, #44882, .F. ) ;
#46313=CARTESIAN_POINT ( 'NONE',  ( 5.551115123125782702E-14, -166.9999999999999432, 355.9999999999997726 ) ) ;
#46314=VECTOR ( 'NONE', #590, 1000.000000000000000 ) ;
#46315=DIRECTION ( 'NONE',  ( 3.172065784643303486E-16, 1.000000000000000000, 8.758115402030106693E-47 ) ) ;
#46323=AXIS2_PLACEMENT_3D ( 'NONE', #13225, #9637, #48082 ) ;
#46324=CARTESIAN_POINT ( 'NONE',  ( 339.9999999999999432, 181.0000000000000284, -344.0000000000001705 ) ) ;
#46327=PLANE ( 'NONE',  #351 ) ;
#46328=( GEOMETRIC_REPRESENTATION_CONTEXT ( 3 ) GLOBAL_UNCERTAINTY_ASSIGNED_CONTEXT ( ( #12786 ) ) GLOBAL_UNIT_ASSIGNED_CONTEXT ( ( #47510, #35514, #12639 ) ) REPRESENTATION_CONTEXT ( 'NONE', 'WORKASPACE' ) );
#46330=CARTESIAN_POINT ( 'NONE',  ( 185.0000000000000000, -164.9999999999999432, -356.0000000000001705 ) ) ;
#46338=FACE_OUTER_BOUND ( 'NONE', #20977, .T. ) ;
#46352=EDGE_CURVE ( 'NONE', #15209, #12301, #26674, .T. ) ;
#46353=VECTOR ( 'NONE', #23166, 1000.000000000000000 ) ;
#46362=DIRECTION ( 'NONE',  ( 1.612977847700450206E-50, 0.000000000000000000, -1.000000000000000000 ) ) ;
#46363=EDGE_CURVE ( 'NONE', #16830, #27540, #30785, .T. ) ;
#46367=DIRECTION ( 'NONE',  ( 1.000000000000000000, 0.000000000000000000, -4.758098676964956461E-16 ) ) ;
#46370=ORIENTED_EDGE ( 'NONE', *, *, #18029, .T. ) ;
#46375=CARTESIAN_POINT ( 'NONE',  ( 344.0000000000000000, 175.0000000000000284, -92.00000000000019895 ) ) ;
#46391=CARTESIAN_POINT ( 'NONE',  ( 339.9999999999998863, -166.9999999999999432, 355.9999999999997726 ) ) ;
#46404=CARTESIAN_POINT ( 'NONE',  ( 344.0000000000000000, 174.9999999999996874, -342.0000000000002842 ) ) ;
#46413=CARTESIAN_POINT ( 'NONE',  ( 359.9999999999999432, -181.0000000000001421, -356.0000000000003411 ) ) ;
#46419=EDGE_LOOP ( 'NONE', ( #40482, #35769, #30793, #10119 ) ) ;
#46420=DIRECTION ( 'NONE',  ( 0.000000000000000000, -1.000000000000000000, 0.000000000000000000 ) ) ;
#46424=DIRECTION ( 'NONE',  ( -1.000000000000000000, -0.000000000000000000, 0.000000000000000000 ) ) ;
#46425=CARTESIAN_POINT ( 'NONE',  ( 339.9999999999999432, 174.9999999999996589, -344.0000000000002842 ) ) ;
#46427=FACE_OUTER_BOUND ( 'NONE', #37763, .T. ) ;
#46432=DIRECTION ( 'NONE',  ( 6.203854594147707562E-25, -2.067951531382569187E-25, 1.000000000000000000 ) ) ;
#46434=VERTEX_POINT ( 'NONE', #7945 ) ;
#46443=DIRECTION ( 'NONE',  ( 1.000000000000000000, 0.000000000000000000, 0.000000000000000000 ) ) ;
#46447=LINE ( 'NONE', #22632, #177 ) ;
#46451=CIRCLE ( 'NONE', #23574, 4.000000000000003553 ) ;
#46453=CARTESIAN_POINT ( 'NONE',  ( 344.0000000000000000, 165.0000000000001990, -340.0000000000002842 ) ) ;
#46454=CARTESIAN_POINT ( 'NONE',  ( 339.9999999999999432, 181.0000000000000284, -342.0000000000001705 ) ) ;
#46458=CARTESIAN_POINT ( 'NONE',  ( 168.9999999999999716, -164.9999999999999432, -342.0000000000001137 ) ) ;
#46460=CARTESIAN_POINT ( 'NONE',  ( 181.0000000000000000, -180.9999999999999716, -350.0000000000001705 ) ) ;
#46463=DIRECTION ( 'NONE',  ( 1.000000000000000000, 0.000000000000000000, 0.000000000000000000 ) ) ;
#46470=ORIENTED_EDGE ( 'NONE', *, *, #47785, .F. ) ;
#46472=VERTEX_POINT ( 'NONE', #27941 ) ;
#46474=CARTESIAN_POINT ( 'NONE',  ( 356.0000000000006253, 167.0000000000000000, -342.0000000000001137 ) ) ;
#46475=CARTESIAN_POINT ( 'NONE',  ( 168.9999999999999716, 165.0000000000000000, -344.0000000000001137 ) ) ;
#46477=DIRECTION ( 'NONE',  ( 0.000000000000000000, -1.000000000000000000, 0.000000000000000000 ) ) ;
#46488=ORIENTED_EDGE ( 'NONE', *, *, #11133, .T. ) ;
#46492=ORIENTED_EDGE ( 'NONE', *, *, #13614, .T. ) ;
#46493=DIRECTION ( 'NONE',  ( 1.000000000000000000, 0.000000000000000000, 0.000000000000000000 ) ) ;
#46496=ORIENTED_EDGE ( 'NONE', *, *, #29451, .F. ) ;
#46498=LINE ( 'NONE', #19592, #36732 ) ;
#46512=EDGE_CURVE ( 'NONE', #20771, #38870, #41267, .T. ) ;
#46521=CARTESIAN_POINT ( 'NONE',  ( 168.9999999999999716, 175.0000000000000284, -356.0000000000001705 ) ) ;
#46525=CARTESIAN_POINT ( 'NONE',  ( 0.000000000000000000, -165.1999999999999602, 359.7999999999997840 ) ) ;
#46538=DIRECTION ( 'NONE',  ( 1.000000000000000000, 0.000000000000000000, 0.000000000000000000 ) ) ;
#46539=ORIENTED_EDGE ( 'NONE', *, *, #13609, .T. ) ;
#46540=ORIENTED_EDGE ( 'NONE', *, *, #25353, .T. ) ;
#46542=PLANE ( 'NONE',  #35729 ) ;
#46544=VERTEX_POINT ( 'NONE', #48894 ) ;
#46545=DIRECTION ( 'NONE',  ( 1.000000000000000000, 0.000000000000000000, 7.793956916774525800E-48 ) ) ;
#46551=LINE ( 'NONE', #23512, #35805 ) ;
#46553=UNCERTAINTY_MEASURE_WITH_UNIT (LENGTH_MEASURE( 1.000000000000000082E-05 ), #52, 'distance_accuracy_value', 'NONE');
#46554=EDGE_LOOP ( 'NONE', ( #42374, #16778, #39482, #26190 ) ) ;
#46558=VECTOR ( 'NONE', #4765, 1000.000000000000000 ) ;
#46559=CARTESIAN_POINT ( 'NONE',  ( 168.9999999999999716, -81.49999999999995737, -115.0000000000001563 ) ) ;
#46573=ORIENTED_EDGE ( 'NONE', *, *, #28499, .F. ) ;
#46575=EDGE_CURVE ( 'NONE', #22827, #39841, #13277, .T. ) ;
#46576=DIRECTION ( 'NONE',  ( -1.000000000000000000, 0.000000000000000000, -1.586032872232979935E-16 ) ) ;
#46580=LINE ( 'NONE', #4030, #7378 ) ;
#46582=CARTESIAN_POINT ( 'NONE',  ( 343.9999999999999432, -183.0000000000001421, 358.0000000000001137 ) ) ;
#46592=VECTOR ( 'NONE', #6032, 1000.000000000000000 ) ;
#46594=ORIENTED_EDGE ( 'NONE', *, *, #50000, .F. ) ;
#46597=LINE ( 'NONE', #31768, #15086 ) ;
#46599=VECTOR ( 'NONE', #38303, 1000.000000000000000 ) ;
#46601=AXIS2_PLACEMENT_3D ( 'NONE', #41062, #5905, #25930 ) ;
#46609=LINE ( 'NONE', #3031, #13839 ) ;
#46610=ORIENTED_EDGE ( 'NONE', *, *, #32558, .T. ) ;
#46613=CARTESIAN_POINT ( 'NONE',  ( 0.000000000000000000, 169.0000000000000000, 357.9999999999997726 ) ) ;
#46614=LINE ( 'NONE', #42789, #38143 ) ;
#46615=EDGE_LOOP ( 'NONE', ( #1982, #41112, #44393, #49718 ) ) ;
#46628=DIRECTION ( 'NONE',  ( -1.000000000000000000, 0.000000000000000000, -7.793956916774525800E-48 ) ) ;
#46631=EDGE_CURVE ( 'NONE', #34498, #37542, #9693, .T. ) ;
#46638=EDGE_CURVE ( 'NONE', #40480, #7451, #5847, .T. ) ;
#46642=EDGE_CURVE ( 'NONE', #50507, #21498, #47792, .T. ) ;
#46643=EDGE_CURVE ( 'NONE', #16943, #14950, #23000, .T. ) ;
#46648=LINE ( 'NONE', #11548, #19638 ) ;
#46650=EDGE_CURVE ( 'NONE', #35217, #1861, #30459, .T. ) ;
#46651=LINE ( 'NONE', #34912, #20521 ) ;
#46656=ORIENTED_EDGE ( 'NONE', *, *, #18029, .F. ) ;
#46658=VERTEX_POINT ( 'NONE', #50150 ) ;
#46660=FACE_OUTER_BOUND ( 'NONE', #4596, .T. ) ;
#46666=ORIENTED_EDGE ( 'NONE', *, *, #44738, .F. ) ;
#46667=CARTESIAN_POINT ( 'NONE',  ( 165.0000000000000000, -81.49999999999995737, -115.0000000000001563 ) ) ;
#46669=LINE ( 'NONE', #39277, #33792 ) ;
#46671=VECTOR ( 'NONE', #16029, 1000.000000000000000 ) ;
#46675=ORIENTED_EDGE ( 'NONE', *, *, #49014, .F. ) ;
#46678=VECTOR ( 'NONE', #39799, 1000.000000000000000 ) ;
#46682=CARTESIAN_POINT ( 'NONE',  ( 355.9999999999999432, -183.0000000000001421, -349.9999999999998863 ) ) ;
#46683=CARTESIAN_POINT ( 'NONE',  ( 357.9999999999999432, -181.0000000000001421, -356.0000000000003979 ) ) ;
#46689=FACE_OUTER_BOUND ( 'NONE', #2401, .T. ) ;
#46690=CARTESIAN_POINT ( 'NONE',  ( 344.0000000000000000, 165.0000000000000000, -92.00000000000019895 ) ) ;
#46701=VECTOR ( 'NONE', #1771, 1000.000000000000000 ) ;
#46703=( LENGTH_UNIT ( ) NAMED_UNIT ( * ) SI_UNIT ( .MILLI., .METRE. ) );
#46705=CARTESIAN_POINT ( 'NONE',  ( 183.0000000000000000, -168.9999999999999432, -350.0000000000001705 ) ) ;
#46710=PLANE ( 'NONE',  #27895 ) ;
#46713=CIRCLE ( 'NONE', #42639, 4.000000000000003553 ) ;
#46715=ORIENTED_EDGE ( 'NONE', *, *, #489, .T. ) ;
#46723=ORIENTED_EDGE ( 'NONE', *, *, #15141, .T. ) ;
#46729=LINE ( 'NONE', #46229, #13311 ) ;
#46741=FACE_BOUND ( 'NONE', #29290, .T. ) ;
#46744=EDGE_LOOP ( 'NONE', ( #9870, #37536, #20997, #47993 ) ) ;
#46748=CARTESIAN_POINT ( 'NONE',  ( 168.9999999999999716, -5.999999999999950262, -340.0000000000001137 ) ) ;
#46751=DIRECTION ( 'NONE',  ( -1.000000000000000000, 0.000000000000000000, -7.793956916774525800E-48 ) ) ;
#46760=CARTESIAN_POINT ( 'NONE',  ( 167.0000000000000000, -9.999999999999953815, -111.0000000000001563 ) ) ;
#46765=DIRECTION ( 'NONE',  ( 0.000000000000000000, -1.000000000000000000, 0.000000000000000000 ) ) ;
#46766=ADVANCED_FACE ( 'NONE', ( #42256, #42004 ), #46327, .T. ) ;
#46767=VECTOR ( 'NONE', #4703, 1000.000000000000000 ) ;
#46768=EDGE_LOOP ( 'NONE', ( #50569, #4614, #24829, #6197, #46666, #40519, #39110, #7786 ) ) ;
#46771=PLANE ( 'NONE',  #29903 ) ;
#46773=EDGE_CURVE ( 'NONE', #21399, #46031, #25668, .T. ) ;
#46774=ADVANCED_FACE ( 'NONE', ( #26861 ), #42499, .T. ) ;
#46780=ADVANCED_FACE ( 'NONE', ( #41667 ), #2411, .T. ) ;
#46783=CARTESIAN_POINT ( 'NONE',  ( 357.9999999999999432, -180.9999999999999716, 355.9999999999998295 ) ) ;
#46795=ADVANCED_FACE ( 'NONE', ( #22168, #37589 ), #45227, .T. ) ;
#46801=VERTEX_POINT ( 'NONE', #1668 ) ;
#46802=ORIENTED_EDGE ( 'NONE', *, *, #11109, .T. ) ;
#46815=FACE_OUTER_BOUND ( 'NONE', #49966, .T. ) ;
#46818=CARTESIAN_POINT ( 'NONE',  ( 168.9999999999999716, -164.9999999999999432, -115.0000000000001847 ) ) ;
#46827=ORIENTED_EDGE ( 'NONE', *, *, #49247, .T. ) ;
#46829=ADVANCED_FACE ( 'NONE', ( #26026 ), #37348, .F. ) ;
#46830=CARTESIAN_POINT ( 'NONE',  ( 181.0000000000000000, -95.49999999999998579, -340.0000000000001137 ) ) ;
#46834=DIRECTION ( 'NONE',  ( 0.000000000000000000, 0.000000000000000000, -1.000000000000000000 ) ) ;
#46836=ORIENTED_EDGE ( 'NONE', *, *, #8255, .F. ) ;
#46838=CARTESIAN_POINT ( 'NONE',  ( 183.0000000000000000, 175.0000000000000284, -344.0000000000001137 ) ) ;
#46840=CARTESIAN_POINT ( 'NONE',  ( 166.9999999999999716, -164.9999999999999432, -356.0000000000001705 ) ) ;
#46845=ORIENTED_EDGE ( 'NONE', *, *, #6379, .T. ) ;
#46859=EDGE_CURVE ( 'NONE', #34025, #28991, #4436, .T. ) ;
#46861=DIRECTION ( 'NONE',  ( 0.000000000000000000, 1.000000000000000000, 0.000000000000000000 ) ) ;
#46863=VERTEX_POINT ( 'NONE', #11096 ) ;
#46869=ORIENTED_EDGE ( 'NONE', *, *, #21630, .F. ) ;
#46870=EDGE_CURVE ( 'NONE', #14588, #34800, #26000, .T. ) ;
#46878=( NAMED_UNIT ( * ) PLANE_ANGLE_UNIT ( ) SI_UNIT ( $, .RADIAN. ) );
#46883=VERTEX_POINT ( 'NONE', #49538 ) ;
#46885=DIRECTION ( 'NONE',  ( 0.000000000000000000, -2.265761274745217480E-16, 1.000000000000000000 ) ) ;
#46891=DIRECTION ( 'NONE',  ( 1.000000000000000000, 0.000000000000000000, -1.586032892321652482E-16 ) ) ;
#46896=DIRECTION ( 'NONE',  ( -4.758098676964957447E-16, -1.000000000000000000, 7.143884938411937192E-48 ) ) ;
#46899=( BOUNDED_CURVE ( )  B_SPLINE_CURVE ( 3, ( #11714, #27367, #43002, #7882 ),
 .UNSPECIFIED., .F., .F. ) 
 B_SPLINE_CURVE_WITH_KNOTS ( ( 4, 4 ),
 ( 3.141592653589793116, 4.712388980384689674 ),
 .UNSPECIFIED. ) 
 CURVE ( )  GEOMETRIC_REPRESENTATION_ITEM ( )  RATIONAL_B_SPLINE_CURVE ( ( 1.000000000000000000, 0.8047378541243649375, 0.8047378541243649375, 1.000000000000000000 ) ) 
 REPRESENTATION_ITEM ( '' )  );
#46903=EDGE_CURVE ( 'NONE', #14416, #11052, #30349, .T. ) ;
#46907=EDGE_LOOP ( 'NONE', ( #25187, #26384, #10791, #18716 ) ) ;
#46910=ORIENTED_EDGE ( 'NONE', *, *, #46650, .F. ) ;
#46913=CIRCLE ( 'NONE', #45273, 2.000000000000001776 ) ;
#46918=DIRECTION ( 'NONE',  ( 6.203854594147707562E-25, -2.067951531382569187E-25, 1.000000000000000000 ) ) ;
#46920=VERTEX_POINT ( 'NONE', #19034 ) ;
#46927=CARTESIAN_POINT ( 'NONE',  ( 168.9999999999999716, -272.4999999999999432, -349.9999999999999432 ) ) ;
#46933=CARTESIAN_POINT ( 'NONE',  ( 359.9999999999999432, -178.0000000000000000, 352.9999999999998295 ) ) ;
#46935=DIRECTION ( 'NONE',  ( 1.333906992743555050E-23, -1.000000000000000000, 0.000000000000000000 ) ) ;
#46936=VERTEX_POINT ( 'NONE', #10581 ) ;
#46939=EDGE_CURVE ( 'NONE', #25458, #19871, #27316, .T. ) ;
#46941=ORIENTED_EDGE ( 'NONE', *, *, #10867, .T. ) ;
#46942=ORIENTED_EDGE ( 'NONE', *, *, #48078, .T. ) ;
#46949=DIRECTION ( 'NONE',  ( 0.000000000000000000, -2.969158215481698263E-48, 1.000000000000000000 ) ) ;
#46960=STYLED_ITEM('',(#50747),#38306);
#46961=FACE_OUTER_BOUND ( 'NONE', #41536, .T. ) ;
#46963=DIRECTION ( 'NONE',  ( 0.000000000000000000, -1.000000000000000000, 0.000000000000000000 ) ) ;
#46966=( LENGTH_UNIT ( ) NAMED_UNIT ( * ) SI_UNIT ( .MILLI., .METRE. ) );
#46968=VERTEX_POINT ( 'NONE', #7248 ) ;
#46972=CARTESIAN_POINT ( 'NONE',  ( 168.9999999999999716, -164.9999999999999432, 355.9999999999998863 ) ) ;
#46983=FACE_BOUND ( 'NONE', #6582, .T. ) ;
#46984=VECTOR ( 'NONE', #6436, 1000.000000000000000 ) ;
#46985=DIRECTION ( 'NONE',  ( 0.000000000000000000, 0.000000000000000000, 1.000000000000000000 ) ) ;
#46986=ORIENTED_EDGE ( 'NONE', *, *, #45940, .T. ) ;
#46991=AXIS2_PLACEMENT_3D ( 'NONE', #5036, #45022, #24807 ) ;
#46994=AXIS2_PLACEMENT_3D ( 'NONE', #8447, #40004, #36677 ) ;
#46998=ORIENTED_EDGE ( 'NONE', *, *, #4226, .F. ) ;
#47015=EDGE_LOOP ( 'NONE', ( #33428, #23015, #45037, #41959 ) ) ;
#47017=CARTESIAN_POINT ( 'NONE',  ( 5.551115123125782702E-14, -168.9999999999999432, 341.9999999999997726 ) ) ;
#47027=CIRCLE ( 'NONE', #29050, 4.000000000000003553 ) ;
#47028=EDGE_CURVE ( 'NONE', #19710, #13422, #20033, .T. ) ;
#47043=DIRECTION ( 'NONE',  ( 0.000000000000000000, -0.000000000000000000, 1.000000000000000000 ) ) ;
#47051=ORIENTED_EDGE ( 'NONE', *, *, #14505, .T. ) ;
#47052=CARTESIAN_POINT ( 'NONE',  ( 358.0000000000001137, 167.8284271247464687, 342.8284271247463266 ) ) ;
#47053=CARTESIAN_POINT ( 'NONE',  ( 356.0000000000006253, 167.0000000000000000, 341.9999999999998295 ) ) ;
#47055=VECTOR ( 'NONE', #36830, 1000.000000000000000 ) ;
#47056=VERTEX_POINT ( 'NONE', #16710 ) ;
#47073=CARTESIAN_POINT ( 'NONE',  ( 339.9999999999999432, -181.0000000000001421, -356.0000000000003411 ) ) ;
#47075=CARTESIAN_POINT ( 'NONE',  ( 359.9999999999999432, 174.9999999999996589, -356.0000000000003411 ) ) ;
#47076=VECTOR ( 'NONE', #34712, 1000.000000000000000 ) ;
#47079=ADVANCED_FACE ( 'NONE', ( #35983 ), #15703, .T. ) ;
#47083=CARTESIAN_POINT ( 'NONE',  ( 168.9999999999998863, 165.0000000000000000, 357.9999999999998863 ) ) ;
#47100=DIRECTION ( 'NONE',  ( 1.000000000000000000, 0.000000000000000000, 4.758098658057970186E-16 ) ) ;
#47102=DIRECTION ( 'NONE',  ( 2.958228394578793832E-31, 0.000000000000000000, 1.000000000000000000 ) ) ;
#47104=LINE ( 'NONE', #12009, #21706 ) ;
#47106=LINE ( 'NONE', #12011, #7029 ) ;
#47113=ORIENTED_EDGE ( 'NONE', *, *, #176, .F. ) ;
#47118=EDGE_CURVE ( 'NONE', #40366, #46863, #4163, .T. ) ;
#47119=CIRCLE ( 'NONE', #34877, 4.000000000000003553 ) ;
#47123=EDGE_CURVE ( 'NONE', #16301, #26083, #32573, .T. ) ;
#47127=AXIS2_PLACEMENT_3D ( 'NONE', #23896, #32105, #12847 ) ;
#47138=LINE ( 'NONE', #30517, #42972 ) ;
#47143=DIRECTION ( 'NONE',  ( 0.000000000000000000, 0.000000000000000000, -1.000000000000000000 ) ) ;
#47150=VECTOR ( 'NONE', #5613, 1000.000000000000000 ) ;
#47154=DIRECTION ( 'NONE',  ( -1.586032892321652236E-16, -1.000000000000000000, -2.288264760618012091E-48 ) ) ;
#47155=AXIS2_PLACEMENT_3D ( 'NONE', #13507, #17614, #41722 ) ;
#47160=EDGE_CURVE ( 'NONE', #28712, #34498, #1332, .T. ) ;
#47163=ORIENTED_EDGE ( 'NONE', *, *, #17840, .T. ) ;
#47164=VECTOR ( 'NONE', #29418, 1000.000000000000000 ) ;
#47165=ORIENTED_EDGE ( 'NONE', *, *, #14872, .T. ) ;
#47167=DIRECTION ( 'NONE',  ( 0.000000000000000000, -1.000000000000000000, -3.186989995019654210E-49 ) ) ;
#47168=CIRCLE ( 'NONE', #16050, 2.000000000000001776 ) ;
#47169=VERTEX_POINT ( 'NONE', #9515 ) ;
#47173=VERTEX_POINT ( 'NONE', #29023 ) ;
#47178=VERTEX_POINT ( 'NONE', #44641 ) ;
#47189=DIRECTION ( 'NONE',  ( 0.000000000000000000, 1.000000000000000000, 0.000000000000000000 ) ) ;
#47190=AXIS2_PLACEMENT_3D ( 'NONE', #87, #5182, #24197 ) ;
#47196=CARTESIAN_POINT ( 'NONE',  ( 166.9999999999999716, -256.4999999999996589, -114.9999999999999574 ) ) ;
#47198=VERTEX_POINT ( 'NONE', #40324 ) ;
#47204=AXIS2_PLACEMENT_3D ( 'NONE', #30716, #34562, #38173 ) ;
#47211=FACE_OUTER_BOUND ( 'NONE', #32592, .T. ) ;
#47215=DIRECTION ( 'NONE',  ( -5.473822126268816076E-48, 1.000000000000000000, 1.654361225106055350E-24 ) ) ;
#47216=EDGE_CURVE ( 'NONE', #31506, #9910, #24771, .T. ) ;
#47223=CARTESIAN_POINT ( 'NONE',  ( 339.9999999999999432, -169.0000000000001137, 344.0000000000000000 ) ) ;
#47230=PLANE ( 'NONE',  #40162 ) ;
#47234=DIRECTION ( 'NONE',  ( -1.000000000000000000, 0.000000000000000000, 1.586032892321651989E-16 ) ) ;
#47238=ORIENTED_EDGE ( 'NONE', *, *, #33834, .T. ) ;
#47246=VERTEX_POINT ( 'NONE', #18974 ) ;
#47247=ORIENTED_EDGE ( 'NONE', *, *, #24892, .T. ) ;
#47248=VECTOR ( 'NONE', #4435, 1000.000000000000000 ) ;
#47252=ORIENTED_EDGE ( 'NONE', *, *, #2313, .T. ) ;
#47254=PLANE ( 'NONE',  #13191 ) ;
#47261=EDGE_CURVE ( 'NONE', #23604, #15862, #49471, .T. ) ;
#47263=EDGE_LOOP ( 'NONE', ( #10974, #43440 ) ) ;
#47265=FACE_OUTER_BOUND ( 'NONE', #50293, .T. ) ;
#47267=DIRECTION ( 'NONE',  ( 1.586032892321651989E-16, -3.736034562988530447E-32, 1.000000000000000000 ) ) ;
#47271=DIRECTION ( 'NONE',  ( 0.000000000000000000, 0.000000000000000000, -1.000000000000000000 ) ) ;
#47272=ORIENTED_EDGE ( 'NONE', *, *, #25307, .T. ) ;
#47290=FACE_OUTER_BOUND ( 'NONE', #27303, .T. ) ;
#47303=DIRECTION ( 'NONE',  ( -1.000000000000000000, 0.000000000000000000, 0.000000000000000000 ) ) ;
#47305=ORIENTED_EDGE ( 'NONE', *, *, #10006, .T. ) ;
#47310=LINE ( 'NONE', #16305, #37762 ) ;
#47311=ORIENTED_EDGE ( 'NONE', *, *, #12533, .F. ) ;
#47318=ORIENTED_EDGE ( 'NONE', *, *, #13519, .T. ) ;
#47324=DIRECTION ( 'NONE',  ( 0.000000000000000000, -2.969158215481698263E-48, 1.000000000000000000 ) ) ;
#47331=LINE ( 'NONE', #11978, #29386 ) ;
#47332=CARTESIAN_POINT ( 'NONE',  ( 183.0000000000000000, -268.5000000000000000, -339.9999999999998863 ) ) ;
#47333=AXIS2_PLACEMENT_3D ( 'NONE', #14288, #10952, #37923 ) ;
#47335=DIRECTION ( 'NONE',  ( 1.000000000000000000, 0.000000000000000000, 0.000000000000000000 ) ) ;
#47337=ORIENTED_EDGE ( 'NONE', *, *, #4350, .F. ) ;
#47343=LINE ( 'NONE', #23267, #26478 ) ;
#47344=DIRECTION ( 'NONE',  ( -1.000000000000000000, 0.000000000000000000, 1.860490536778032451E-50 ) ) ;
#47346=CARTESIAN_POINT ( 'NONE',  ( 339.9999999999999432, -166.9999999999999432, -356.0000000000002274 ) ) ;
#47351=CARTESIAN_POINT ( 'NONE',  ( 356.0000000000000568, 183.0000000000000853, 357.9999999999998295 ) ) ;
#47353=DIRECTION ( 'NONE',  ( -1.000000000000000000, 0.000000000000000000, -7.793956916774525800E-48 ) ) ;
#47354=DIRECTION ( 'NONE',  ( 1.000000000000000000, 6.344131455081961406E-16, -4.759647537211363479E-16 ) ) ;
#47357=ORIENTED_EDGE ( 'NONE', *, *, #24488, .T. ) ;
#47360=( LENGTH_UNIT ( ) NAMED_UNIT ( * ) SI_UNIT ( .MILLI., .METRE. ) );
#47362=CIRCLE ( 'NONE', #12964, 2.000000000000001776 ) ;
#47367=ORIENTED_EDGE ( 'NONE', *, *, #39555, .F. ) ;
#47369=DIRECTION ( 'NONE',  ( 0.000000000000000000, 0.000000000000000000, -1.000000000000000000 ) ) ;
#47371=CLOSED_SHELL ( 'NONE', ( #33704, #24746, #23676, #11738, #17735, #6302, #19686, #15298, #12787, #28997, #3103, #17087, #44601, #12039, #36046, #13011, #50618, #39161 ) ) ;
#47382=DIRECTION ( 'NONE',  ( 0.000000000000000000, 0.000000000000000000, -1.000000000000000000 ) ) ;
#47383=DIRECTION ( 'NONE',  ( 3.364279341222519273E-16, -0.7071067811865474617, 0.7071067811865476838 ) ) ;
#47385=CARTESIAN_POINT ( 'NONE',  ( 169.0000000000000000, -174.9999999999999716, -95.00000000000014211 ) ) ;
#47391=AXIS2_PLACEMENT_3D ( 'NONE', #20667, #1187, #24786 ) ;
#47394=CARTESIAN_POINT ( 'NONE',  ( 166.9999999999999716, -5.999999999999950262, -350.0000000000001705 ) ) ;
#47395=CIRCLE ( 'NONE', #38450, 4.000000000000003553 ) ;
#47397=DIRECTION ( 'NONE',  ( -1.000000000000000000, 0.000000000000000000, -1.612977847700450206E-50 ) ) ;
#47398=VECTOR ( 'NONE', #34960, 1000.000000000000000 ) ;
#47402=EDGE_CURVE ( 'NONE', #9482, #27139, #50268, .T. ) ;
#47404=DIRECTION ( 'NONE',  ( -1.000000000000000000, 0.000000000000000000, 1.132880637372608740E-16 ) ) ;
#47409=ORIENTED_EDGE ( 'NONE', *, *, #33432, .F. ) ;
#47413=VERTEX_POINT ( 'NONE', #24121 ) ;
#47419=ADVANCED_FACE ( 'NONE', ( #3578 ), #8721, .F. ) ;
#47426=EDGE_CURVE ( 'NONE', #10712, #45613, #42950, .T. ) ;
#47431=DIRECTION ( 'NONE',  ( 0.000000000000000000, -0.000000000000000000, 1.000000000000000000 ) ) ;
#47435=DIRECTION ( 'NONE',  ( 6.203854594147707562E-25, -2.067951531382569187E-25, 1.000000000000000000 ) ) ;
#47437=CARTESIAN_POINT ( 'NONE',  ( 168.9999999999999716, -268.4999999999999432, -349.9999999999999432 ) ) ;
#47439=CARTESIAN_POINT ( 'NONE',  ( 342.0000000000000568, -178.0000000000000853, 2.999999999999892086 ) ) ;
#47448=VECTOR ( 'NONE', #22256, 1000.000000000000000 ) ;
#47450=ORIENTED_EDGE ( 'NONE', *, *, #8043, .T. ) ;
#47452=VECTOR ( 'NONE', #16036, 1000.000000000000000 ) ;
#47469=ORIENTED_EDGE ( 'NONE', *, *, #19952, .F. ) ;
#47475=AXIS2_PLACEMENT_3D ( 'NONE', #3330, #45402, #49989 ) ;
#47477=ADVANCED_FACE ( 'NONE', ( #44570 ), #24615, .F. ) ;
#47483=CARTESIAN_POINT ( 'NONE',  ( 341.9999999999999432, -182.1715728752535597, 357.1715728752534460 ) ) ;
#47485=CARTESIAN_POINT ( 'NONE',  ( 359.9999999999999432, 181.0000000000002274, -356.0000000000003411 ) ) ;
#47491=EDGE_CURVE ( 'NONE', #46801, #21789, #1109, .T. ) ;
#47492=VECTOR ( 'NONE', #47234, 1000.000000000000000 ) ;
#47493=ORIENTED_EDGE ( 'NONE', *, *, #36847, .F. ) ;
#47494=CARTESIAN_POINT ( 'NONE',  ( 181.0000000000000000, -272.4999999999999432, -349.9999999999999432 ) ) ;
#47497=EDGE_CURVE ( 'NONE', #6873, #48314, #13548, .T. ) ;
#47501=CYLINDRICAL_SURFACE ( 'NONE', #14448, 4.000000000000003553 ) ;
#47502=CYLINDRICAL_SURFACE ( 'NONE', #42725, 2.000000000000001776 ) ;
#47504=ADVANCED_FACE ( 'NONE', ( #36693 ), #45080, .T. ) ;
#47507=ORIENTED_EDGE ( 'NONE', *, *, #8016, .F. ) ;
#47508=DIRECTION ( 'NONE',  ( -7.793956916774525800E-48, 0.000000000000000000, -1.000000000000000000 ) ) ;
#47510=( LENGTH_UNIT ( ) NAMED_UNIT ( * ) SI_UNIT ( .MILLI., .METRE. ) );
#47515=AXIS2_PLACEMENT_3D ( 'NONE', #30226, #17904, #49174 ) ;
#47516=ORIENTED_EDGE ( 'NONE', *, *, #25020, .T. ) ;
#47517=ADVANCED_FACE ( 'NONE', ( #20749 ), #36430, .T. ) ;
#47520=VERTEX_POINT ( 'NONE', #44333 ) ;
#47522=CARTESIAN_POINT ( 'NONE',  ( 358.3431457505076310, 185.0000000000000284, -360.0000000000002274 ) ) ;
#47524=FACE_OUTER_BOUND ( 'NONE', #22602, .T. ) ;
#47531=CIRCLE ( 'NONE', #27902, 4.000000000000003553 ) ;
#47535=LINE ( 'NONE', #12414, #33569 ) ;
#47537=DIRECTION ( 'NONE',  ( 1.333906992743555050E-23, -1.000000000000000000, 0.000000000000000000 ) ) ;
#47540=CARTESIAN_POINT ( 'NONE',  ( 340.0000000000000000, 175.0000000000000284, -94.00000000000019895 ) ) ;
#47542=DIRECTION ( 'NONE',  ( 2.958228394578793832E-31, 0.000000000000000000, 1.000000000000000000 ) ) ;
#47553=CARTESIAN_POINT ( 'NONE',  ( 349.9999999999999432, -180.9999999999999716, 343.9999999999997726 ) ) ;
#47560=ORIENTED_EDGE ( 'NONE', *, *, #45653, .F. ) ;
#47561=EDGE_CURVE ( 'NONE', #19563, #47056, #32826, .T. ) ;
#47563=LINE ( 'NONE', #43744, #18063 ) ;
#47566=DIRECTION ( 'NONE',  ( 1.000000000000000000, 0.000000000000000000, 0.000000000000000000 ) ) ;
#47571=ORIENTED_EDGE ( 'NONE', *, *, #48868, .T. ) ;
#47573=ORIENTED_EDGE ( 'NONE', *, *, #29322, .F. ) ;
#47577=EDGE_LOOP ( 'NONE', ( #754, #36337, #3646, #32313 ) ) ;
#47578=EDGE_CURVE ( 'NONE', #12301, #24963, #33076, .T. ) ;
#47595=FACE_OUTER_BOUND ( 'NONE', #13175, .T. ) ;
#47613=VERTEX_POINT ( 'NONE', #22768 ) ;
#47624=DIRECTION ( 'NONE',  ( 0.000000000000000000, -1.000000000000000000, 0.000000000000000000 ) ) ;
#47626=VECTOR ( 'NONE', #24432, 1000.000000000000000 ) ;
#47629=CARTESIAN_POINT ( 'NONE',  ( 181.0000000000000000, -174.9999999999999716, -344.0000000000001137 ) ) ;
#47638=DIRECTION ( 'NONE',  ( 0.000000000000000000, 1.000000000000000000, 1.544785076050074834E-48 ) ) ;
#47643=ORIENTED_EDGE ( 'NONE', *, *, #12105, .F. ) ;
#47648=EDGE_LOOP ( 'NONE', ( #37266, #7237, #5038, #28245 ) ) ;
#47651=LINE ( 'NONE', #20746, #27037 ) ;
#47658=ORIENTED_EDGE ( 'NONE', *, *, #13922, .F. ) ;
#47662=DIRECTION ( 'NONE',  ( -0.000000000000000000, -0.000000000000000000, 1.000000000000000000 ) ) ;
#47665=CARTESIAN_POINT ( 'NONE',  ( 359.9999999999999432, -181.0000000000001421, -349.9999999999998863 ) ) ;
#47671=DIRECTION ( 'NONE',  ( 0.000000000000000000, -3.186989995019654210E-49, -1.000000000000000000 ) ) ;
#47679=DIRECTION ( 'NONE',  ( 0.000000000000000000, 3.186989995019654210E-49, 1.000000000000000000 ) ) ;
#47681=AXIS2_PLACEMENT_3D ( 'NONE', #31626, #47215, #12114 ) ;
#47688=FACE_OUTER_BOUND ( 'NONE', #40599, .T. ) ;
#47689=DIRECTION ( 'NONE',  ( 1.132880637372608740E-16, 4.718402560806925739E-50, 1.000000000000000000 ) ) ;
#47698=CARTESIAN_POINT ( 'NONE',  ( 356.0000000000001137, 183.0000000000000284, 357.9999999999998295 ) ) ;
#47700=CARTESIAN_POINT ( 'NONE',  ( 358.0000000000000000, 169.0000000000000000, -344.0000000000001137 ) ) ;
#47704=EDGE_CURVE ( 'NONE', #35493, #2551, #45823, .T. ) ;
#47711=VERTEX_POINT ( 'NONE', #22007 ) ;
#47714=FACE_OUTER_BOUND ( 'NONE', #9803, .T. ) ;
#47716=ORIENTED_EDGE ( 'NONE', *, *, #2492, .F. ) ;
#47718=CARTESIAN_POINT ( 'NONE',  ( 181.0000000000000000, -164.9999999999999432, -356.0000000000001705 ) ) ;
#47724=AXIS2_PLACEMENT_3D ( 'NONE', #16335, #46834, #8391 ) ;
#47726=EDGE_CURVE ( 'NONE', #44375, #38075, #29974, .T. ) ;
#47734=VERTEX_POINT ( 'NONE', #42270 ) ;
#47737=VERTEX_POINT ( 'NONE', #38198 ) ;
#47743=DIRECTION ( 'NONE',  ( 6.203854594147707562E-25, -2.067951531382569187E-25, 1.000000000000000000 ) ) ;
#47745=EDGE_CURVE ( 'NONE', #11842, #19947, #30587, .T. ) ;
#47758=ADVANCED_FACE ( 'NONE', ( #19161, #7639 ), #39706, .T. ) ;
#47764=FACE_OUTER_BOUND ( 'NONE', #1138, .T. ) ;
#47765=VECTOR ( 'NONE', #1317, 1000.000000000000000 ) ;
#47774=AXIS2_PLACEMENT_3D ( 'NONE', #32412, #40363, #13152 ) ;
#47775=( NAMED_UNIT ( * ) SI_UNIT ( $, .STERADIAN. ) SOLID_ANGLE_UNIT ( ) );
#47778=FACE_OUTER_BOUND ( 'NONE', #46021, .T. ) ;
#47779=ORIENTED_EDGE ( 'NONE', *, *, #5136, .F. ) ;
#47785=EDGE_CURVE ( 'NONE', #15688, #23492, #47343, .T. ) ;
#47786=FACE_OUTER_BOUND ( 'NONE', #19292, .T. ) ;
#47792=CIRCLE ( 'NONE', #44539, 3.749999999999975575 ) ;
#47794=ORIENTED_EDGE ( 'NONE', *, *, #4239, .F. ) ;
#47796=CARTESIAN_POINT ( 'NONE',  ( 356.0000000000000568, 165.0000000000000000, -94.00000000000019895 ) ) ;
#47799=AXIS2_PLACEMENT_3D ( 'NONE', #23060, #38239, #34375 ) ;
#47802=DIRECTION ( 'NONE',  ( 0.000000000000000000, 2.537652627714642000E-15, 1.000000000000000000 ) ) ;
#47810=VECTOR ( 'NONE', #17074, 1000.000000000000000 ) ;
#47818=EDGE_LOOP ( 'NONE', ( #1203, #7345, #37816, #41634 ) ) ;
#47820=DIRECTION ( 'NONE',  ( 4.758098676964954489E-16, 1.000000000000000000, 1.751623080406021339E-46 ) ) ;
#47828=VERTEX_POINT ( 'NONE', #23792 ) ;
#47844=AXIS2_PLACEMENT_3D ( 'NONE', #372, #16016, #15259 ) ;
#47846=DIRECTION ( 'NONE',  ( 1.000000000000000000, 0.000000000000000000, -0.000000000000000000 ) ) ;
#47858=LINE ( 'NONE', #12986, #18089 ) ;
#47862=CARTESIAN_POINT ( 'NONE',  ( 166.9999999999999716, -256.4999999999999432, -339.9999999999998863 ) ) ;
#47863=VECTOR ( 'NONE', #29733, 1000.000000000000000 ) ;
#47869=DIRECTION ( 'NONE',  ( -1.586032892321652236E-16, -1.000000000000000000, -2.288264760618012091E-48 ) ) ;
#47874=DIRECTION ( 'NONE',  ( 1.000000000000000000, 0.000000000000000000, 1.612977847700450206E-50 ) ) ;
#47875=ORIENTED_EDGE ( 'NONE', *, *, #21630, .T. ) ;
#47882=DIRECTION ( 'NONE',  ( 0.000000000000000000, -1.000000000000000000, -3.186989995019654210E-49 ) ) ;
#47894=AXIS2_PLACEMENT_3D ( 'NONE', #10749, #42307, #34370 ) ;
#47912=PLANE ( 'NONE',  #24127 ) ;
#47916=EDGE_CURVE ( 'NONE', #19896, #47246, #21193, .T. ) ;
#47927=AXIS2_PLACEMENT_3D ( 'NONE', #9315, #13405, #24977 ) ;
#47936=ORIENTED_EDGE ( 'NONE', *, *, #9729, .F. ) ;
#47938=CARTESIAN_POINT ( 'NONE',  ( 5.551115123125782702E-14, -180.9999999999999716, 359.9999999999997726 ) ) ;
#47939=EDGE_LOOP ( 'NONE', ( #12645, #34683, #127, #13639 ) ) ;
#47949=DIRECTION ( 'NONE',  ( 1.000000000000000000, 0.000000000000000000, 0.000000000000000000 ) ) ;
#47951=ADVANCED_FACE ( 'NONE', ( #48097, #12979 ), #9143, .T. ) ;
#47957=DIRECTION ( 'NONE',  ( 0.000000000000000000, -1.000000000000000000, 0.000000000000000000 ) ) ;
#47968=ORIENTED_EDGE ( 'NONE', *, *, #24099, .T. ) ;
#47975=FACE_OUTER_BOUND ( 'NONE', #23766, .T. ) ;
#47977=CARTESIAN_POINT ( 'NONE',  ( 0.000000000000000000, 185.0000000000000284, 355.9999999999997726 ) ) ;
#47980=LINE ( 'NONE', #44649, #50222 ) ;
#47983=EDGE_CURVE ( 'NONE', #10796, #6015, #49357, .T. ) ;
#47987=ORIENTED_EDGE ( 'NONE', *, *, #31586, .F. ) ;
#47989=CARTESIAN_POINT ( 'NONE',  ( -5.000000000000000000, -165.1999999999999602, 340.1999999999997044 ) ) ;
#47991=CARTESIAN_POINT ( 'NONE',  ( 344.0000000000000000, -174.9999999999999432, 339.9999999999998295 ) ) ;
#47992=AXIS2_PLACEMENT_3D ( 'NONE', #7219, #26963, #39040 ) ;
#47993=ORIENTED_EDGE ( 'NONE', *, *, #18608, .T. ) ;
#47994=DIRECTION ( 'NONE',  ( -1.586032892321652236E-16, -1.000000000000000000, -6.853681917100419162E-49 ) ) ;
#47996=PLANE ( 'NONE',  #36644 ) ;
#47997=CARTESIAN_POINT ( 'NONE',  ( 343.9999999999999432, -181.0000000000001421, -349.9999999999998863 ) ) ;
#47999=( BOUNDED_CURVE ( )  B_SPLINE_CURVE ( 3, ( #32963, #8838, #20635, #48544 ),
 .UNSPECIFIED., .F., .F. ) 
 B_SPLINE_CURVE_WITH_KNOTS ( ( 4, 4 ),
 ( 1.570796326794903663, 3.141592653589793116 ),
 .UNSPECIFIED. ) 
 CURVE ( )  GEOMETRIC_REPRESENTATION_ITEM ( )  RATIONAL_B_SPLINE_CURVE ( ( 1.000000000000000000, 0.8047378541243667138, 0.8047378541243667138, 1.000000000000000000 ) ) 
 REPRESENTATION_ITEM ( '' )  );
#48007=CARTESIAN_POINT ( 'NONE',  ( 358.0000000000000000, 181.0000000000000284, -356.0000000000001705 ) ) ;
#48009=DIRECTION ( 'NONE',  ( -0.000000000000000000, -1.000000000000000000, -0.000000000000000000 ) ) ;
#48010=DIRECTION ( 'NONE',  ( 0.000000000000000000, 0.000000000000000000, 1.000000000000000000 ) ) ;
#48012=AXIS2_PLACEMENT_3D ( 'NONE', #34221, #10097, #49798 ) ;
#48024=DIRECTION ( 'NONE',  ( 0.000000000000000000, 1.000000000000000000, 6.123233995736766036E-17 ) ) ;
#48026=VECTOR ( 'NONE', #6069, 1000.000000000000000 ) ;
#48030=DIRECTION ( 'NONE',  ( 7.793956916774525800E-48, 0.000000000000000000, -1.000000000000000000 ) ) ;
#48034=EDGE_CURVE ( 'NONE', #32484, #50534, #14502, .T. ) ;
#48035=CARTESIAN_POINT ( 'NONE',  ( 183.0000000000000000, -93.50000000000005684, -340.0000000000001137 ) ) ;
#48042=ADVANCED_FACE ( 'NONE', ( #29651 ), #6806, .T. ) ;
#48046=EDGE_LOOP ( 'NONE', ( #12387, #17052, #11950, #34282 ) ) ;
#48047=VERTEX_POINT ( 'NONE', #41192 ) ;
#48056=AXIS2_PLACEMENT_3D ( 'NONE', #1987, #2731, #9682 ) ;
#48062=ORIENTED_EDGE ( 'NONE', *, *, #15856, .F. ) ;
#48068=ORIENTED_EDGE ( 'NONE', *, *, #37858, .T. ) ;
#48069=EDGE_CURVE ( 'NONE', #9965, #28730, #11758, .T. ) ;
#48074=CARTESIAN_POINT ( 'NONE',  ( 5.551115123125782702E-14, -182.9999999999999716, 355.9999999999997726 ) ) ;
#48077=DIRECTION ( 'NONE',  ( 0.000000000000000000, 0.000000000000000000, -1.000000000000000000 ) ) ;
#48078=EDGE_CURVE ( 'NONE', #26951, #48972, #11278, .T. ) ;
#48082=DIRECTION ( 'NONE',  ( -1.000000000000000000, 0.000000000000000000, 0.000000000000000000 ) ) ;
#48097=FACE_BOUND ( 'NONE', #49503, .T. ) ;
#48099=ORIENTED_EDGE ( 'NONE', *, *, #7333, .F. ) ;
#48101=ORIENTED_EDGE ( 'NONE', *, *, #5889, .T. ) ;
#48114=DIRECTION ( 'NONE',  ( -1.586032892321652236E-16, -1.000000000000000000, -2.288264760618012091E-48 ) ) ;
#48117=EDGE_LOOP ( 'NONE', ( #19893, #38761, #36177, #38848, #33112, #31175, #14462, #2546 ) ) ;
#48121=ADVANCED_FACE ( 'NONE', ( #43170 ), #39586, .T. ) ;
#48132=EDGE_CURVE ( 'NONE', #6887, #29772, #44506, .T. ) ;
#48133=DIRECTION ( 'NONE',  ( 6.203854594147707562E-25, -2.067951531382569187E-25, 1.000000000000000000 ) ) ;
#48135=CARTESIAN_POINT ( 'NONE',  ( 183.0000000000000000, -93.49999999999998579, -340.0000000000001137 ) ) ;
#48139=EDGE_CURVE ( 'NONE', #15830, #11949, #35544, .T. ) ;
#48143=UNCERTAINTY_MEASURE_WITH_UNIT (LENGTH_MEASURE( 1.000000000000000082E-05 ), #34954, 'distance_accuracy_value', 'NONE');
#48153=CARTESIAN_POINT ( 'NONE',  ( 168.9999999999999716, -166.9999999999999432, -350.0000000000001705 ) ) ;
#48155=CARTESIAN_POINT ( 'NONE',  ( 350.0000000000000000, 169.0000000000000000, -342.0000000000001705 ) ) ;
#48163=ORIENTED_EDGE ( 'NONE', *, *, #9821, .T. ) ;
#48166=EDGE_LOOP ( 'NONE', ( #3090, #12122, #14078, #5490 ) ) ;
#48172=DIRECTION ( 'NONE',  ( 0.000000000000000000, 0.000000000000000000, -1.000000000000000000 ) ) ;
#48174=CLOSED_SHELL ( 'NONE', ( #40023, #25865, #46774, #22738, #24966, #11457, #20739, #3859, #48415, #26293, #42685, #40024, #48416, #9571, #18741, #39688, #17423, #31390 ) ) ;
#48176=CARTESIAN_POINT ( 'NONE',  ( 185.0000000000000000, -93.49999999999998579, -350.0000000000001705 ) ) ;
#48179=DIRECTION ( 'NONE',  ( -1.000000000000000000, 0.000000000000000000, -7.793956916774525800E-48 ) ) ;
#48182=DIRECTION ( 'NONE',  ( 6.203854594147707562E-25, -2.067951531382569187E-25, 1.000000000000000000 ) ) ;
#48191=EDGE_CURVE ( 'NONE', #13514, #40964, #47980, .T. ) ;
#48193=LINE ( 'NONE', #8499, #32696 ) ;
#48198=ORIENTED_EDGE ( 'NONE', *, *, #42406, .T. ) ;
#48203=EDGE_CURVE ( 'NONE', #46968, #23694, #25357, .T. ) ;
#48204=LINE ( 'NONE', #4885, #33540 ) ;
#48205=CARTESIAN_POINT ( 'NONE',  ( 168.9999999999999716, -268.4999999999999432, -339.9999999999998863 ) ) ;
#48207=CARTESIAN_POINT ( 'NONE',  ( 181.0000000000000284, -9.999999999999953815, -113.0000000000001563 ) ) ;
#48210=AXIS2_PLACEMENT_3D ( 'NONE', #114, #27567, #27811 ) ;
#48211=CIRCLE ( 'NONE', #28618, 2.000000000000001776 ) ;
#48233=VERTEX_POINT ( 'NONE', #24939 ) ;
#48237=VECTOR ( 'NONE', #8878, 1000.000000000000000 ) ;
#48244=ORIENTED_EDGE ( 'NONE', *, *, #21907, .F. ) ;
#48247=CIRCLE ( 'NONE', #8958, 2.000000000000001776 ) ;
#48248=LINE ( 'NONE', #21862, #37414 ) ;
#48255=VERTEX_POINT ( 'NONE', #29284 ) ;
#48259=CARTESIAN_POINT ( 'NONE',  ( 342.8284271247460993, 167.0000000000001990, -342.0000000000002842 ) ) ;
#48266=CARTESIAN_POINT ( 'NONE',  ( 339.9999999999999432, -169.0000000000001137, -349.9999999999998863 ) ) ;
#48274=FACE_OUTER_BOUND ( 'NONE', #18568, .T. ) ;
#48282=VECTOR ( 'NONE', #34114, 1000.000000000000000 ) ;
#48286=ORIENTED_EDGE ( 'NONE', *, *, #2969, .T. ) ;
#48287=VECTOR ( 'NONE', #6945, 1000.000000000000000 ) ;
#48299=ORIENTED_EDGE ( 'NONE', *, *, #4826, .F. ) ;
#48314=VERTEX_POINT ( 'NONE', #41085 ) ;
#48316=VECTOR ( 'NONE', #37409, 1000.000000000000000 ) ;
#48319=CARTESIAN_POINT ( 'NONE',  ( 164.9999999999999716, -168.9999999999999432, -340.0000000000001137 ) ) ;
#48321=ORIENTED_EDGE ( 'NONE', *, *, #2080, .F. ) ;
#48323=VERTEX_POINT ( 'NONE', #44404 ) ;
#48324=CARTESIAN_POINT ( 'NONE',  ( 164.9999999999999716, 174.9999999999999716, -340.0000000000001137 ) ) ;
#48328=CARTESIAN_POINT ( 'NONE',  ( 168.9999999999999716, -79.49999999999995737, -115.0000000000001563 ) ) ;
#48335=CARTESIAN_POINT ( 'NONE',  ( 168.9999999999999716, -184.9999999999999716, -340.0000000000001705 ) ) ;
#48336=FACE_OUTER_BOUND ( 'NONE', #13815, .T. ) ;
#48350=( GEOMETRIC_REPRESENTATION_CONTEXT ( 3 ) GLOBAL_UNCERTAINTY_ASSIGNED_CONTEXT ( ( #19173 ) ) GLOBAL_UNIT_ASSIGNED_CONTEXT ( ( #49131, #49631, #10178 ) ) REPRESENTATION_CONTEXT ( 'NONE', 'WORKASPACE' ) );
#48355=EDGE_CURVE ( 'NONE', #21998, #9239, #37268, .T. ) ;
#48356=VERTEX_POINT ( 'NONE', #38271 ) ;
#48361=DIRECTION ( 'NONE',  ( -1.586032892321652236E-16, -1.000000000000000000, -2.288264760618012091E-48 ) ) ;
#48366=CARTESIAN_POINT ( 'NONE',  ( 0.000000000000000000, -184.7999999999999545, -340.2000000000001592 ) ) ;
#48372=( NAMED_UNIT ( * ) SI_UNIT ( $, .STERADIAN. ) SOLID_ANGLE_UNIT ( ) );
#48373=ORIENTED_EDGE ( 'NONE', *, *, #50014, .F. ) ;
#48374=ORIENTED_EDGE ( 'NONE', *, *, #10521, .T. ) ;
#48377=DIRECTION ( 'NONE',  ( 0.000000000000000000, 0.000000000000000000, -1.000000000000000000 ) ) ;
#48378=ORIENTED_EDGE ( 'NONE', *, *, #48191, .F. ) ;
#48379=EDGE_CURVE ( 'NONE', #17305, #12755, #4397, .T. ) ;
#48386=DIRECTION ( 'NONE',  ( 0.000000000000000000, 0.000000000000000000, 1.000000000000000000 ) ) ;
#48399=FACE_OUTER_BOUND ( 'NONE', #32327, .T. ) ;
#48409=AXIS2_PLACEMENT_3D ( 'NONE', #37987, #21463, #21974 ) ;
#48410=VERTEX_POINT ( 'NONE', #26192 ) ;
#48413=ORIENTED_EDGE ( 'NONE', *, *, #43412, .F. ) ;
#48415=ADVANCED_FACE ( 'NONE', ( #46660 ), #38515, .T. ) ;
#48416=ADVANCED_FACE ( 'NONE', ( #26435 ), #30052, .T. ) ;
#48418=DIRECTION ( 'NONE',  ( 0.000000000000000000, 0.000000000000000000, 1.000000000000000000 ) ) ;
#48420=VERTEX_POINT ( 'NONE', #50499 ) ;
#48428=EDGE_CURVE ( 'NONE', #1177, #19922, #34660, .T. ) ;
#48433=VERTEX_POINT ( 'NONE', #46413 ) ;
#48446=DIRECTION ( 'NONE',  ( 0.000000000000000000, -1.000000000000000000, 0.000000000000000000 ) ) ;
#48449=AXIS2_PLACEMENT_3D ( 'NONE', #6452, #22352, #14658 ) ;
#48465=DIRECTION ( 'NONE',  ( 4.996003610813203446E-16, 1.000000000000000000, 0.000000000000000000 ) ) ;
#48469=ORIENTED_EDGE ( 'NONE', *, *, #47916, .F. ) ;
#48477=ORIENTED_EDGE ( 'NONE', *, *, #13130, .T. ) ;
#48478=LINE ( 'NONE', #13372, #41753 ) ;
#48482=CARTESIAN_POINT ( 'NONE',  ( 357.9999999999999432, -174.9999999999999716, 355.9999999999998295 ) ) ;
#48488=PLANE ( 'NONE',  #9519 ) ;
#48492=AXIS2_PLACEMENT_3D ( 'NONE', #26573, #34802, #34533 ) ;
#48495=EDGE_LOOP ( 'NONE', ( #35784, #6843, #1782, #42581 ) ) ;
#48497=EDGE_CURVE ( 'NONE', #47734, #27082, #28966, .T. ) ;
#48499=ORIENTED_EDGE ( 'NONE', *, *, #2946, .F. ) ;
#48509=CARTESIAN_POINT ( 'NONE',  ( 168.9999999999999716, -9.999999999999953815, -350.0000000000001705 ) ) ;
#48512=ORIENTED_EDGE ( 'NONE', *, *, #17196, .F. ) ;
#48517=CARTESIAN_POINT ( 'NONE',  ( 0.000000000000000000, 169.0000000000000000, 343.9999999999997726 ) ) ;
#48520=VECTOR ( 'NONE', #7042, 1000.000000000000000 ) ;
#48522=ORIENTED_EDGE ( 'NONE', *, *, #10583, .T. ) ;
#48526=LINE ( 'NONE', #13413, #46242 ) ;
#48535=LINE ( 'NONE', #5982, #41384 ) ;
#48539=EDGE_CURVE ( 'NONE', #38121, #21871, #7713, .T. ) ;
#48544=CARTESIAN_POINT ( 'NONE',  ( 356.0000000000000000, -165.0000000000001137, -340.0000000000002842 ) ) ;
#48547=ORIENTED_EDGE ( 'NONE', *, *, #28133, .F. ) ;
#48550=EDGE_CURVE ( 'NONE', #48323, #16118, #37232, .T. ) ;
#48553=VERTEX_POINT ( 'NONE', #12303 ) ;
#48554=CARTESIAN_POINT ( 'NONE',  ( 185.0000000000000000, -168.9999999999999432, -350.0000000000001705 ) ) ;
#48556=CARTESIAN_POINT ( 'NONE',  ( 181.0000000000000000, -7.999999999999952038, -350.0000000000001705 ) ) ;
#48557=AXIS2_PLACEMENT_3D ( 'NONE', #27647, #11236, #15585 ) ;
#48558=DIRECTION ( 'NONE',  ( -0.000000000000000000, -1.544785076050074834E-48, -1.000000000000000000 ) ) ;
#48569=ORIENTED_EDGE ( 'NONE', *, *, #11722, .F. ) ;
#48575=DIRECTION ( 'NONE',  ( 2.220446049250312588E-16, 0.7071067811865475727, 0.7071067811865474617 ) ) ;
#48577=DIRECTION ( 'NONE',  ( 0.000000000000000000, -1.000000000000000000, 2.969158215481698263E-48 ) ) ;
#48580=DIRECTION ( 'NONE',  ( 1.000000000000000000, 0.000000000000000000, 0.000000000000000000 ) ) ;
#48589=DIRECTION ( 'NONE',  ( -1.000000000000000000, 0.000000000000000000, 0.000000000000000000 ) ) ;
#48597=( BOUNDED_CURVE ( )  B_SPLINE_CURVE ( 3, ( #17982, #36768, #33656, #45414 ),
 .UNSPECIFIED., .F., .F. ) 
 B_SPLINE_CURVE_WITH_KNOTS ( ( 4, 4 ),
 ( 3.169317492284578310E-16, 1.570796326794938302 ),
 .UNSPECIFIED. ) 
 CURVE ( )  GEOMETRIC_REPRESENTATION_ITEM ( )  RATIONAL_B_SPLINE_CURVE ( ( 1.000000000000000000, 0.8047378541243551675, 0.8047378541243551675, 1.000000000000000000 ) ) 
 REPRESENTATION_ITEM ( '' )  );
#48607=LINE ( 'NONE', #29403, #14434 ) ;
#48614=EDGE_CURVE ( 'NONE', #28535, #27142, #15859, .T. ) ;
#48628=CARTESIAN_POINT ( 'NONE',  ( 341.9999999999999432, -181.0000000000001705, -356.0000000000003411 ) ) ;
#48652=CIRCLE ( 'NONE', #34816, 4.000000000000003553 ) ;
#48656=DIRECTION ( 'NONE',  ( 0.000000000000000000, -4.687818848539279227E-49, 1.000000000000000000 ) ) ;
#48658=ORIENTED_EDGE ( 'NONE', *, *, #23710, .F. ) ;
#48661=ORIENTED_EDGE ( 'NONE', *, *, #18608, .F. ) ;
#48667=CYLINDRICAL_SURFACE ( 'NONE', #8987, 4.000000000000003553 ) ;
#48673=CARTESIAN_POINT ( 'NONE',  ( 340.0000000000000568, 165.0000000000000000, 355.9999999999997726 ) ) ;
#48683=AXIS2_PLACEMENT_3D ( 'NONE', #26238, #2616, #42376 ) ;
#48685=ORIENTED_EDGE ( 'NONE', *, *, #32396, .T. ) ;
#48686=DIRECTION ( 'NONE',  ( 1.000000000000000000, 0.000000000000000000, 0.000000000000000000 ) ) ;
#48716=VECTOR ( 'NONE', #29463, 1000.000000000000000 ) ;
#48718=VERTEX_POINT ( 'NONE', #34098 ) ;
#48730=ADVANCED_FACE ( 'NONE', ( #14318 ), #23026, .F. ) ;
#48732=DIRECTION ( 'NONE',  ( 1.000000000000000000, 0.000000000000000000, -1.860490536778032451E-50 ) ) ;
#48733=VECTOR ( 'NONE', #48577, 1000.000000000000000 ) ;
#48734=CARTESIAN_POINT ( 'NONE',  ( 340.0000000000000568, 169.0000000000000284, 343.9999999999998295 ) ) ;
#48740=PRODUCT_DEFINITION_FORMATION_WITH_SPECIFIED_SOURCE ( 'ANY', '', #43383, .NOT_KNOWN. ) ;
#48742=FACE_OUTER_BOUND ( 'NONE', #16514, .T. ) ;
#48751=CARTESIAN_POINT ( 'NONE',  ( 340.0000000000000568, 169.0000000000000000, 343.9999999999998295 ) ) ;
#48754=FACE_OUTER_BOUND ( 'NONE', #37733, .T. ) ;
#48755=DIRECTION ( 'NONE',  ( 1.000000000000000000, 0.000000000000000000, 0.000000000000000000 ) ) ;
#48769=LINE ( 'NONE', #10328, #2099 ) ;
#48770=VERTEX_POINT ( 'NONE', #42521 ) ;
#48777=EDGE_CURVE ( 'NONE', #48433, #22911, #18149, .T. ) ;
#48780=STYLED_ITEM('',(#50747),#21477);
#48787=VECTOR ( 'NONE', #7362, 1000.000000000000000 ) ;
#48789=EDGE_CURVE ( 'NONE', #21707, #218, #701, .T. ) ;
#48790=ORIENTED_EDGE ( 'NONE', *, *, #49385, .T. ) ;
#48791=CYLINDRICAL_SURFACE ( 'NONE', #30269, 4.000000000000003553 ) ;
#48795=EDGE_CURVE ( 'NONE', #21143, #13147, #46597, .T. ) ;
#48796=CARTESIAN_POINT ( 'NONE',  ( 185.0000000000000000, -164.9999999999999432, 343.9999999999998863 ) ) ;
#48797=VECTOR ( 'NONE', #5871, 1000.000000000000000 ) ;
#48801=PLANE ( 'NONE',  #45042 ) ;
#48804=ORIENTED_EDGE ( 'NONE', *, *, #46939, .T. ) ;
#48807=VERTEX_POINT ( 'NONE', #43288 ) ;
#48818=VERTEX_POINT ( 'NONE', #4789 ) ;
#48821=VERTEX_POINT ( 'NONE', #12246 ) ;
#48824=CARTESIAN_POINT ( 'NONE',  ( 339.9999999999998863, -181.0000000000001421, -349.9999999999998863 ) ) ;
#48827=DIRECTION ( 'NONE',  ( 1.000000000000000000, 0.000000000000000000, 0.000000000000000000 ) ) ;
#48832=VECTOR ( 'NONE', #8041, 1000.000000000000000 ) ;
#48840=CARTESIAN_POINT ( 'NONE',  ( 183.0000000000000000, -180.9999999999999716, -350.0000000000001705 ) ) ;
#48841=EDGE_CURVE ( 'NONE', #49685, #47734, #462, .T. ) ;
#48846=PLANE ( 'NONE',  #27822 ) ;
#48855=DIRECTION ( 'NONE',  ( -1.586032880504786307E-16, 1.654361225106055350E-24, -1.000000000000000000 ) ) ;
#48859=CARTESIAN_POINT ( 'NONE',  ( 355.9999999999999432, -183.0000000000001421, -358.0000000000003411 ) ) ;
#48862=ORIENTED_EDGE ( 'NONE', *, *, #18598, .T. ) ;
#48868=EDGE_CURVE ( 'NONE', #11426, #48770, #25751, .T. ) ;
#48870=CARTESIAN_POINT ( 'NONE',  ( 359.9999999999999432, -180.9999999999999716, 355.9999999999998295 ) ) ;
#48874=DIRECTION ( 'NONE',  ( -1.000000000000000000, 0.000000000000000000, -7.793956916774525800E-48 ) ) ;
#48879=DIRECTION ( 'NONE',  ( -1.000000000000000000, 0.000000000000000000, 0.000000000000000000 ) ) ;
#48880=CARTESIAN_POINT ( 'NONE',  ( 357.1715728752538439, -183.0000000000001421, 358.0000000000000568 ) ) ;
#48894=CARTESIAN_POINT ( 'NONE',  ( 0.000000000000000000, 169.0000000000000000, 359.9999999999997726 ) ) ;
#48895=ORIENTED_EDGE ( 'NONE', *, *, #37159, .F. ) ;
#48897=DIRECTION ( 'NONE',  ( -1.000000000000000000, 0.000000000000000000, -1.612977847700450206E-50 ) ) ;
#48899=CYLINDRICAL_SURFACE ( 'NONE', #14375, 4.000000000000003553 ) ;
#48916=ORIENTED_EDGE ( 'NONE', *, *, #2270, .F. ) ;
#48921=CYLINDRICAL_SURFACE ( 'NONE', #10980, 4.000000000000003553 ) ;
#48924=LINE ( 'NONE', #25383, #45248 ) ;
#48926=DIRECTION ( 'NONE',  ( -1.000000000000000000, 0.000000000000000000, -7.793956916774525800E-48 ) ) ;
#48930=CARTESIAN_POINT ( 'NONE',  ( 181.0000000000000000, -272.4999999999999432, -341.9999999999999432 ) ) ;
#48932=VERTEX_POINT ( 'NONE', #7913 ) ;
#48934=LINE ( 'NONE', #36723, #13535 ) ;
#48943=DIRECTION ( 'NONE',  ( 1.333906992743555050E-23, -1.000000000000000000, 0.000000000000000000 ) ) ;
#48951=EDGE_CURVE ( 'NONE', #47413, #2629, #35377, .T. ) ;
#48959=CARTESIAN_POINT ( 'NONE',  ( 358.0000000000001137, 181.0000000000000284, 355.9999999999998295 ) ) ;
#48963=ORIENTED_EDGE ( 'NONE', *, *, #5480, .F. ) ;
#48964=LINE ( 'NONE', #22074, #16421 ) ;
#48972=VERTEX_POINT ( 'NONE', #24815 ) ;
#48975=DIRECTION ( 'NONE',  ( 0.000000000000000000, 1.000000000000000000, 0.000000000000000000 ) ) ;
#48976=CARTESIAN_POINT ( 'NONE',  ( 343.9999999999999432, -185.0000000000001421, -349.9999999999999432 ) ) ;
#48978=ORIENTED_EDGE ( 'NONE', *, *, #36405, .T. ) ;
#48979=EDGE_CURVE ( 'NONE', #1426, #5304, #44527, .T. ) ;
#48983=EDGE_CURVE ( 'NONE', #8311, #269, #32267, .T. ) ;
#48984=EDGE_CURVE ( 'NONE', #8311, #4051, #13751, .T. ) ;
#48987=DIRECTION ( 'NONE',  ( 0.000000000000000000, -1.000000000000000000, 0.000000000000000000 ) ) ;
#48988=ORIENTED_EDGE ( 'NONE', *, *, #24201, .T. ) ;
#48990=ADVANCED_FACE ( 'NONE', ( #1472 ), #12753, .F. ) ;
#48993=ORIENTED_EDGE ( 'NONE', *, *, #35625, .F. ) ;
#48996=DIRECTION ( 'NONE',  ( -1.586032880504786307E-16, 1.654361225106055350E-24, -1.000000000000000000 ) ) ;
#49006=CIRCLE ( 'NONE', #41665, 2.000000000000001776 ) ;
#49010=ORIENTED_EDGE ( 'NONE', *, *, #808, .F. ) ;
#49014=EDGE_CURVE ( 'NONE', #38360, #31812, #9408, .T. ) ;
#49027=EDGE_LOOP ( 'NONE', ( #37200, #34724, #46488, #44294 ) ) ;
#49031=CARTESIAN_POINT ( 'NONE',  ( 349.9999999999999432, -168.9999999999999432, 341.9999999999997726 ) ) ;
#49033=ADVANCED_FACE ( 'NONE', ( #21448 ), #45283, .F. ) ;
#49035=VECTOR ( 'NONE', #7501, 1000.000000000000000 ) ;
#49039=EDGE_CURVE ( 'NONE', #24656, #10537, #10916, .T. ) ;
#49040=LINE ( 'NONE', #2637, #26216 ) ;
#49042=VECTOR ( 'NONE', #4565, 1000.000000000000000 ) ;
#49044=AXIS2_PLACEMENT_3D ( 'NONE', #12791, #35909, #24360 ) ;
#49047=ORIENTED_EDGE ( 'NONE', *, *, #12533, .T. ) ;
#49062=EDGE_CURVE ( 'NONE', #7227, #3886, #45537, .T. ) ;
#49063=( BOUNDED_CURVE ( )  B_SPLINE_CURVE ( 3, ( #7545, #34238, #22673, #38348 ),
 .UNSPECIFIED., .F., .F. ) 
 B_SPLINE_CURVE_WITH_KNOTS ( ( 4, 4 ),
 ( 3.141592653589794004, 4.712388980384689674 ),
 .UNSPECIFIED. ) 
 CURVE ( )  GEOMETRIC_REPRESENTATION_ITEM ( )  RATIONAL_B_SPLINE_CURVE ( ( 1.000000000000000000, 0.8047378541243652705, 0.8047378541243652705, 1.000000000000000000 ) ) 
 REPRESENTATION_ITEM ( '' )  );
#49074=ORIENTED_EDGE ( 'NONE', *, *, #34056, .T. ) ;
#49076=PLANE ( 'NONE',  #43611 ) ;
#49078=ORIENTED_EDGE ( 'NONE', *, *, #7616, .T. ) ;
#49082=LINE ( 'NONE', #48328, #40884 ) ;
#49084=EDGE_CURVE ( 'NONE', #23039, #44300, #20115, .T. ) ;
#49088=VECTOR ( 'NONE', #14589, 1000.000000000000000 ) ;
#49089=CARTESIAN_POINT ( 'NONE',  ( 185.0000000000000000, -5.999999999999950262, -350.0000000000001705 ) ) ;
#49098=DIRECTION ( 'NONE',  ( 0.000000000000000000, 5.664403186863042467E-17, 1.000000000000000000 ) ) ;
#49102=CARTESIAN_POINT ( 'NONE',  ( 0.000000000000000000, 183.0000000000000284, 343.9999999999997726 ) ) ;
#49105=VERTEX_POINT ( 'NONE', #14513 ) ;
#49110=VECTOR ( 'NONE', #16155, 1000.000000000000000 ) ;
#49118=CIRCLE ( 'NONE', #8233, 2.000000000000001776 ) ;
#49128=ORIENTED_EDGE ( 'NONE', *, *, #46263, .T. ) ;
#49129=FACE_OUTER_BOUND ( 'NONE', #18127, .T. ) ;
#49131=( LENGTH_UNIT ( ) NAMED_UNIT ( * ) SI_UNIT ( .MILLI., .METRE. ) );
#49141=DIRECTION ( 'NONE',  ( 0.000000000000000000, 0.000000000000000000, 1.000000000000000000 ) ) ;
#49144=FACE_OUTER_BOUND ( 'NONE', #22222, .T. ) ;
#49149=DIRECTION ( 'NONE',  ( -1.000000000000000000, 0.000000000000000000, 0.000000000000000000 ) ) ;
#49150=AXIS2_PLACEMENT_3D ( 'NONE', #4357, #11292, #26937 ) ;
#49156=VECTOR ( 'NONE', #14810, 1000.000000000000000 ) ;
#49158=EDGE_CURVE ( 'NONE', #7906, #28175, #15779, .T. ) ;
#49159=ORIENTED_EDGE ( 'NONE', *, *, #4469, .F. ) ;
#49167=ORIENTED_EDGE ( 'NONE', *, *, #27143, .F. ) ;
#49169=EDGE_LOOP ( 'NONE', ( #1622, #7320, #30908, #27863 ) ) ;
#49174=DIRECTION ( 'NONE',  ( 0.000000000000000000, 0.000000000000000000, -1.000000000000000000 ) ) ;
#49180=ORIENTED_EDGE ( 'NONE', *, *, #36731, .T. ) ;
#49181=CARTESIAN_POINT ( 'NONE',  ( 181.0000000000000284, 2.775557561562891351E-14, -99.00000000000014211 ) ) ;
#49185=CARTESIAN_POINT ( 'NONE',  ( 350.0000000000000000, -184.9999999999999716, -344.0000000000001705 ) ) ;
#49186=AXIS2_PLACEMENT_3D ( 'NONE', #37819, #14176, #46463 ) ;
#49193=CARTESIAN_POINT ( 'NONE',  ( 343.9999999999999432, -167.0000000000000853, -342.0000000000002842 ) ) ;
#49198=ORIENTED_EDGE ( 'NONE', *, *, #15905, .F. ) ;
#49204=CYLINDRICAL_SURFACE ( 'NONE', #9253, 2.000000000000001776 ) ;
#49211=DIRECTION ( 'NONE',  ( 0.000000000000000000, 0.000000000000000000, -1.000000000000000000 ) ) ;
#49223=CARTESIAN_POINT ( 'NONE',  ( 355.9999999999999432, -185.0000000000000284, 359.9999999999998295 ) ) ;
#49229=VECTOR ( 'NONE', #4673, 1000.000000000000000 ) ;
#49236=CARTESIAN_POINT ( 'NONE',  ( 169.0000000000000284, 175.0000000000000284, 341.9999999999998863 ) ) ;
#49245=VERTEX_POINT ( 'NONE', #35826 ) ;
#49247=EDGE_CURVE ( 'NONE', #14517, #11426, #11429, .T. ) ;
#49249=AXIS2_PLACEMENT_3D ( 'NONE', #46559, #47324, #35586 ) ;
#49252=DIRECTION ( 'NONE',  ( -4.758098676964954489E-16, -1.000000000000000000, -1.751623080406021339E-46 ) ) ;
#49254=LINE ( 'NONE', #30571, #37286 ) ;
#49255=LINE ( 'NONE', #8855, #9075 ) ;
#49263=DIRECTION ( 'NONE',  ( 0.000000000000000000, 1.000000000000000000, 0.000000000000000000 ) ) ;
#49272=CARTESIAN_POINT ( 'NONE',  ( 183.0000000000000000, -81.49999999999995737, -115.0000000000001563 ) ) ;
#49276=CYLINDRICAL_SURFACE ( 'NONE', #9164, 4.000000000000003553 ) ;
#49280=ADVANCED_FACE ( 'NONE', ( #43980 ), #5246, .F. ) ;
#49288=AXIS2_PLACEMENT_3D ( 'NONE', #33116, #1799, #13590 ) ;
#49291=AXIS2_PLACEMENT_3D ( 'NONE', #24137, #23872, #19242 ) ;
#49297=VERTEX_POINT ( 'NONE', #12690 ) ;
#49298=VERTEX_POINT ( 'NONE', #1907 ) ;
#49305=ORIENTED_EDGE ( 'NONE', *, *, #50285, .T. ) ;
#49312=AXIS2_PLACEMENT_3D ( 'NONE', #47553, #33723, #33472 ) ;
#49316=ORIENTED_EDGE ( 'NONE', *, *, #11822, .F. ) ;
#49317=VECTOR ( 'NONE', #50654, 1000.000000000000000 ) ;
#49320=VECTOR ( 'NONE', #22358, 1000.000000000000000 ) ;
#49322=EDGE_LOOP ( 'NONE', ( #24364, #25387, #47450, #8450 ) ) ;
#49324=ORIENTED_EDGE ( 'NONE', *, *, #5550, .F. ) ;
#49334=CARTESIAN_POINT ( 'NONE',  ( 181.0000000000000284, -174.9999999999999716, -111.0000000000001563 ) ) ;
#49342=EDGE_CURVE ( 'NONE', #19122, #8719, #1163, .T. ) ;
#49347=DIRECTION ( 'NONE',  ( 2.958228394578793832E-31, 0.000000000000000000, 1.000000000000000000 ) ) ;
#49354=PLANE ( 'NONE',  #2703 ) ;
#49357=LINE ( 'NONE', #39089, #14190 ) ;
#49363=( GEOMETRIC_REPRESENTATION_CONTEXT ( 3 ) GLOBAL_UNCERTAINTY_ASSIGNED_CONTEXT ( ( #11700 ) ) GLOBAL_UNIT_ASSIGNED_CONTEXT ( ( #951, #8143, #42750 ) ) REPRESENTATION_CONTEXT ( 'NONE', 'WORKASPACE' ) );
#49364=DIRECTION ( 'NONE',  ( -1.000000000000000000, 0.000000000000000000, 0.000000000000000000 ) ) ;
#49367=ADVANCED_FACE ( 'NONE', ( #40905 ), #6270, .F. ) ;
#49372=ORIENTED_EDGE ( 'NONE', *, *, #8408, .T. ) ;
#49385=EDGE_CURVE ( 'NONE', #19838, #21347, #37832, .T. ) ;
#49393=VECTOR ( 'NONE', #44085, 1000.000000000000000 ) ;
#49394=EDGE_CURVE ( 'NONE', #6937, #20029, #45974, .T. ) ;
#49395=DIRECTION ( 'NONE',  ( 0.000000000000000000, 1.000000000000000000, 0.000000000000000000 ) ) ;
#49397=( NAMED_UNIT ( * ) SI_UNIT ( $, .STERADIAN. ) SOLID_ANGLE_UNIT ( ) );
#49401=FACE_OUTER_BOUND ( 'NONE', #25265, .T. ) ;
#49410=ADVANCED_FACE ( 'NONE', ( #14710 ), #13696, .T. ) ;
#49411=FACE_OUTER_BOUND ( 'NONE', #46302, .T. ) ;
#49412=FACE_OUTER_BOUND ( 'NONE', #5350, .T. ) ;
#49425=ORIENTED_EDGE ( 'NONE', *, *, #16129, .F. ) ;
#49428=ORIENTED_EDGE ( 'NONE', *, *, #12796, .F. ) ;
#49435=DIRECTION ( 'NONE',  ( 0.000000000000000000, 1.000000000000000000, 1.544785076050074834E-48 ) ) ;
#49436=ORIENTED_EDGE ( 'NONE', *, *, #17121, .T. ) ;
#49446=ORIENTED_EDGE ( 'NONE', *, *, #18899, .F. ) ;
#49450=EDGE_LOOP ( 'NONE', ( #36279, #47252, #25313, #9741 ) ) ;
#49471=CIRCLE ( 'NONE', #5275, 2.000000000000001776 ) ;
#49489=( BOUNDED_CURVE ( )  B_SPLINE_CURVE ( 3, ( #564, #15182, #23385, #8005 ),
 .UNSPECIFIED., .F., .F. ) 
 B_SPLINE_CURVE_WITH_KNOTS ( ( 4, 4 ),
 ( 4.712388980384693227, 6.283185307179586232 ),
 .UNSPECIFIED. ) 
 CURVE ( )  GEOMETRIC_REPRESENTATION_ITEM ( )  RATIONAL_B_SPLINE_CURVE ( ( 1.000000000000000000, 0.8047378541243658256, 0.8047378541243658256, 1.000000000000000000 ) ) 
 REPRESENTATION_ITEM ( '' )  );
#49494=AXIS2_PLACEMENT_3D ( 'NONE', #41946, #27052, #34257 ) ;
#49498=ORIENTED_EDGE ( 'NONE', *, *, #875, .F. ) ;
#49502=CARTESIAN_POINT ( 'NONE',  ( 339.9999999999999432, 169.0000000000001705, -344.0000000000002842 ) ) ;
#49503=EDGE_LOOP ( 'NONE', ( #505, #13913, #12183, #5185, #37598, #6638, #48378, #16470 ) ) ;
#49506=CARTESIAN_POINT ( 'NONE',  ( 183.0000000000000284, 2.775557561562891351E-14, -99.00000000000014211 ) ) ;
#49511=CARTESIAN_POINT ( 'NONE',  ( 339.9999999999999432, 181.0000000000002274, -356.0000000000003411 ) ) ;
#49513=ORIENTED_EDGE ( 'NONE', *, *, #34064, .F. ) ;
#49523=LINE ( 'NONE', #29325, #35696 ) ;
#49524=FACE_OUTER_BOUND ( 'NONE', #45545, .T. ) ;
#49529=CARTESIAN_POINT ( 'NONE',  ( 356.0000000000000000, -174.9999999999999147, 343.9999999999998295 ) ) ;
#49530=DIRECTION ( 'NONE',  ( 1.000000000000000000, -3.172065784643302499E-16, -1.942330104924128867E-32 ) ) ;
#49538=CARTESIAN_POINT ( 'NONE',  ( 0.000000000000000000, 181.0000000000000284, 357.9999999999997726 ) ) ;
#49547=DIRECTION ( 'NONE',  ( -0.000000000000000000, -1.000000000000000000, 2.537652627714643577E-15 ) ) ;
#49561=ORIENTED_EDGE ( 'NONE', *, *, #45852, .T. ) ;
#49562=AXIS2_PLACEMENT_3D ( 'NONE', #42369, #34443, #33439 ) ;
#49570=DIRECTION ( 'NONE',  ( 0.000000000000000000, -1.000000000000000000, 0.000000000000000000 ) ) ;
#49581=CARTESIAN_POINT ( 'NONE',  ( 183.0000000000000000, -168.9999999999999432, -340.0000000000001705 ) ) ;
#49585=EDGE_LOOP ( 'NONE', ( #11827, #208, #46310, #34528 ) ) ;
#49587=PLANE ( 'NONE',  #37170 ) ;
#49606=LINE ( 'NONE', #22706, #38937 ) ;
#49607=ADVANCED_FACE ( 'NONE', ( #35244 ), #31131, .F. ) ;
#49612=CARTESIAN_POINT ( 'NONE',  ( 341.9999999999999432, -168.9999999999999147, 343.9999999999998295 ) ) ;
#49617=ORIENTED_EDGE ( 'NONE', *, *, #808, .T. ) ;
#49629=CIRCLE ( 'NONE', #20199, 4.000000000000003553 ) ;
#49631=( NAMED_UNIT ( * ) PLANE_ANGLE_UNIT ( ) SI_UNIT ( $, .RADIAN. ) );
#49637=CARTESIAN_POINT ( 'NONE',  ( 0.000000000000000000, -184.7999999999999545, -340.2000000000001592 ) ) ;
#49644=CARTESIAN_POINT ( 'NONE',  ( 360.0000000000000568, 183.3431457505076310, 358.3431457505075741 ) ) ;
#49649=( BOUNDED_CURVE ( )  B_SPLINE_CURVE ( 3, ( #29148, #21685, #13483, #2199 ),
 .UNSPECIFIED., .F., .F. ) 
 B_SPLINE_CURVE_WITH_KNOTS ( ( 4, 4 ),
 ( 4.712388980384700332, 6.283185307179586232 ),
 .UNSPECIFIED. ) 
 CURVE ( )  GEOMETRIC_REPRESENTATION_ITEM ( )  RATIONAL_B_SPLINE_CURVE ( ( 1.000000000000000000, 0.8047378541243676020, 0.8047378541243676020, 1.000000000000000000 ) ) 
 REPRESENTATION_ITEM ( '' )  );
#49652=ADVANCED_FACE ( 'NONE', ( #26770 ), #19314, .F. ) ;
#49653=AXIS2_PLACEMENT_3D ( 'NONE', #9533, #17488, #29039 ) ;
#49654=DIRECTION ( 'NONE',  ( 2.958228394578793832E-31, 0.000000000000000000, 1.000000000000000000 ) ) ;
#49664=VERTEX_POINT ( 'NONE', #6378 ) ;
#49667=VERTEX_POINT ( 'NONE', #32645 ) ;
#49668=CARTESIAN_POINT ( 'NONE',  ( 356.0000000000000568, 175.0000000000000284, -90.00000000000018474 ) ) ;
#49670=CARTESIAN_POINT ( 'NONE',  ( 349.9999999999999432, -182.9999999999999716, 343.9999999999997726 ) ) ;
#49674=EDGE_LOOP ( 'NONE', ( #41463, #41755, #47516, #7212 ) ) ;
#49680=DIRECTION ( 'NONE',  ( 0.000000000000000000, 5.664403186863042467E-17, 1.000000000000000000 ) ) ;
#49681=ADVANCED_FACE ( 'NONE', ( #32143 ), #9978, .T. ) ;
#49685=VERTEX_POINT ( 'NONE', #28539 ) ;
#49686=AXIS2_PLACEMENT_3D ( 'NONE', #49807, #45978, #10860 ) ;
#49690=EDGE_CURVE ( 'NONE', #7855, #25186, #42983, .T. ) ;
#49700=DIRECTION ( 'NONE',  ( -1.586032892321651989E-16, 3.736034562988530447E-32, -1.000000000000000000 ) ) ;
#49701=ORIENTED_EDGE ( 'NONE', *, *, #42760, .F. ) ;
#49704=CARTESIAN_POINT ( 'NONE',  ( 0.000000000000000000, -184.7999999999999545, 340.1999999999997044 ) ) ;
#49709=VERTEX_POINT ( 'NONE', #44169 ) ;
#49713=CARTESIAN_POINT ( 'NONE',  ( 183.0000000000000000, -93.50000000000005684, -115.0000000000001563 ) ) ;
#49715=EDGE_CURVE ( 'NONE', #55, #48047, #48652, .T. ) ;
#49717=FACE_OUTER_BOUND ( 'NONE', #25119, .T. ) ;
#49718=ORIENTED_EDGE ( 'NONE', *, *, #27130, .F. ) ;
#49726=VERTEX_POINT ( 'NONE', #28033 ) ;
#49732=CARTESIAN_POINT ( 'NONE',  ( 168.9999999999999716, -174.9999999999999716, -342.0000000000001137 ) ) ;
#49733=VERTEX_POINT ( 'NONE', #39858 ) ;
#49742=ORIENTED_EDGE ( 'NONE', *, *, #37699, .F. ) ;
#49752=VECTOR ( 'NONE', #46751, 1000.000000000000000 ) ;
#49753=EDGE_CURVE ( 'NONE', #30152, #38030, #10234, .T. ) ;
#49764=EDGE_CURVE ( 'NONE', #40720, #21347, #3026, .T. ) ;
#49767=ORIENTED_EDGE ( 'NONE', *, *, #4065, .T. ) ;
#49771=VECTOR ( 'NONE', #38673, 1000.000000000000000 ) ;
#49781=VERTEX_POINT ( 'NONE', #49929 ) ;
#49798=DIRECTION ( 'NONE',  ( 0.000000000000000000, -0.000000000000000000, 1.000000000000000000 ) ) ;
#49805=DIRECTION ( 'NONE',  ( 0.000000000000000000, 0.000000000000000000, 1.000000000000000000 ) ) ;
#49807=CARTESIAN_POINT ( 'NONE',  ( 169.0000000000000000, -174.9999999999999716, -95.00000000000014211 ) ) ;
#49808=ORIENTED_EDGE ( 'NONE', *, *, #296, .T. ) ;
#49809=CLOSED_SHELL ( 'NONE', ( #3234, #19972, #40269, #36879, #46165, #3042, #6405, #27408 ) ) ;
#49816=EDGE_CURVE ( 'NONE', #9207, #1177, #10212, .T. ) ;
#49817=( LENGTH_UNIT ( ) NAMED_UNIT ( * ) SI_UNIT ( .MILLI., .METRE. ) );
#49818=CARTESIAN_POINT ( 'NONE',  ( 356.0000000000001137, -166.9999999999999432, 341.9999999999998295 ) ) ;
#49821=ORIENTED_EDGE ( 'NONE', *, *, #44516, .F. ) ;
#49823=ORIENTED_EDGE ( 'NONE', *, *, #48379, .F. ) ;
#49825=LINE ( 'NONE', #30137, #25130 ) ;
#49828=VERTEX_POINT ( 'NONE', #42529 ) ;
#49830=PLANE ( 'NONE',  #2355 ) ;
#49832=CIRCLE ( 'NONE', #16317, 4.000000000000003553 ) ;
#49835=VECTOR ( 'NONE', #7230, 1000.000000000000000 ) ;
#49836=VECTOR ( 'NONE', #27410, 1000.000000000000000 ) ;
#49837=DIRECTION ( 'NONE',  ( -1.000000000000000000, 1.331116318405244905E-23, 4.755310728521421461E-16 ) ) ;
#49846=DIRECTION ( 'NONE',  ( 3.172065745548403743E-16, 1.000000000000000000, 0.000000000000000000 ) ) ;
#49851=CARTESIAN_POINT ( 'NONE',  ( 341.9999999999999432, -171.9999999999999147, -347.0000000000001137 ) ) ;
#49858=VERTEX_POINT ( 'NONE', #6633 ) ;
#49860=CARTESIAN_POINT ( 'NONE',  ( 165.0000000000000000, -174.9999999999999716, -99.00000000000014211 ) ) ;
#49864=AXIS2_PLACEMENT_3D ( 'NONE', #15007, #23721, #38368 ) ;
#49865=DIRECTION ( 'NONE',  ( 0.000000000000000000, -1.000000000000000000, 0.000000000000000000 ) ) ;
#49870=FACE_OUTER_BOUND ( 'NONE', #31125, .T. ) ;
#49871=VECTOR ( 'NONE', #14013, 1000.000000000000000 ) ;
#49873=AXIS2_PLACEMENT_3D ( 'NONE', #23585, #50481, #15631 ) ;
#49877=EDGE_LOOP ( 'NONE', ( #26078, #11572, #7512, #17152 ) ) ;
#49880=VECTOR ( 'NONE', #49547, 1000.000000000000000 ) ;
#49882=DIRECTION ( 'NONE',  ( -0.000000000000000000, 1.000000000000000000, 0.000000000000000000 ) ) ;
#49888=CARTESIAN_POINT ( 'NONE',  ( 183.0000000000000000, -272.4999999999999432, -356.0000000000001705 ) ) ;
#49897=ADVANCED_FACE ( 'NONE', ( #26642 ), #37957, .F. ) ;
#49900=CARTESIAN_POINT ( 'NONE',  ( 339.9999999999999432, -165.0000000000001137, -94.00000000000019895 ) ) ;
#49901=AXIS2_PLACEMENT_3D ( 'NONE', #38686, #15833, #39197 ) ;
#49902=EDGE_CURVE ( 'NONE', #49105, #11132, #7145, .T. ) ;
#49908=ORIENTED_EDGE ( 'NONE', *, *, #48984, .T. ) ;
#49929=CARTESIAN_POINT ( 'NONE',  ( 343.9999999999996589, -165.0000000000001137, -108.0000000000002132 ) ) ;
#49933=EDGE_CURVE ( 'NONE', #50534, #25569, #23810, .T. ) ;
#49942=EDGE_CURVE ( 'NONE', #22449, #48410, #16610, .T. ) ;
#49945=ORIENTED_EDGE ( 'NONE', *, *, #47745, .F. ) ;
#49966=EDGE_LOOP ( 'NONE', ( #6491, #41054, #49316, #19308 ) ) ;
#49981=EDGE_CURVE ( 'NONE', #39875, #32721, #2834, .T. ) ;
#49985=ADVANCED_FACE ( 'NONE', ( #4312 ), #27405, .T. ) ;
#49987=VECTOR ( 'NONE', #35995, 1000.000000000000000 ) ;
#49989=DIRECTION ( 'NONE',  ( 1.654361225106055350E-24, 1.654361225106055350E-24, -1.000000000000000000 ) ) ;
#50000=EDGE_CURVE ( 'NONE', #48420, #3658, #35381, .T. ) ;
#50002=DIRECTION ( 'NONE',  ( 1.000000000000000000, -1.331116318405244905E-23, -4.755310728521421461E-16 ) ) ;
#50004=DIRECTION ( 'NONE',  ( 0.000000000000000000, 5.664403186863042467E-17, 1.000000000000000000 ) ) ;
#50009=CARTESIAN_POINT ( 'NONE',  ( 181.0000000000000000, -77.49999999999995737, -115.0000000000001563 ) ) ;
#50013=DIRECTION ( 'NONE',  ( -0.000000000000000000, -1.000000000000000000, -0.000000000000000000 ) ) ;
#50014=EDGE_CURVE ( 'NONE', #12862, #39919, #47104, .T. ) ;
#50018=CARTESIAN_POINT ( 'NONE',  ( 168.9999999999999716, -77.49999999999997158, -340.0000000000001137 ) ) ;
#50019=CARTESIAN_POINT ( 'NONE',  ( 168.9999999999999716, -174.9999999999999716, -356.0000000000001705 ) ) ;
#50024=ORIENTED_EDGE ( 'NONE', *, *, #25353, .F. ) ;
#50028=VECTOR ( 'NONE', #15066, 1000.000000000000000 ) ;
#50030=ADVANCED_FACE ( 'NONE', ( #27659 ), #8419, .F. ) ;
#50031=( NAMED_UNIT ( * ) SI_UNIT ( $, .STERADIAN. ) SOLID_ANGLE_UNIT ( ) );
#50040=VERTEX_POINT ( 'NONE', #8909 ) ;
#50053=CARTESIAN_POINT ( 'NONE',  ( 168.9999999999999716, -79.49999999999997158, -340.0000000000001137 ) ) ;
#50060=EDGE_LOOP ( 'NONE', ( #26695, #29458, #46470, #17046 ) ) ;
#50061=DIRECTION ( 'NONE',  ( 0.000000000000000000, -1.580451535867971417E-48, 1.000000000000000000 ) ) ;
#50068=ORIENTED_EDGE ( 'NONE', *, *, #281, .T. ) ;
#50082=CARTESIAN_POINT ( 'NONE',  ( 181.0000000000000000, -97.49999999999997158, -115.0000000000001563 ) ) ;
#50087=VECTOR ( 'NONE', #46935, 1000.000000000000000 ) ;
#50100=ADVANCED_FACE ( 'NONE', ( #36387 ), #44287, .T. ) ;
#50105=EDGE_CURVE ( 'NONE', #42389, #6937, #34847, .T. ) ;
#50117=VECTOR ( 'NONE', #20985, 1000.000000000000114 ) ;
#50127=CIRCLE ( 'NONE', #1847, 4.000000000000003553 ) ;
#50129=LINE ( 'NONE', #34046, #38497 ) ;
#50131=ORIENTED_EDGE ( 'NONE', *, *, #10006, .F. ) ;
#50143=ORIENTED_EDGE ( 'NONE', *, *, #12710, .T. ) ;
#50146=CIRCLE ( 'NONE', #38756, 4.000000000000003553 ) ;
#50150=CARTESIAN_POINT ( 'NONE',  ( 169.0000000000000000, -9.999999999999953815, -113.0000000000001563 ) ) ;
#50151=ORIENTED_EDGE ( 'NONE', *, *, #11722, .T. ) ;
#50157=CIRCLE ( 'NONE', #17446, 4.000000000000003553 ) ;
#50158=DIRECTION ( 'NONE',  ( 0.000000000000000000, 0.000000000000000000, 1.000000000000000000 ) ) ;
#50160=CARTESIAN_POINT ( 'NONE',  ( 168.9999999999999716, -79.49999999999995737, -115.0000000000001563 ) ) ;
#50161=DIRECTION ( 'NONE',  ( -1.000000000000000000, 0.000000000000000000, -2.958228394578794270E-31 ) ) ;
#50166=( NAMED_UNIT ( * ) PLANE_ANGLE_UNIT ( ) SI_UNIT ( $, .RADIAN. ) );
#50168=EDGE_LOOP ( 'NONE', ( #1191, #20095, #13392, #42331 ) ) ;
#50173=CARTESIAN_POINT ( 'NONE',  ( 358.3431457505075741, -185.0000000000001421, -360.0000000000003411 ) ) ;
#50178=ADVANCED_FACE ( 'NONE', ( #10670 ), #6825, .T. ) ;
#50179=DIRECTION ( 'NONE',  ( -1.586032880504786307E-16, 1.654361225106055350E-24, -1.000000000000000000 ) ) ;
#50180=PLANE ( 'NONE',  #25054 ) ;
#50189=DIRECTION ( 'NONE',  ( 0.000000000000000000, -1.000000000000000000, 0.000000000000000000 ) ) ;
#50190=VECTOR ( 'NONE', #22993, 1000.000000000000000 ) ;
#50207=DIRECTION ( 'NONE',  ( -1.586032880504786307E-16, 1.654361225106055350E-24, -1.000000000000000000 ) ) ;
#50217=EDGE_LOOP ( 'NONE', ( #3243, #41289, #49561, #4848 ) ) ;
#50222=VECTOR ( 'NONE', #16981, 1000.000000000000000 ) ;
#50224=DIRECTION ( 'NONE',  ( 6.203854594147707562E-25, -2.067951531382569187E-25, 1.000000000000000000 ) ) ;
#50226=VECTOR ( 'NONE', #15383, 1000.000000000000000 ) ;
#50231=VECTOR ( 'NONE', #32322, 1000.000000000000000 ) ;
#50232=ADVANCED_FACE ( 'NONE', ( #22473 ), #18858, .T. ) ;
#50234=EDGE_CURVE ( 'NONE', #24618, #22458, #45288, .T. ) ;
#50242=CARTESIAN_POINT ( 'NONE',  ( 166.9999999999999716, -168.9999999999999432, -350.0000000000001705 ) ) ;
#50245=ORIENTED_EDGE ( 'NONE', *, *, #16148, .T. ) ;
#50248=VECTOR ( 'NONE', #48133, 1000.000000000000000 ) ;
#50256=EDGE_LOOP ( 'NONE', ( #35776, #1905, #16341, #38446, #43128, #21559, #16409, #39118 ) ) ;
#50259=FACE_OUTER_BOUND ( 'NONE', #12635, .T. ) ;
#50261=ADVANCED_FACE ( 'NONE', ( #41469 ), #3206, .F. ) ;
#50268=CIRCLE ( 'NONE', #34786, 4.000000000000003553 ) ;
#50273=VERTEX_POINT ( 'NONE', #14518 ) ;
#50285=EDGE_CURVE ( 'NONE', #15830, #17104, #33454, .T. ) ;
#50291=CARTESIAN_POINT ( 'NONE',  ( 350.0000000000000000, 165.0000000000000000, -344.0000000000001705 ) ) ;
#50293=EDGE_LOOP ( 'NONE', ( #45522, #20394, #105, #22495 ) ) ;
#50296=DIRECTION ( 'NONE',  ( -1.000000000000000000, 0.000000000000000000, 0.000000000000000000 ) ) ;
#50304=EDGE_CURVE ( 'NONE', #44732, #2449, #45198, .T. ) ;
#50314=LINE ( 'NONE', #14968, #18214 ) ;
#50321=DIRECTION ( 'NONE',  ( 1.132880637372608740E-16, 4.718402560806925739E-50, 1.000000000000000000 ) ) ;
#50325=ORIENTED_EDGE ( 'NONE', *, *, #46638, .T. ) ;
#50326=ORIENTED_EDGE ( 'NONE', *, *, #43545, .F. ) ;
#50331=CARTESIAN_POINT ( 'NONE',  ( 185.0000000000000000, -256.4999999999999432, -114.9999999999999432 ) ) ;
#50338=PLANE ( 'NONE',  #12709 ) ;
#50340=DIRECTION ( 'NONE',  ( -1.000000000000000000, 0.000000000000000000, 1.860490536778032451E-50 ) ) ;
#50350=EDGE_CURVE ( 'NONE', #20029, #14416, #13425, .T. ) ;
#50355=EDGE_CURVE ( 'NONE', #28730, #43135, #2384, .T. ) ;
#50356=CARTESIAN_POINT ( 'NONE',  ( 181.0000000000000000, -93.49999999999997158, -115.0000000000001563 ) ) ;
#50359=CARTESIAN_POINT ( 'NONE',  ( 181.0000000000000000, -268.4999999999999432, -349.9999999999999432 ) ) ;
#50367=ORIENTED_EDGE ( 'NONE', *, *, #31857, .F. ) ;
#50368=ORIENTED_EDGE ( 'NONE', *, *, #23316, .T. ) ;
#50371=VECTOR ( 'NONE', #41874, 1000.000000000000000 ) ;
#50373=ORIENTED_EDGE ( 'NONE', *, *, #24123, .T. ) ;
#50376=DIRECTION ( 'NONE',  ( -1.586032892321652236E-16, -1.000000000000000000, -2.288264760618012091E-48 ) ) ;
#50377=VECTOR ( 'NONE', #50340, 1000.000000000000000 ) ;
#50385=DIRECTION ( 'NONE',  ( 7.793956916774525800E-48, 0.000000000000000000, 1.000000000000000000 ) ) ;
#50399=EDGE_CURVE ( 'NONE', #8725, #47613, #48535, .T. ) ;
#50401=VERTEX_POINT ( 'NONE', #9585 ) ;
#50407=CARTESIAN_POINT ( 'NONE',  ( 0.000000000000000000, 169.0000000000000000, 339.9999999999997726 ) ) ;
#50409=CARTESIAN_POINT ( 'NONE',  ( 339.9999999999999432, -165.0000000000001137, -106.0000000000001990 ) ) ;
#50412=ADVANCED_FACE ( 'NONE', ( #3816 ), #11269, .T. ) ;
#50413=FACE_OUTER_BOUND ( 'NONE', #4667, .T. ) ;
#50414=CIRCLE ( 'NONE', #10204, 4.000000000000003553 ) ;
#50415=EDGE_CURVE ( 'NONE', #44239, #41902, #38235, .T. ) ;
#50434=ORIENTED_EDGE ( 'NONE', *, *, #36986, .F. ) ;
#50435=ORIENTED_EDGE ( 'NONE', *, *, #12170, .T. ) ;
#50441=DIRECTION ( 'NONE',  ( -1.586032880504786307E-16, 1.654361225106055350E-24, -1.000000000000000000 ) ) ;
#50443=VECTOR ( 'NONE', #47435, 1000.000000000000000 ) ;
#50448=FACE_OUTER_BOUND ( 'NONE', #27185, .T. ) ;
#50453=CARTESIAN_POINT ( 'NONE',  ( 339.9999999999998863, -180.9999999999999716, 341.9999999999997726 ) ) ;
#50459=ORIENTED_EDGE ( 'NONE', *, *, #47704, .F. ) ;
#50465=CARTESIAN_POINT ( 'NONE',  ( 169.0000000000000000, -174.9999999999999716, -95.00000000000014211 ) ) ;
#50472=ORIENTED_EDGE ( 'NONE', *, *, #28126, .T. ) ;
#50476=DIRECTION ( 'NONE',  ( 1.333906992743555050E-23, -1.000000000000000000, 0.000000000000000000 ) ) ;
#50481=DIRECTION ( 'NONE',  ( -1.586032892321652236E-16, -1.000000000000000000, -6.853681917100419162E-49 ) ) ;
#50483=CARTESIAN_POINT ( 'NONE',  ( 181.0000000000000284, -174.9999999999999716, -115.0000000000001563 ) ) ;
#50485=VERTEX_POINT ( 'NONE', #22805 ) ;
#50489=ORIENTED_EDGE ( 'NONE', *, *, #23750, .T. ) ;
#50490=DIRECTION ( 'NONE',  ( -1.000000000000000000, 4.758098676964957447E-16, 1.586032892321651989E-16 ) ) ;
#50491=ORIENTED_EDGE ( 'NONE', *, *, #12166, .F. ) ;
#50499=CARTESIAN_POINT ( 'NONE',  ( 339.9999999999999432, 181.0000000000002274, -356.0000000000003411 ) ) ;
#50502=CARTESIAN_POINT ( 'NONE',  ( 350.0000000000000000, 181.0000000000000284, -356.0000000000002274 ) ) ;
#50503=DIRECTION ( 'NONE',  ( 0.000000000000000000, -2.265761274745217480E-16, 1.000000000000000000 ) ) ;
#50504=ORIENTED_EDGE ( 'NONE', *, *, #46903, .F. ) ;
#50505=CARTESIAN_POINT ( 'NONE',  ( 339.9999999999998863, -174.9999999999999716, 359.9999999999998295 ) ) ;
#50506=DIRECTION ( 'NONE',  ( 0.000000000000000000, 0.000000000000000000, 1.000000000000000000 ) ) ;
#50507=VERTEX_POINT ( 'NONE', #7938 ) ;
#50510=CARTESIAN_POINT ( 'NONE',  ( 350.0000000000001137, 167.0000000000000000, 355.9999999999997726 ) ) ;
#50516=CARTESIAN_POINT ( 'NONE',  ( 342.0000000000000000, -167.8284271247461561, 342.8284271247460424 ) ) ;
#50532=DIRECTION ( 'NONE',  ( 0.000000000000000000, 0.000000000000000000, -1.000000000000000000 ) ) ;
#50534=VERTEX_POINT ( 'NONE', #26663 ) ;
#50540=DIRECTION ( 'NONE',  ( -1.000000000000000000, 0.000000000000000000, -1.612977847700450206E-50 ) ) ;
#50541=ADVANCED_FACE ( 'NONE', ( #27174 ), #42547, .T. ) ;
#50545=DIRECTION ( 'NONE',  ( 0.000000000000000000, 1.000000000000000000, -3.186989995019654210E-49 ) ) ;
#50547=ORIENTED_EDGE ( 'NONE', *, *, #28220, .T. ) ;
#50548=CARTESIAN_POINT ( 'NONE',  ( 181.0000000000000000, -256.4999999999999432, -349.9999999999999432 ) ) ;
#50555=EDGE_CURVE ( 'NONE', #15793, #29971, #13214, .T. ) ;
#50569=ORIENTED_EDGE ( 'NONE', *, *, #26775, .F. ) ;
#50571=DIRECTION ( 'NONE',  ( 1.000000000000000000, 0.000000000000000000, 0.000000000000000000 ) ) ;
#50572=DIRECTION ( 'NONE',  ( 0.000000000000000000, 1.000000000000000000, 0.000000000000000000 ) ) ;
#50575=CARTESIAN_POINT ( 'NONE',  ( 164.9999999999999716, 6.000000000000060396, -340.0000000000001137 ) ) ;
#50579=CARTESIAN_POINT ( 'NONE',  ( 344.0000000000000000, 167.0000000000000000, -342.0000000000001137 ) ) ;
#50583=CIRCLE ( 'NONE', #39190, 2.000000000000001776 ) ;
#50585=VERTEX_POINT ( 'NONE', #1680 ) ;
#50587=DIRECTION ( 'NONE',  ( 0.000000000000000000, -0.7071067811865475727, 0.7071067811865474617 ) ) ;
#50594=ADVANCED_FACE ( 'NONE', ( #39492 ), #12272, .F. ) ;
#50607=DIRECTION ( 'NONE',  ( -1.000000000000000000, 0.000000000000000000, 1.132880637372608740E-16 ) ) ;
#50609=EDGE_CURVE ( 'NONE', #9207, #35315, #17319, .T. ) ;
#50618=ADVANCED_FACE ( 'NONE', ( #43570, #13719 ), #6291, .T. ) ;
#50620=DIRECTION ( 'NONE',  ( 0.000000000000000000, 1.000000000000000000, 0.000000000000000000 ) ) ;
#50622=PLANE ( 'NONE',  #40569 ) ;
#50628=CARTESIAN_POINT ( 'NONE',  ( 168.9999999999999716, -79.49999999999997158, -340.0000000000001137 ) ) ;
#50640=ORIENTED_EDGE ( 'NONE', *, *, #40435, .T. ) ;
#50642=EDGE_CURVE ( 'NONE', #4741, #38121, #32425, .T. ) ;
#50644=DIRECTION ( 'NONE',  ( 1.000000000000000000, 0.000000000000000000, 0.000000000000000000 ) ) ;
#50645=ORIENTED_EDGE ( 'NONE', *, *, #43491, .T. ) ;
#50646=EDGE_LOOP ( 'NONE', ( #665, #43487, #27390, #14001 ) ) ;
#50654=DIRECTION ( 'NONE',  ( -3.172065784643302499E-16, -1.000000000000000000, 2.537652627714642000E-15 ) ) ;
#50656=VERTEX_POINT ( 'NONE', #14214 ) ;
#50666=DIRECTION ( 'NONE',  ( 0.000000000000000000, 0.000000000000000000, -1.000000000000000000 ) ) ;
#50667=CLOSED_SHELL ( 'NONE', ( #12857, #48730, #33141, #49280, #18247, #1447, #20300, #17064, #28644, #25948, #30151, #23822, #42852, #18263, #48042, #20630, #2548, #14861 ) ) ;
#50674=DIRECTION ( 'NONE',  ( 0.000000000000000000, 4.687818848539279227E-49, -1.000000000000000000 ) ) ;
#50676=ADVANCED_FACE ( 'NONE', ( #45995, #41678 ), #33492, .T. ) ;
#50678=ORIENTED_EDGE ( 'NONE', *, *, #22742, .F. ) ;
#50679=DIRECTION ( 'NONE',  ( 0.000000000000000000, 0.000000000000000000, -1.000000000000000000 ) ) ;
#50689=LINE ( 'NONE', #27394, #2910 ) ;
#50694=VECTOR ( 'NONE', #46012, 1000.000000000000000 ) ;
#50696=PLANE ( 'NONE',  #25427 ) ;
#50700=( BOUNDED_CURVE ( )  B_SPLINE_CURVE ( 3, ( #15797, #22479, #19644, #47053 ),
 .UNSPECIFIED., .F., .F. ) 
 B_SPLINE_CURVE_WITH_KNOTS ( ( 4, 4 ),
 ( 1.570796326794903441, 3.141592653589515560 ),
 .UNSPECIFIED. ) 
 CURVE ( )  GEOMETRIC_REPRESENTATION_ITEM ( )  RATIONAL_B_SPLINE_CURVE ( ( 1.000000000000000000, 0.8047378541244319949, 0.8047378541244319949, 1.000000000000000000 ) ) 
 REPRESENTATION_ITEM ( '' )  );
#50701=EDGE_CURVE ( 'NONE', #33352, #23671, #19841, .T. ) ;
#50702=LINE ( 'NONE', #15090, #31708 ) ;
#50706=( NAMED_UNIT ( * ) PLANE_ANGLE_UNIT ( ) SI_UNIT ( $, .RADIAN. ) );
#50710=DIRECTION ( 'NONE',  ( 1.000000000000000000, -4.758098676964956461E-16, -8.975803739141899931E-48 ) ) ;
#50718=VERTEX_POINT ( 'NONE', #43445 ) ;
#50722=CARTESIAN_POINT ( 'NONE',  ( 344.0000000000000000, 183.0000000000000284, 357.9999999999998863 ) ) ;
#50741=COLOUR_RGB('Dark Blue',0.08,0.2,0.34);
#50742=FILL_AREA_STYLE_COLOUR('',#50741);
#50743=FILL_AREA_STYLE('',(#50742));
#50744=SURFACE_STYLE_FILL_AREA(#50743);
#50745=SURFACE_SIDE_STYLE('',(#50744));
#50746=SURFACE_STYLE_USAGE(.BOTH.,#50745);
#50747=PRESENTATION_STYLE_ASSIGNMENT((#50746));
ENDSEC;
END-ISO-10303-21;
